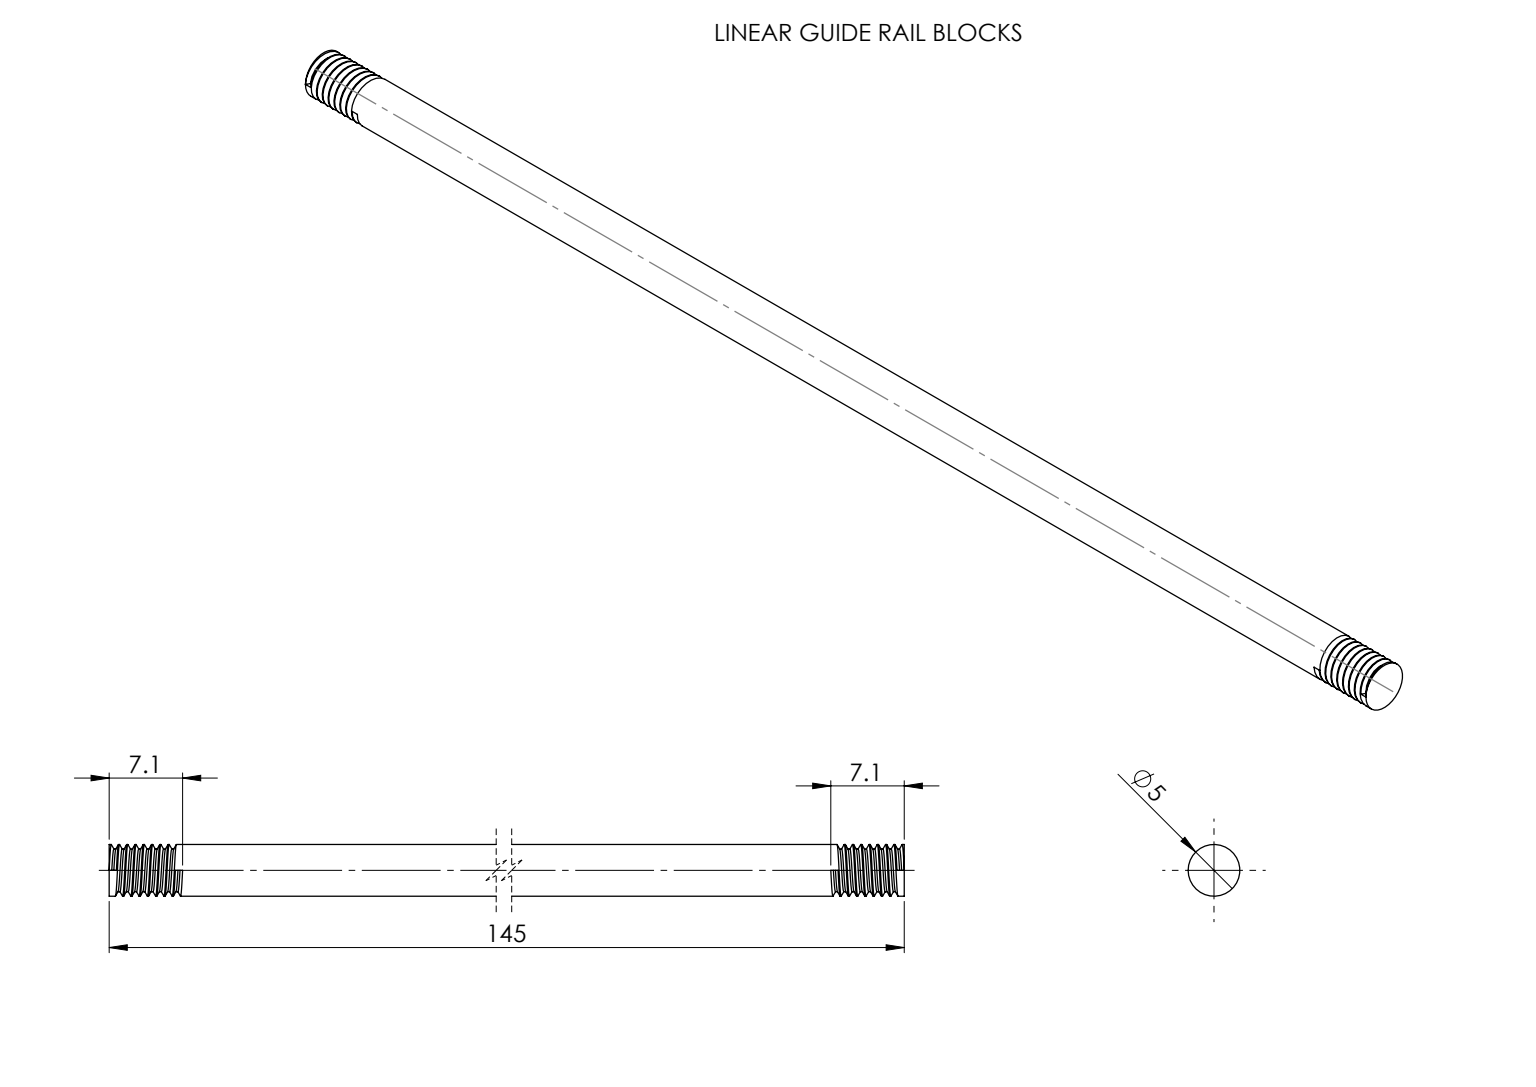
ISO-10303-21;
HEADER;
FILE_DESCRIPTION (('STEP AP214'),
    '1' );
FILE_NAME ('Linear Guide Rail Blocks.step',
    '2026-10-08T13:46:47',
    ( '' ),
    ( '' ),
    'SwSTEP 2.0',
    'SolidWorks 2026',
    '' );
FILE_SCHEMA (( 'AUTOMOTIVE_DESIGN' ));
ENDSEC;

DATA;
#7=AXIS2_PLACEMENT_3D ( 'NONE', #19593, #12332, #12571 ) ;
#8=CARTESIAN_POINT ( 'NONE',  ( -67.64999999999999147, 11.03553390593273598, 17.50000000000000355 ) ) ;
#17=CARTESIAN_POINT ( 'NONE',  ( 65.80000000218494449, 9.999999999999998224, 12.49999999999999289 ) ) ;
#19=CARTESIAN_POINT ( 'NONE',  ( -69.15000000109247935, 8.538419263543524096, 13.53841926354352054 ) ) ;
#22=CARTESIAN_POINT ( 'NONE',  ( -68.25000000109247367, 7.933012699999995476, 14.99999999999999645 ) ) ;
#32=CARTESIAN_POINT ( 'NONE',  ( -70.40000000109250777, 10.85617417291294551, 17.06698729999999742 ) ) ;
#33=CARTESIAN_POINT ( 'NONE',  ( -70.80000000109245661, 7.933012699999995476, 15.85617417291294196 ) ) ;
#43=CARTESIAN_POINT ( 'NONE',  ( 70.34999999999999432, 7.499999999999996447, 13.96446609406725514 ) ) ;
#48=EDGE_CURVE ( 'NONE', #4600, #14452, #12227, .T. ) ;
#57=( BOUNDED_CURVE ( )  B_SPLINE_CURVE ( 2, ( #2610, #2843, #8385, #9828, #929, #6582, #8267, #22849, #6463, #6101, #17122, #17483, #13433, #15701, #13784, #9954, #4303, #22975, #13896, #11639, #18906, #22618, #13542, #6222, #20810, #11753, #17248, #20493, #4334, #741, #505, #18828, #9508, #20729, #17161, #8185, #2415, #386, #851, #13111, #22409, #7826, #15148, #8076, #2169, #17043, #22169, #15387, #5783, #17285, #13469, #19061, #2652, #18588, #20845, #4223, #7945, #20371, #3977, #22286, #6018, #15031, #9746, #619, #18944, #15264, #9995, #7717, #11673, #4452, #2527, #5903, #11314, #13228, #4096, #9867, #13575, #16805, #11436, #18711, #22651, #22534, #2301, #9636, #6257, #16927, #11789, #11559, #13345, #20613, #6145, #10351, #23232, #4923, #21079, #10224, #15739, #2878, #3239, #19639, #8539, #1312, #13695, #13823, #19181, #20955, #6378, #23115, #17398, #12136, #14038, #23010, #4688, #12260, #8652, #1083, #8426, #10464, #2766, #17640, #1430, #6500, #17858, #21428, #22767, #13933, #19527, #15950, #1200 ),
 .UNSPECIFIED., .F., .F. ) 
 B_SPLINE_CURVE_WITH_KNOTS ( ( 3, 2, 2, 2, 2, 2, 2, 2, 2, 2, 2, 2, 2, 2, 2, 2, 2, 2, 2, 2, 2, 2, 2, 2, 2, 2, 2, 2, 2, 2, 2, 2, 2, 2, 2, 2, 2, 2, 2, 2, 2, 2, 2, 2, 2, 2, 2, 2, 2, 2, 2, 2, 2, 2, 2, 2, 2, 2, 2, 2, 2, 2, 2, 2, 3 ),
 ( 0.000000000000000000, 0.01562500000000000000, 0.03125000000000000000, 0.04687500000000000000, 0.06250000000000000000, 0.07812500000000000000, 0.09375000000000000000, 0.1093750000000000000, 0.1250000000000000000, 0.1406250000000000000, 0.1562500000000000000, 0.1718750000000000000, 0.1875000000000000000, 0.2031250000000000000, 0.2187500000000000000, 0.2343750000000000000, 0.2500000000000000000, 0.2656250000000000000, 0.2812500000000000000, 0.2968750000000000000, 0.3125000000000000000, 0.3281250000000000000, 0.3437500000000000000, 0.3593750000000000000, 0.3750000000000000000, 0.3906250000000000000, 0.4062500000000000000, 0.4218750000000000000, 0.4375000000000000000, 0.4531250000000000000, 0.4687500000000000000, 0.4843750000000000000, 0.5000000000000000000, 0.5156250000000000000, 0.5312500000000000000, 0.5468750000000000000, 0.5625000000000000000, 0.5781250000000000000, 0.5937500000000000000, 0.6093750000000000000, 0.6250000000000000000, 0.6406250000000000000, 0.6562500000000000000, 0.6718750000000000000, 0.6875000000000000000, 0.7031250000000000000, 0.7187500000000000000, 0.7343750000000000000, 0.7500000000000000000, 0.7656250000000000000, 0.7812500000000000000, 0.7968750000000000000, 0.8125000000000000000, 0.8281250000000000000, 0.8437500000000000000, 0.8593750000000000000, 0.8750000000000000000, 0.8906250000000000000, 0.9062500000000000000, 0.9218750000000000000, 0.9375000000000000000, 0.9531250000000000000, 0.9687500000000000000, 0.9843750000000000000, 1.000000000000000000 ),
 .UNSPECIFIED. ) 
 CURVE ( )  GEOMETRIC_REPRESENTATION_ITEM ( )  RATIONAL_B_SPLINE_CURVE ( ( 1.000000000000000000, 0.9238795325112867385, 1.000000000000000000, 0.9238795325112867385, 1.000000000000000000, 0.9238795325112867385, 1.000000000000000000, 0.9238795325112867385, 1.000000000000000000, 0.9238795325112867385, 1.000000000000000000, 0.9238795325112867385, 1.000000000000000000, 0.9238795325112867385, 1.000000000000000000, 0.9238795325112867385, 1.000000000000000000, 0.9238795325112867385, 1.000000000000000000, 0.9238795325112867385, 1.000000000000000000, 0.9238795325112867385, 1.000000000000000000, 0.9238795325112867385, 1.000000000000000000, 0.9238795325112867385, 1.000000000000000000, 0.9238795325112867385, 1.000000000000000000, 0.9238795325112867385, 1.000000000000000000, 0.9238795325112867385, 1.000000000000000000, 0.9238795325112867385, 1.000000000000000000, 0.9238795325112867385, 1.000000000000000000, 0.9238795325112867385, 1.000000000000000000, 0.9238795325112867385, 1.000000000000000000, 0.9238795325112867385, 1.000000000000000000, 0.9238795325112867385, 1.000000000000000000, 0.9238795325112867385, 1.000000000000000000, 0.9238795325112867385, 1.000000000000000000, 0.9238795325112867385, 1.000000000000000000, 0.9238795325112867385, 1.000000000000000000, 0.9238795325112867385, 1.000000000000000000, 0.9238795325112867385, 1.000000000000000000, 0.9238795325112867385, 1.000000000000000000, 0.9238795325112867385, 1.000000000000000000, 0.9238795325112867385, 1.000000000000000000, 0.9238795325112867385, 1.000000000000000000, 0.9238795325112867385, 1.000000000000000000, 0.9238795325112867385, 1.000000000000000000, 0.9238795325112867385, 1.000000000000000000, 0.9238795325112867385, 1.000000000000000000, 0.9238795325112867385, 1.000000000000000000, 0.9238795325112867385, 1.000000000000000000, 0.9238795325112867385, 1.000000000000000000, 0.9238795325112867385, 1.000000000000000000, 0.9238795325112867385, 1.000000000000000000, 0.9238795325112867385, 1.000000000000000000, 0.9238795325112867385, 1.000000000000000000, 0.9238795325112867385, 1.000000000000000000, 0.9238795325112867385, 1.000000000000000000, 0.9238795325112867385, 1.000000000000000000, 0.9238795325112867385, 1.000000000000000000, 0.9238795325112867385, 1.000000000000000000, 0.9238795325112867385, 1.000000000000000000, 0.9238795325112867385, 1.000000000000000000, 0.9238795325112867385, 1.000000000000000000, 0.9238795325112867385, 1.000000000000000000, 0.9238795325112867385, 1.000000000000000000, 0.9238795325112867385, 1.000000000000000000, 0.9238795325112867385, 1.000000000000000000, 0.9238795325112867385, 1.000000000000000000, 0.9238795325112867385, 1.000000000000000000, 0.9238795325112867385, 1.000000000000000000, 0.9238795325112867385, 1.000000000000000000, 0.9238795325112867385, 1.000000000000000000, 0.9238795325112867385, 1.000000000000000000, 0.9238795325112867385, 1.000000000000000000, 0.9238795325112867385, 1.000000000000000000, 0.9238795325112867385, 1.000000000000000000 ) ) 
 REPRESENTATION_ITEM ( '' )  );
#59=CARTESIAN_POINT ( 'NONE',  ( 68.14999999999999147, 11.03553390593273598, 12.49999999999999289 ) ) ;
#68=ORIENTED_EDGE ( 'NONE', *, *, #3329, .T. ) ;
#71=CARTESIAN_POINT ( 'NONE',  ( -72.37500000054622262, 9.999999999999998224, 17.28349365000000049 ) ) ;
#81=CARTESIAN_POINT ( 'NONE',  ( 66.15000000218495302, 11.03553390593273598, 17.50000000000000355 ) ) ;
#93=CARTESIAN_POINT ( 'NONE',  ( 72.25000000000000000, 12.50000000000000000, 13.96446609406725692 ) ) ;
#94=LINE ( 'NONE', #22476, #8071 ) ;
#96=DIRECTION ( 'NONE',  ( -1.000000000000000000, -0.000000000000000000, -0.000000000000000000 ) ) ;
#99=( NAMED_UNIT ( * ) PLANE_ANGLE_UNIT ( ) SI_UNIT ( $, .RADIAN. ) );
#105=CARTESIAN_POINT ( 'NONE',  ( 69.74999999999998579, 11.03553390593276262, 12.50000000000001776 ) ) ;
#107=CARTESIAN_POINT ( 'NONE',  ( -65.40000000218495302, 9.999999999999998224, 17.49999999999999645 ) ) ;
#116=CARTESIAN_POINT ( 'NONE',  ( -66.74999999999998579, 12.50000000000000000, 16.03553390593273420 ) ) ;
#117=AXIS2_PLACEMENT_3D ( 'NONE', #18833, #4695, #4456 ) ;
#118=CARTESIAN_POINT ( 'NONE',  ( 66.45000000218495018, 7.499999999999996447, 13.96446609406725514 ) ) ;
#120=CARTESIAN_POINT ( 'NONE',  ( 65.80000000109247082, 7.933012699999995476, 15.85617417291294196 ) ) ;
#127=PRODUCT ( 'Linear Guide Rail Blocks', 'Linear Guide Rail Blocks', '', ( #7707 ) ) ;
#130=CARTESIAN_POINT ( 'NONE',  ( -70.65000000109247935, 7.933012699999995476, 14.99999999999999645 ) ) ;
#133=CARTESIAN_POINT ( 'NONE',  ( -69.95000000109247651, 8.538419263543522320, 16.46158073645647235 ) ) ;
#141=CARTESIAN_POINT ( 'NONE',  ( -70.30000000109248504, 12.06698730000000275, 15.85617417291294196 ) ) ;
#144=CARTESIAN_POINT ( 'NONE',  ( -68.90000000109246514, 12.06698730000000275, 15.85617417291294196 ) ) ;
#170=CARTESIAN_POINT ( 'NONE',  ( 67.99999999999998579, 8.232233047033629347, 13.23223304703362402 ) ) ;
#172=DIRECTION ( 'NONE',  ( 0.000000000000000000, 0.000000000000000000, 1.000000000000000000 ) ) ;
#181=CARTESIAN_POINT ( 'NONE',  ( 68.60000000218495586, 9.999999999999998224, 17.49999999999999645 ) ) ;
#191=( BOUNDED_CURVE ( )  B_SPLINE_CURVE ( 2, ( #20921, #4538, #19693, #10520, #10408, #17688, #1250, #8589, #23173 ),
 .UNSPECIFIED., .F., .F. ) 
 B_SPLINE_CURVE_WITH_KNOTS ( ( 3, 2, 2, 2, 3 ),
 ( 0.3125000000000002776, 0.3281250000000001665, 0.3437500000000001110, 0.3593750000000000000, 0.3749999999999998890 ),
 .UNSPECIFIED. ) 
 CURVE ( )  GEOMETRIC_REPRESENTATION_ITEM ( )  RATIONAL_B_SPLINE_CURVE ( ( 0.9999999999999986677, 0.9238795325112880708, 1.000000000000000000, 0.9238795325112867385, 1.000000000000000000, 0.9238795325112867385, 1.000000000000000000, 0.9238795325112872936, 0.9999999999999994449 ) ) 
 REPRESENTATION_ITEM ( '' )  );
#198=CARTESIAN_POINT ( 'NONE',  ( 70.50000000109247367, 9.143825827087049163, 17.06698729999999742 ) ) ;
#200=CARTESIAN_POINT ( 'NONE',  ( 70.75000000109247367, 8.538419263543522320, 16.46158073645647235 ) ) ;
#206=DIRECTION ( 'NONE',  ( -1.000000000000000000, -0.000000000000000000, -0.000000000000000000 ) ) ;
#218=CARTESIAN_POINT ( 'NONE',  ( 70.54999999999999716, 11.03553390593272177, 12.49999999999998046 ) ) ;
#229=CARTESIAN_POINT ( 'NONE',  ( 71.25000000109247367, 12.06698730000000097, 14.99999999999999645 ) ) ;
#230=ORIENTED_EDGE ( 'NONE', *, *, #2307, .F. ) ;
#231=CARTESIAN_POINT ( 'NONE',  ( -68.54999999999999716, 8.964466094067258695, 17.50000000000000355 ) ) ;
#233=CARTESIAN_POINT ( 'NONE',  ( 66.95000000109246230, 11.46158073645647235, 13.53841926354352232 ) ) ;
#242=CARTESIAN_POINT ( 'NONE',  ( -69.65000000109247935, 9.999999999999998224, 17.06698730000000097 ) ) ;
#245=CARTESIAN_POINT ( 'NONE',  ( -71.80000000109245661, 9.143825827087050939, 12.93301269999999370 ) ) ;
#254=CARTESIAN_POINT ( 'NONE',  ( -70.50000000109247367, 9.143825827087049163, 17.06698729999999742 ) ) ;
#256=CARTESIAN_POINT ( 'NONE',  ( -69.15000000109246514, 8.538419263543522320, 16.46158073645647235 ) ) ;
#258=PLANE ( 'NONE',  #11121 ) ;
#260=CARTESIAN_POINT ( 'NONE',  ( -71.70000000000000284, 9.999999999999998224, 17.49999999999999645 ) ) ;
#283=ADVANCED_FACE ( 'NONE', ( #1848 ), #11347, .T. ) ;
#289=CARTESIAN_POINT ( 'NONE',  ( 69.14999999999999147, 12.50000000000000000, 16.03553390593273420 ) ) ;
#318=CARTESIAN_POINT ( 'NONE',  ( 70.70000000109247651, 7.933012699999995476, 14.14382582708705094 ) ) ;
#319=CARTESIAN_POINT ( 'NONE',  ( 66.49999999999998579, 9.999999999999998224, 12.49999999999999289 ) ) ;
#320=CARTESIAN_POINT ( 'NONE',  ( 71.55000000109245661, 8.538419263543522320, 16.46158073645647235 ) ) ;
#333=CARTESIAN_POINT ( 'NONE',  ( -70.20000000218495018, 9.999999999999998224, 17.49999999999999645 ) ) ;
#337=ORIENTED_EDGE ( 'NONE', *, *, #22086, .T. ) ;
#354=CARTESIAN_POINT ( 'NONE',  ( 69.75000000109245946, 11.46158073645647235, 16.46158073645647235 ) ) ;
#360=CARTESIAN_POINT ( 'NONE',  ( 65.75000000109247367, 8.538419263543522320, 16.46158073645647235 ) ) ;
#366=CARTESIAN_POINT ( 'NONE',  ( -71.30000000218494449, 8.232233047033629347, 13.23223304703362402 ) ) ;
#370=CARTESIAN_POINT ( 'NONE',  ( -68.10000000109248219, 9.143825827087049163, 17.06698730000000097 ) ) ;
#373=CARTESIAN_POINT ( 'NONE',  ( -71.90000000109246514, 10.85617417291294551, 12.93301269999999370 ) ) ;
#384=CARTESIAN_POINT ( 'NONE',  ( -67.50000000109247367, 7.933012699999995476, 14.14382582708705094 ) ) ;
#386=CARTESIAN_POINT ( 'NONE',  ( 70.20000000109246230, 12.06698729999999919, 14.14382582708705094 ) ) ;
#388=CARTESIAN_POINT ( 'NONE',  ( -67.75000000109245946, 8.538419263543524096, 13.53841926354352054 ) ) ;
#399=ORIENTED_EDGE ( 'NONE', *, *, #10605, .F. ) ;
#400=CARTESIAN_POINT ( 'NONE',  ( 70.39999999999999147, 8.232233047033629347, 13.23223304703362402 ) ) ;
#411=DIRECTION ( 'NONE',  ( 0.000000000000000000, 0.000000000000000000, -1.000000000000000000 ) ) ;
#413=CARTESIAN_POINT ( 'NONE',  ( -70.80000000218494449, 12.50000000000000000, 14.99999999999999645 ) ) ;
#417=CARTESIAN_POINT ( 'NONE',  ( 69.49999999999998579, 7.499999999999996447, 14.99999999999999645 ) ) ;
#426=CARTESIAN_POINT ( 'NONE',  ( -71.30000000109247082, 12.06698729999999919, 15.85617417291294196 ) ) ;
#431=CARTESIAN_POINT ( 'NONE',  ( -71.35000000109246798, 8.538419263543522320, 16.46158073645647235 ) ) ;
#433=VERTEX_POINT ( 'NONE', #17433 ) ;
#442=CARTESIAN_POINT ( 'NONE',  ( 71.20000000109246230, 10.85617417291294551, 17.06698729999999742 ) ) ;
#444=CARTESIAN_POINT ( 'NONE',  ( 70.85000000109246798, 7.933012699999995476, 14.99999999999999645 ) ) ;
#445=EDGE_CURVE ( 'NONE', #15027, #12453, #14670, .T. ) ;
#448=CARTESIAN_POINT ( 'NONE',  ( -69.70000000000000284, 9.999999999999998224, 12.49999999999999289 ) ) ;
#456=CARTESIAN_POINT ( 'NONE',  ( -67.00000000109245946, 9.143825827087052716, 12.93301269999999192 ) ) ;
#467=ORIENTED_EDGE ( 'NONE', *, *, #9823, .T. ) ;
#468=CARTESIAN_POINT ( 'NONE',  ( 72.50000000000000000, 9.999999999999998224, 14.99999999999999645 ) ) ;
#474=( NAMED_UNIT ( * ) PLANE_ANGLE_UNIT ( ) SI_UNIT ( $, .RADIAN. ) );
#475=CARTESIAN_POINT ( 'NONE',  ( 70.65000000109246514, 9.999999999999998224, 17.06698730000000097 ) ) ;
#481=CARTESIAN_POINT ( 'NONE',  ( 71.55000000109245661, 8.538419263543522320, 16.46158073645647235 ) ) ;
#489=DIRECTION ( 'NONE',  ( -1.000000000000000000, -0.000000000000000000, -0.000000000000000000 ) ) ;
#494=CARTESIAN_POINT ( 'NONE',  ( -71.70000000109247651, 7.933012699999995476, 14.14382582708705094 ) ) ;
#503=CARTESIAN_POINT ( 'NONE',  ( -66.95000000109246230, 11.46158073645647235, 13.53841926354352232 ) ) ;
#505=CARTESIAN_POINT ( 'NONE',  ( 70.55000000109247082, 8.538419263543522320, 16.46158073645647235 ) ) ;
#506=CARTESIAN_POINT ( 'NONE',  ( -67.35000000109246798, 11.46158073645647235, 16.46158073645647235 ) ) ;
#515=CARTESIAN_POINT ( 'NONE',  ( 72.09999999999999432, 9.999999999999998224, 12.49999999999999289 ) ) ;
#516=EDGE_LOOP ( 'NONE', ( #68, #21518, #3055, #2681, #12780, #20192, #1158, #14031, #18308, #16919, #16791, #2387, #4988, #13331, #13453, #17105, #21865, #10269, #6716 ) ) ;
#528=CARTESIAN_POINT ( 'NONE',  ( -69.50000000218494733, 8.232233047033627571, 16.76776695296636532 ) ) ;
#531=CARTESIAN_POINT ( 'NONE',  ( 68.34999999999999432, 12.50000000000000000, 16.03553390593273420 ) ) ;
#541=( BOUNDED_CURVE ( )  B_SPLINE_CURVE ( 2, ( #16400, #7064, #18073, #8877, #7426, #5378, #16170, #18188, #11021 ),
 .UNSPECIFIED., .F., .F. ) 
 B_SPLINE_CURVE_WITH_KNOTS ( ( 3, 2, 2, 2, 3 ),
 ( 0.4999999999999991118, 0.5156249999999995559, 0.5312500000000000000, 0.5468750000000004441, 0.5625000000000008882 ),
 .UNSPECIFIED. ) 
 CURVE ( )  GEOMETRIC_REPRESENTATION_ITEM ( )  RATIONAL_B_SPLINE_CURVE ( ( 1.000000000000004219, 0.9238795325112824086, 1.000000000000000000, 0.9238795325112867385, 1.000000000000000000, 0.9238795325112867385, 1.000000000000000000, 0.9238795325112824086, 1.000000000000004219 ) ) 
 REPRESENTATION_ITEM ( '' )  );
#543=CARTESIAN_POINT ( 'NONE',  ( -70.85000000109246798, 9.999999999999998224, 12.93301269999999192 ) ) ;
#552=CARTESIAN_POINT ( 'NONE',  ( 66.35000000218495586, 7.499999999999995559, 16.03553390593273420 ) ) ;
#555=CARTESIAN_POINT ( 'NONE',  ( 71.30000000109247082, 12.06698730000000275, 15.85617417291294196 ) ) ;
#588=CARTESIAN_POINT ( 'NONE',  ( 69.45000000109247651, 9.999999999999998224, 12.93301269999999192 ) ) ;
#593=CARTESIAN_POINT ( 'NONE',  ( 72.15000000109246514, 11.46158073645647235, 16.46158073645647235 ) ) ;
#603=CARTESIAN_POINT ( 'NONE',  ( -66.70000000109246230, 7.933012699999995476, 14.14382582708705094 ) ) ;
#606=CARTESIAN_POINT ( 'NONE',  ( -67.85000000109246798, 9.999999999999998224, 12.93301269999999192 ) ) ;
#618=CARTESIAN_POINT ( 'NONE',  ( -67.35000000109248219, 8.538419263543522320, 16.46158073645647235 ) ) ;
#619=CARTESIAN_POINT ( 'NONE',  ( 68.90000000109247935, 9.143825827087049163, 17.06698730000000097 ) ) ;
#620=CARTESIAN_POINT ( 'NONE',  ( -72.29999999999998295, 12.50000000000000000, 14.99999999999999645 ) ) ;
#635=LINE ( 'NONE', #22428, #20559 ) ;
#641=CARTESIAN_POINT ( 'NONE',  ( -71.65000000218496723, 12.50000000000000000, 16.03553390593273420 ) ) ;
#646=CARTESIAN_POINT ( 'NONE',  ( 70.45000000109247651, 9.999999999999998224, 17.06698730000000097 ) ) ;
#647=VECTOR ( 'NONE', #5180, 999.9999999999997726 ) ;
#653=CARTESIAN_POINT ( 'NONE',  ( -71.40000000109246514, 10.85617417291294551, 17.06698730000000097 ) ) ;
#658=CARTESIAN_POINT ( 'NONE',  ( -71.10000000109246798, 12.06698730000000275, 15.85617417291294196 ) ) ;
#667=CARTESIAN_POINT ( 'NONE',  ( 68.15000000109247935, 8.538419263543522320, 16.46158073645647235 ) ) ;
#668=CARTESIAN_POINT ( 'NONE',  ( 69.50000000109247367, 10.85617417291294551, 12.93301269999999370 ) ) ;
#683=VERTEX_POINT ( 'NONE', #3814 ) ;
#686=CARTESIAN_POINT ( 'NONE',  ( -70.54999999999999716, 11.03553390593272177, 12.49999999999998046 ) ) ;
#687=ADVANCED_FACE ( 'NONE', ( #12941 ), #1773, .T. ) ;
#691=CARTESIAN_POINT ( 'NONE',  ( -72.50000000000000000, 9.999999999999998224, 12.49999999999999289 ) ) ;
#704=CARTESIAN_POINT ( 'NONE',  ( 71.50000000109247367, 9.143825827087049163, 17.06698730000000097 ) ) ;
#711=CARTESIAN_POINT ( 'NONE',  ( 70.70000000109247651, 9.143825827087049163, 17.06698729999999742 ) ) ;
#728=CARTESIAN_POINT ( 'NONE',  ( -67.80000000109247082, 9.143825827087050939, 12.93301269999999370 ) ) ;
#735=VERTEX_POINT ( 'NONE', #17959 ) ;
#740=CARTESIAN_POINT ( 'NONE',  ( -68.40000000109249356, 9.143825827087050939, 12.93301269999999370 ) ) ;
#741=CARTESIAN_POINT ( 'NONE',  ( 70.60000000109246798, 7.933012699999995476, 15.85617417291294196 ) ) ;
#742=CARTESIAN_POINT ( 'NONE',  ( -65.90000000109246514, 9.143825827087049163, 17.06698729999999742 ) ) ;
#748=CARTESIAN_POINT ( 'NONE',  ( 72.50000000000000000, 9.999999999999998224, 17.49999999999999645 ) ) ;
#751=CARTESIAN_POINT ( 'NONE',  ( 72.05000000109247082, 9.999999999999998224, 17.06698730000000097 ) ) ;
#768=CARTESIAN_POINT ( 'NONE',  ( -69.20000000218495018, 12.50000000000000000, 14.99999999999999645 ) ) ;
#773=CARTESIAN_POINT ( 'NONE',  ( -71.29999999999998295, 9.999999999999998224, 12.49999999999999289 ) ) ;
#775=CARTESIAN_POINT ( 'NONE',  ( 70.40000000109250777, 10.85617417291294551, 17.06698729999999742 ) ) ;
#776=CARTESIAN_POINT ( 'NONE',  ( 70.70000000218495018, 11.76776695296636888, 13.23223304703362579 ) ) ;
#783=CARTESIAN_POINT ( 'NONE',  ( -68.40000000109246514, 7.933012699999995476, 15.85617417291294196 ) ) ;
#790=CARTESIAN_POINT ( 'NONE',  ( -69.45000000109247651, 12.06698730000000097, 14.99999999999999645 ) ) ;
#793=CARTESIAN_POINT ( 'NONE',  ( 72.50000000000000000, 9.999999999999998224, 12.49999999999999289 ) ) ;
#798=CARTESIAN_POINT ( 'NONE',  ( 68.70000000109246230, 12.06698730000000275, 15.85617417291294196 ) ) ;
#799=CARTESIAN_POINT ( 'NONE',  ( 68.70000000109246230, 10.85617417291294551, 12.93301269999999370 ) ) ;
#807=ORIENTED_EDGE ( 'NONE', *, *, #21186, .F. ) ;
#815=CARTESIAN_POINT ( 'NONE',  ( 71.20000000218495018, 7.499999999999996447, 14.99999999999999645 ) ) ;
#822=CARTESIAN_POINT ( 'NONE',  ( 71.45000000218495018, 11.03553390593273598, 12.49999999999999289 ) ) ;
#826=CARTESIAN_POINT ( 'NONE',  ( 68.30000000109247082, 9.143825827087049163, 17.06698730000000097 ) ) ;
#829=CARTESIAN_POINT ( 'NONE',  ( 70.65000000109246514, 9.999999999999998224, 17.06698730000000097 ) ) ;
#838=CARTESIAN_POINT ( 'NONE',  ( -67.10000000109248219, 12.06698729999999919, 15.85617417291294196 ) ) ;
#840=CARTESIAN_POINT ( 'NONE',  ( -68.10000000109245377, 12.06698730000000275, 15.85617417291294196 ) ) ;
#849=CARTESIAN_POINT ( 'NONE',  ( -68.60000000109248219, 12.06698730000000275, 14.14382582708705094 ) ) ;
#851=CARTESIAN_POINT ( 'NONE',  ( 70.15000000109247935, 11.46158073645647235, 13.53841926354352232 ) ) ;
#853=CARTESIAN_POINT ( 'NONE',  ( -67.95000000109247651, 11.46158073645647235, 13.53841926354352232 ) ) ;
#858=LINE ( 'NONE', #4584, #16612 ) ;
#876=CARTESIAN_POINT ( 'NONE',  ( -71.70000000218495018, 11.76776695296636888, 16.76776695296636532 ) ) ;
#881=CARTESIAN_POINT ( 'NONE',  ( 66.59999999999999432, 11.76776695296636888, 13.23223304703362579 ) ) ;
#882=CARTESIAN_POINT ( 'NONE',  ( 70.75000000109247367, 8.538419263543524096, 13.53841926354352054 ) ) ;
#888=CARTESIAN_POINT ( 'NONE',  ( 67.35000000000000853, 11.03553390593276973, 12.50000000000002665 ) ) ;
#889=CARTESIAN_POINT ( 'NONE',  ( -69.40000000109246514, 9.143825827087052716, 12.93301269999999192 ) ) ;
#905=CARTESIAN_POINT ( 'NONE',  ( 67.75000000109247367, 11.46158073645647235, 13.53841926354352232 ) ) ;
#906=EDGE_CURVE ( 'NONE', #14683, #16067, #1009, .T. ) ;
#907=CARTESIAN_POINT ( 'NONE',  ( 68.45000000109247651, 7.933012699999995476, 14.99999999999999645 ) ) ;
#914=DIRECTION ( 'NONE',  ( -1.000000000000000000, -0.000000000000000000, -0.000000000000000000 ) ) ;
#921=CARTESIAN_POINT ( 'NONE',  ( 69.30000000218494449, 11.76776695296636888, 16.76776695296636532 ) ) ;
#922=CARTESIAN_POINT ( 'NONE',  ( 72.50000000000000000, 9.999999999999998224, 12.49999999999999289 ) ) ;
#923=PRODUCT_DEFINITION_CONTEXT ( 'detailed design', #3030, 'design' ) ;
#928=ORIENTED_EDGE ( 'NONE', *, *, #4298, .F. ) ;
#929=CARTESIAN_POINT ( 'NONE',  ( 71.85000000109246798, 12.06698730000000097, 14.99999999999999645 ) ) ;
#932=CARTESIAN_POINT ( 'NONE',  ( 70.70000000218495018, 11.76776695296636888, 13.23223304703362579 ) ) ;
#935=CARTESIAN_POINT ( 'NONE',  ( 68.10000000109246798, 12.06698729999999919, 15.85617417291294196 ) ) ;
#939=CARTESIAN_POINT ( 'NONE',  ( 70.30000000109248504, 10.85617417291294551, 12.93301269999999370 ) ) ;
#945=LINE ( 'NONE', #1062, #11167 ) ;
#955=CARTESIAN_POINT ( 'NONE',  ( -69.20000000109246230, 7.933012699999995476, 15.85617417291294196 ) ) ;
#967=CARTESIAN_POINT ( 'NONE',  ( -70.95000000000000284, 8.964466094067258695, 17.50000000000000355 ) ) ;
#980=CARTESIAN_POINT ( 'NONE',  ( -71.40000000218495302, 9.999999999999998224, 12.49999999999999289 ) ) ;
#985=EDGE_CURVE ( 'NONE', #683, #21124, #19386, .T. ) ;
#994=CARTESIAN_POINT ( 'NONE',  ( -67.35000000218495586, 8.964466094067258695, 12.49999999999999289 ) ) ;
#997=CARTESIAN_POINT ( 'NONE',  ( 66.40000000000000568, 8.232233047033629347, 13.23223304703362402 ) ) ;
#1000=CARTESIAN_POINT ( 'NONE',  ( 71.20000000109246230, 10.85617417291294551, 17.06698729999999742 ) ) ;
#1008=CARTESIAN_POINT ( 'NONE',  ( -67.55000000109247082, 8.538419263543522320, 16.46158073645647235 ) ) ;
#1009=LINE ( 'NONE', #6420, #5098 ) ;
#1023=CARTESIAN_POINT ( 'NONE',  ( 68.30000000109247082, 7.933012699999995476, 14.14382582708705094 ) ) ;
#1025=CARTESIAN_POINT ( 'NONE',  ( 68.15000000109246514, 11.46158073645647235, 16.46158073645647235 ) ) ;
#1047=CARTESIAN_POINT ( 'NONE',  ( 71.70000000000000284, 9.999999999999998224, 17.49999999999999645 ) ) ;
#1050=CARTESIAN_POINT ( 'NONE',  ( 69.75000000218496155, 8.964466094067258695, 12.49999999999999289 ) ) ;
#1054=CARTESIAN_POINT ( 'NONE',  ( 68.40000000109246514, 7.933012699999995476, 15.85617417291294196 ) ) ;
#1057=LINE ( 'NONE', #8392, #23303 ) ;
#1059=CARTESIAN_POINT ( 'NONE',  ( 69.60000000109248219, 12.06698730000000275, 14.14382582708705094 ) ) ;
#1062=CARTESIAN_POINT ( 'NONE',  ( 72.50000000000000000, 9.999999999999998224, 12.49999999999999289 ) ) ;
#1073=CARTESIAN_POINT ( 'NONE',  ( -68.00000000109245946, 12.06698730000000275, 14.14382582708705094 ) ) ;
#1083=CARTESIAN_POINT ( 'NONE',  ( 66.30000000109247082, 12.06698729999999919, 15.85617417291294196 ) ) ;
#1084=CARTESIAN_POINT ( 'NONE',  ( -70.09999999999999432, 9.999999999999998224, 17.49999999999999645 ) ) ;
#1095=CARTESIAN_POINT ( 'NONE',  ( -71.00000000109248788, 12.06698729999999919, 14.14382582708705094 ) ) ;
#1109=CARTESIAN_POINT ( 'NONE',  ( -66.35000000218495586, 7.499999999999995559, 16.03553390593273420 ) ) ;
#1117=CARTESIAN_POINT ( 'NONE',  ( 68.50000000109247367, 10.85617417291294551, 12.93301269999999370 ) ) ;
#1119=CARTESIAN_POINT ( 'NONE',  ( 70.80000000218494449, 12.50000000000000000, 14.99999999999999645 ) ) ;
#1123=CARTESIAN_POINT ( 'NONE',  ( -69.60000000109246798, 12.06698729999999919, 14.14382582708705094 ) ) ;
#1125=CARTESIAN_POINT ( 'NONE',  ( -69.95000000218493597, 12.50000000000000000, 13.96446609406725692 ) ) ;
#1141=CARTESIAN_POINT ( 'NONE',  ( 66.75000000109247367, 8.538419263543524096, 13.53841926354352054 ) ) ;
#1144=CARTESIAN_POINT ( 'NONE',  ( 68.60000000109246798, 9.143825827087050939, 12.93301269999999370 ) ) ;
#1157=VECTOR ( 'NONE', #6497, 1000.000000000000000 ) ;
#1158=ORIENTED_EDGE ( 'NONE', *, *, #4205, .F. ) ;
#1160=CARTESIAN_POINT ( 'NONE',  ( 71.50000000109248788, 7.933012699999995476, 14.14382582708705094 ) ) ;
#1164=ORIENTED_EDGE ( 'NONE', *, *, #3803, .F. ) ;
#1169=CARTESIAN_POINT ( 'NONE',  ( 71.40000000218495302, 9.999999999999998224, 12.49999999999999289 ) ) ;
#1172=CARTESIAN_POINT ( 'NONE',  ( 67.65000000109247935, 7.933012699999995476, 14.99999999999999645 ) ) ;
#1188=CARTESIAN_POINT ( 'NONE',  ( -72.15000000000001990, 11.03553390593275374, 12.50000000000001243 ) ) ;
#1189=ORIENTED_EDGE ( 'NONE', *, *, #10837, .T. ) ;
#1200=CARTESIAN_POINT ( 'NONE',  ( 65.65000000109247935, 9.999999999999998224, 17.06698730000000097 ) ) ;
#1203=CARTESIAN_POINT ( 'NONE',  ( -69.05000000000002558, 12.50000000000000000, 13.96446609406725869 ) ) ;
#1207=CARTESIAN_POINT ( 'NONE',  ( -67.60000000218495586, 12.50000000000000000, 14.99999999999999645 ) ) ;
#1208=CARTESIAN_POINT ( 'NONE',  ( 72.50000000000000000, 9.999999999999998224, 14.99999999999999645 ) ) ;
#1212=CARTESIAN_POINT ( 'NONE',  ( -71.95000000109247651, 11.46158073645647235, 16.46158073645647235 ) ) ;
#1215=CARTESIAN_POINT ( 'NONE',  ( -70.25000000109247367, 12.06698730000000097, 14.99999999999999645 ) ) ;
#1224=CARTESIAN_POINT ( 'NONE',  ( -65.80000000218494449, 9.999999999999998224, 12.49999999999999289 ) ) ;
#1235=CARTESIAN_POINT ( 'NONE',  ( -67.60000000109246798, 7.933012699999995476, 15.85617417291294196 ) ) ;
#1244=ORIENTED_EDGE ( 'NONE', *, *, #22795, .F. ) ;
#1250=CARTESIAN_POINT ( 'NONE',  ( -69.50000000218494733, 8.232233047033627571, 16.76776695296636532 ) ) ;
#1253=CARTESIAN_POINT ( 'NONE',  ( 71.89999999999999147, 7.499999999999996447, 14.99999999999999645 ) ) ;
#1264=VERTEX_POINT ( 'NONE', #3404 ) ;
#1266=EDGE_CURVE ( 'NONE', #1264, #22517, #13759, .T. ) ;
#1267=CARTESIAN_POINT ( 'NONE',  ( 68.49999999999998579, 9.999999999999998224, 17.49999999999999645 ) ) ;
#1278=CARTESIAN_POINT ( 'NONE',  ( 67.95000000218495018, 7.499999999999995559, 16.03553390593273420 ) ) ;
#1282=CARTESIAN_POINT ( 'NONE',  ( 68.50000000109245946, 7.933012699999995476, 14.14382582708705094 ) ) ;
#1287=CARTESIAN_POINT ( 'NONE',  ( 67.05000000109247082, 9.999999999999998224, 12.93301269999999192 ) ) ;
#1294=EDGE_CURVE ( 'NONE', #4086, #4004, #9769, .T. ) ;
#1296=CARTESIAN_POINT ( 'NONE',  ( 66.74999999999998579, 12.50000000000000000, 16.03553390593273775 ) ) ;
#1301=( BOUNDED_CURVE ( )  B_SPLINE_CURVE ( 2, ( #8573, #11827, #14083, #4487, #6656, #23044, #12176, #888, #15541 ),
 .UNSPECIFIED., .F., .F. ) 
 B_SPLINE_CURVE_WITH_KNOTS ( ( 3, 2, 2, 2, 3 ),
 ( 0.7499999999999997780, 0.7656249999999996669, 0.7812499999999995559, 0.7968749999999994449, 0.8124999999999993339 ),
 .UNSPECIFIED. ) 
 CURVE ( )  GEOMETRIC_REPRESENTATION_ITEM ( )  RATIONAL_B_SPLINE_CURVE ( ( 1.000000000000001110, 0.9238795325112856283, 1.000000000000000000, 0.9238795325112867385, 1.000000000000000000, 0.9238795325112867385, 1.000000000000000000, 0.9238795325112899581, 0.9999999999999967804 ) ) 
 REPRESENTATION_ITEM ( '' )  );
#1311=CARTESIAN_POINT ( 'NONE',  ( -65.85000000109248219, 7.933012699999995476, 14.99999999999999645 ) ) ;
#1312=CARTESIAN_POINT ( 'NONE',  ( 67.00000000109247367, 12.06698729999999919, 14.14382582708705094 ) ) ;
#1315=CARTESIAN_POINT ( 'NONE',  ( -69.34999999999999432, 8.964466094067258695, 17.50000000000000355 ) ) ;
#1316=AXIS2_PLACEMENT_3D ( 'NONE', #8399, #23094, #6705 ) ;
#1329=CARTESIAN_POINT ( 'NONE',  ( -68.40000000109249356, 9.143825827087050939, 12.93301269999999370 ) ) ;
#1340=EDGE_LOOP ( 'NONE', ( #18060, #5958, #5413, #5040 ) ) ;
#1342=CARTESIAN_POINT ( 'NONE',  ( -68.65000000218496723, 8.964466094067258695, 17.50000000000000355 ) ) ;
#1345=CARTESIAN_POINT ( 'NONE',  ( -71.95000000109247651, 11.46158073645647235, 13.53841926354352232 ) ) ;
#1355=CARTESIAN_POINT ( 'NONE',  ( 70.40000000218495302, 7.499999999999996447, 14.99999999999999645 ) ) ;
#1363=LINE ( 'NONE', #18249, #21589 ) ;
#1371=CARTESIAN_POINT ( 'NONE',  ( 66.00000000109247367, 9.143825827087050939, 12.93301269999999370 ) ) ;
#1372=CARTESIAN_POINT ( 'NONE',  ( 71.70000000000000284, 9.999999999999998224, 17.49999999999999645 ) ) ;
#1373=CARTESIAN_POINT ( 'NONE',  ( -65.60000000218495586, 7.499999999999996447, 14.99999999999999645 ) ) ;
#1390=ORIENTED_EDGE ( 'NONE', *, *, #6277, .F. ) ;
#1392=CARTESIAN_POINT ( 'NONE',  ( 68.95000000218495018, 8.964466094067258695, 12.49999999999999289 ) ) ;
#1395=CARTESIAN_POINT ( 'NONE',  ( -68.79999999999999716, 8.232233047033629347, 13.23223304703362402 ) ) ;
#1402=CARTESIAN_POINT ( 'NONE',  ( 68.00000000109245946, 12.06698730000000275, 14.14382582708705094 ) ) ;
#1405=CARTESIAN_POINT ( 'NONE',  ( 72.50000000000000000, 9.999999999999998224, 14.99999999999999645 ) ) ;
#1411=CARTESIAN_POINT ( 'NONE',  ( 66.49999999999998579, 9.999999999999998224, 12.49999999999999289 ) ) ;
#1412=ORIENTED_EDGE ( 'NONE', *, *, #20233, .F. ) ;
#1417=CARTESIAN_POINT ( 'NONE',  ( -66.05000000218494449, 12.50000000000000000, 16.03553390593273775 ) ) ;
#1428=CARTESIAN_POINT ( 'NONE',  ( -65.70000000109249072, 9.143825827087049163, 17.06698729999999742 ) ) ;
#1430=CARTESIAN_POINT ( 'NONE',  ( 66.05000000109247082, 9.999999999999998224, 12.93301269999999192 ) ) ;
#1432=CARTESIAN_POINT ( 'NONE',  ( -71.84999999999999432, 7.499999999999995559, 16.03553390593273420 ) ) ;
#1440=CARTESIAN_POINT ( 'NONE',  ( 67.40000000218495302, 9.999999999999998224, 12.49999999999999289 ) ) ;
#1443=CARTESIAN_POINT ( 'NONE',  ( -66.60000000218495586, 9.999999999999998224, 12.49999999999999289 ) ) ;
#1445=ORIENTED_EDGE ( 'NONE', *, *, #21073, .F. ) ;
#1447=CARTESIAN_POINT ( 'NONE',  ( -71.20000000109246230, 10.85617417291294551, 17.06698730000000097 ) ) ;
#1450=CARTESIAN_POINT ( 'NONE',  ( -68.55000000109247082, 11.46158073645647235, 13.53841926354352232 ) ) ;
#1461=CARTESIAN_POINT ( 'NONE',  ( -68.00000000218494733, 7.499999999999996447, 14.99999999999999645 ) ) ;
#1468=EDGE_CURVE ( 'NONE', #20225, #9434, #3125, .T. ) ;
#1470=CARTESIAN_POINT ( 'NONE',  ( 67.20000000000000284, 8.232233047033629347, 13.23223304703362402 ) ) ;
#1489=( BOUNDED_CURVE ( )  B_SPLINE_CURVE ( 2, ( #9941, #22479, #9817, #5972, #17238, #4406, #20909, #686, #6333 ),
 .UNSPECIFIED., .F., .F. ) 
 B_SPLINE_CURVE_WITH_KNOTS ( ( 3, 2, 2, 2, 3 ),
 ( 0.2500000000000006661, 0.2656250000000005551, 0.2812500000000004441, 0.2968750000000003886, 0.3125000000000002776 ),
 .UNSPECIFIED. ) 
 CURVE ( )  GEOMETRIC_REPRESENTATION_ITEM ( )  RATIONAL_B_SPLINE_CURVE ( ( 0.9999999999999967804, 0.9238795325112899581, 1.000000000000000000, 0.9238795325112867385, 1.000000000000000000, 0.9238795325112867385, 1.000000000000000000, 0.9238795325112854062, 1.000000000000001332 ) ) 
 REPRESENTATION_ITEM ( '' )  );
#1493=ORIENTED_EDGE ( 'NONE', *, *, #3803, .T. ) ;
#1501=CARTESIAN_POINT ( 'NONE',  ( 71.00000000000000000, 8.232233047033627571, 16.76776695296636532 ) ) ;
#1525=CARTESIAN_POINT ( 'NONE',  ( 67.85000000218495586, 8.964466094067258695, 17.50000000000000355 ) ) ;
#1529=ORIENTED_EDGE ( 'NONE', *, *, #19125, .F. ) ;
#1533=CARTESIAN_POINT ( 'NONE',  ( 67.20000000109247651, 12.06698730000000275, 14.14382582708705094 ) ) ;
#1536=CARTESIAN_POINT ( 'NONE',  ( -68.05000000000001137, 8.964466094067256918, 12.49999999999999822 ) ) ;
#1559=CARTESIAN_POINT ( 'NONE',  ( -68.25000000000000000, 12.50000000000000000, 13.96446609406725869 ) ) ;
#1568=ORIENTED_EDGE ( 'NONE', *, *, #14803, .T. ) ;
#1570=CARTESIAN_POINT ( 'NONE',  ( -71.85000000109246798, 12.06698730000000097, 14.99999999999999645 ) ) ;
#1573=CARTESIAN_POINT ( 'NONE',  ( -66.90000000109246514, 10.85617417291294551, 12.93301269999999370 ) ) ;
#1584=CARTESIAN_POINT ( 'NONE',  ( -71.30000000109248504, 9.143825827087049163, 17.06698729999999742 ) ) ;
#1591=CARTESIAN_POINT ( 'NONE',  ( 72.50000000000000000, 9.999999999999998224, 17.49999999999999645 ) ) ;
#1598=CARTESIAN_POINT ( 'NONE',  ( 70.45000000000000284, 8.964466094067244484, 12.50000000000000711 ) ) ;
#1604=DIRECTION ( 'NONE',  ( -1.000000000000000000, -0.000000000000000000, -0.000000000000000000 ) ) ;
#1612=EDGE_CURVE ( 'NONE', #7519, #14091, #3168, .T. ) ;
#1615=CARTESIAN_POINT ( 'NONE',  ( 65.80000000109247082, 7.933012699999995476, 15.85617417291294196 ) ) ;
#1616=CARTESIAN_POINT ( 'NONE',  ( 66.20000000109246230, 9.143825827087050939, 12.93301269999999370 ) ) ;
#1620=CARTESIAN_POINT ( 'NONE',  ( 69.55000000218493028, 7.499999999999996447, 16.03553390593273775 ) ) ;
#1625=CARTESIAN_POINT ( 'NONE',  ( 72.50000000000000000, 9.999999999999998224, 14.99999999999999645 ) ) ;
#1635=EDGE_CURVE ( 'NONE', #7935, #14210, #23634, .T. ) ;
#1643=CARTESIAN_POINT ( 'NONE',  ( 66.55000000218494449, 8.964466094067258695, 12.49999999999999289 ) ) ;
#1651=LINE ( 'NONE', #6817, #13751 ) ;
#1652=CARTESIAN_POINT ( 'NONE',  ( 67.70000000109246230, 7.933012699999995476, 14.14382582708705094 ) ) ;
#1676=CARTESIAN_POINT ( 'NONE',  ( -66.24999999999998579, 7.499999999999995559, 16.03553390593273420 ) ) ;
#1686=CARTESIAN_POINT ( 'NONE',  ( -70.55000000109247082, 8.538419263543522320, 16.46158073645647235 ) ) ;
#1689=CARTESIAN_POINT ( 'NONE',  ( -66.20000000109247651, 12.06698730000000275, 14.14382582708705094 ) ) ;
#1691=CARTESIAN_POINT ( 'NONE',  ( 72.50000000000000000, 9.999999999999998224, 14.99999999999999645 ) ) ;
#1697=CARTESIAN_POINT ( 'NONE',  ( -70.60000000109246798, 7.933012699999995476, 15.85617417291294196 ) ) ;
#1700=CARTESIAN_POINT ( 'NONE',  ( -69.90000000109246514, 9.143825827087049163, 17.06698729999999742 ) ) ;
#1714=VECTOR ( 'NONE', #1604, 1000.000000000000000 ) ;
#1717=VECTOR ( 'NONE', #16961, 999.9999999999997726 ) ;
#1729=CARTESIAN_POINT ( 'NONE',  ( 65.70000000109249072, 9.143825827087049163, 17.06698729999999742 ) ) ;
#1732=CARTESIAN_POINT ( 'NONE',  ( 70.45000000000000284, 8.964466094067258695, 12.49999999999999289 ) ) ;
#1741=FACE_OUTER_BOUND ( 'NONE', #8414, .T. ) ;
#1756=ORIENTED_EDGE ( 'NONE', *, *, #3903, .T. ) ;
#1758=CARTESIAN_POINT ( 'NONE',  ( 69.15000000218495302, 12.50000000000000000, 13.96446609406725869 ) ) ;
#1769=CARTESIAN_POINT ( 'NONE',  ( 72.29999999999998295, 12.50000000000000000, 14.99999999999999645 ) ) ;
#1773=CYLINDRICAL_SURFACE ( 'NONE', #14305, 2.500000000000002220 ) ;
#1792=CARTESIAN_POINT ( 'NONE',  ( -68.39999999999999147, 11.76776695296636888, 16.76776695296636532 ) ) ;
#1802=ORIENTED_EDGE ( 'NONE', *, *, #20831, .F. ) ;
#1804=CARTESIAN_POINT ( 'NONE',  ( -69.70000000109247651, 9.143825827087049163, 17.06698730000000097 ) ) ;
#1807=CARTESIAN_POINT ( 'NONE',  ( -68.90000000109247935, 9.143825827087049163, 17.06698729999999742 ) ) ;
#1815=CARTESIAN_POINT ( 'NONE',  ( -69.40000000109249356, 12.06698730000000275, 14.14382582708705094 ) ) ;
#1817=CARTESIAN_POINT ( 'NONE',  ( -70.15000000109246514, 8.538419263543524096, 13.53841926354352054 ) ) ;
#1821=CARTESIAN_POINT ( 'NONE',  ( 71.89999999999999147, 7.499999999999996447, 14.99999999999999645 ) ) ;
#1829=CARTESIAN_POINT ( 'NONE',  ( -70.14999999999999147, 8.964466094067256918, 17.49999999999999289 ) ) ;
#1846=CARTESIAN_POINT ( 'NONE',  ( 67.79999999999999716, 8.232233047033627571, 16.76776695296636532 ) ) ;
#1848=FACE_OUTER_BOUND ( 'NONE', #12091, .T. ) ;
#1854=CYLINDRICAL_SURFACE ( 'NONE', #2105, 2.500000000000002220 ) ;
#1860=DIRECTION ( 'NONE',  ( -0.000000000000000000, 0.000000000000000000, -1.000000000000000000 ) ) ;
#1870=ORIENTED_EDGE ( 'NONE', *, *, #19457, .F. ) ;
#1874=CARTESIAN_POINT ( 'NONE',  ( 71.60000000109246798, 9.143825827087050939, 12.93301269999999370 ) ) ;
#1885=CARTESIAN_POINT ( 'NONE',  ( 72.50000000000000000, 9.999999999999998224, 14.99999999999999645 ) ) ;
#1888=CARTESIAN_POINT ( 'NONE',  ( -67.74999999999997158, 8.964466094067246260, 17.49999999999999289 ) ) ;
#1896=ORIENTED_EDGE ( 'NONE', *, *, #15551, .T. ) ;
#1904=VERTEX_POINT ( 'NONE', #260 ) ;
#1910=EDGE_CURVE ( 'NONE', #19081, #21422, #12084, .T. ) ;
#1915=CARTESIAN_POINT ( 'NONE',  ( -67.25000000000000000, 8.964466094067258695, 12.49999999999999289 ) ) ;
#1917=CARTESIAN_POINT ( 'NONE',  ( 66.45000000109247651, 9.999999999999998224, 17.06698730000000097 ) ) ;
#1925=CARTESIAN_POINT ( 'NONE',  ( -67.70000000109247651, 10.85617417291294551, 12.93301269999999192 ) ) ;
#1926=ORIENTED_EDGE ( 'NONE', *, *, #9858, .T. ) ;
#1928=CARTESIAN_POINT ( 'NONE',  ( -71.25000000109247367, 12.06698730000000097, 14.99999999999999645 ) ) ;
#1938=CARTESIAN_POINT ( 'NONE',  ( -70.95000000109247651, 11.46158073645647235, 13.53841926354352232 ) ) ;
#1940=CARTESIAN_POINT ( 'NONE',  ( -69.00000000109245946, 10.85617417291294551, 17.06698729999999742 ) ) ;
#1952=ORIENTED_EDGE ( 'NONE', *, *, #11567, .F. ) ;
#1964=CARTESIAN_POINT ( 'NONE',  ( 69.70000000000000284, 9.999999999999998224, 12.49999999999999289 ) ) ;
#1983=EDGE_LOOP ( 'NONE', ( #13921, #10487, #4144, #18954 ) ) ;
#1988=CARTESIAN_POINT ( 'NONE',  ( 70.65000000109247935, 7.933012699999995476, 14.99999999999999645 ) ) ;
#1998=DIRECTION ( 'NONE',  ( 0.000000000000000000, 0.000000000000000000, -1.000000000000000000 ) ) ;
#2008=CARTESIAN_POINT ( 'NONE',  ( 70.89999999999999147, 9.999999999999998224, 17.49999999999999645 ) ) ;
#2019=CARTESIAN_POINT ( 'NONE',  ( 70.50000000109247367, 12.06698729999999919, 15.85617417291294196 ) ) ;
#2027=CARTESIAN_POINT ( 'NONE',  ( 71.70000000109247651, 7.933012699999995476, 14.14382582708705094 ) ) ;
#2035=ADVANCED_FACE ( 'NONE', ( #11563 ), #19293, .F. ) ;
#2038=EDGE_LOOP ( 'NONE', ( #7103, #10512, #10582, #2161 ) ) ;
#2039=CARTESIAN_POINT ( 'NONE',  ( -68.05000000109247082, 9.999999999999998224, 17.06698730000000097 ) ) ;
#2042=CARTESIAN_POINT ( 'NONE',  ( -69.60000000109248219, 12.06698730000000275, 14.14382582708705094 ) ) ;
#2048=CARTESIAN_POINT ( 'NONE',  ( -65.75000000218494733, 8.964466094067258695, 12.49999999999999289 ) ) ;
#2049=CARTESIAN_POINT ( 'NONE',  ( -70.00000000109247367, 7.933012699999995476, 15.85617417291294196 ) ) ;
#2055=EDGE_CURVE ( 'NONE', #23001, #2788, #13699, .T. ) ;
#2064=CARTESIAN_POINT ( 'NONE',  ( -71.45000000218495018, 11.03553390593275374, 12.50000000000001243 ) ) ;
#2074=( BOUNDED_SURFACE ( )  B_SPLINE_SURFACE ( 1, 2, ( 
 ( #21337, #17774, #15764, #12528, #19790, #6530, #1345, #6645, #13849, #13959, #14198, #4833, #12164, #19434, #14559, #9279, #11197, #3862, #7242, #18589, #22170, #23505, #14671, #5658, #9391, #11073, #20256, #7119, #16564, #33, #12872, #9166, #9044, #3733, #14792, #16685, #14432, #22040, #3512, #21823, #10845, #2173, #1817, #12992, #16218, #2049, #21931, #1700, #5426, #21698, #12763, #7590, #18359, #13113, #18471, #7363, #16454, #20127, #16334, #5784, #23629, #5540, #256, #5308, #14911, #1940, #3617, #144, #10957, #12649, #7476, #20372, #3978, #11315, #19909, #20015, #18121, #18234, #15265, #5904, #16928, #7719, #6258, #13696, #2302, #4579, #853, #9996, #11914, #20959, #388, #22289, #18945, #17286, #19182, #9510, #20617, #13578, #506, #9868, #11792, #16807, #11439, #22769, #19063, #15032, #7828, #13229, #20494, #4098, #17163, #18713, #6147, #8077, #9747, #22410, #20846, #2654, #18830, #2416, #4453, #9638, #4336, #15149, #8186, #6019, #13347, #742, #6379 ),
 ( #4224, #15389, #17045, #13470, #620, #11560, #20730, #11675, #15499, #2529, #7947, #22536, #22652, #1432, #6845, #12025, #21548, #19289, #2879, #8654, #17860, #8299, #19403, #17400, #3126, #23366, #12503, #16078, #8540, #22889, #10225, #967, #23235, #6970, #17517, #5160, #8774, #3243, #2767, #14287, #15620, #6503, #12263, #10590, #10109, #13824, #13934, #14169, #1084, #10468, #5045, #21080, #4690, #8427, #12377, #15742, #23011, #6616, #21189, #4805, #17749, #12137, #23118, #1315, #3001, #10352, #21431, #19643, #17641, #1203, #15847, #6731, #21305, #14040, #4927, #19529, #15952, #11045, #16655, #231, #16191, #18443, #1792, #5512, #3362, #1559, #19883, #19990, #12845, #7340, #9256, #8896, #23603, #14645, #18333, #14409, #19760, #8, #14531, #21670, #3486, #21796, #10703, #17982, #9019, #1915, #12966, #18212, #3593, #5279, #16426, #21904, #16540, #20227, #23478, #116, #7090, #18094, #12622, #5758, #5402, #7448, #10821, #5633, #9140, #1676, #16312, #7217, #12740 ) ),
 .UNSPECIFIED., .F., .F., .F. ) 
 B_SPLINE_SURFACE_WITH_KNOTS ( ( 2, 2 ),
 ( 3, 2, 2, 2, 2, 2, 2, 2, 2, 2, 2, 2, 2, 2, 2, 2, 2, 2, 2, 2, 2, 2, 2, 2, 2, 2, 2, 2, 2, 2, 2, 2, 2, 2, 2, 2, 2, 2, 2, 2, 2, 2, 2, 2, 2, 2, 2, 2, 2, 2, 2, 2, 2, 2, 2, 2, 2, 2, 2, 2, 2, 2, 2, 2, 3 ),
 ( 0.000000000000000000, 1.000000000000000000 ),
 ( 0.000000000000000000, 0.01562500000000000000, 0.03125000000000000000, 0.04687500000000000000, 0.06250000000000000000, 0.07812500000000000000, 0.09375000000000000000, 0.1093750000000000000, 0.1250000000000000000, 0.1406250000000000000, 0.1562500000000000000, 0.1718750000000000000, 0.1875000000000000000, 0.2031250000000000000, 0.2187500000000000000, 0.2343750000000000000, 0.2500000000000000000, 0.2656250000000000000, 0.2812500000000000000, 0.2968750000000000000, 0.3125000000000000000, 0.3281250000000000000, 0.3437500000000000000, 0.3593750000000000000, 0.3750000000000000000, 0.3906250000000000000, 0.4062500000000000000, 0.4218750000000000000, 0.4375000000000000000, 0.4531250000000000000, 0.4687500000000000000, 0.4843750000000000000, 0.5000000000000000000, 0.5156250000000000000, 0.5312500000000000000, 0.5468750000000000000, 0.5625000000000000000, 0.5781250000000000000, 0.5937500000000000000, 0.6093750000000000000, 0.6250000000000000000, 0.6406250000000000000, 0.6562500000000000000, 0.6718750000000000000, 0.6875000000000000000, 0.7031250000000000000, 0.7187500000000000000, 0.7343750000000000000, 0.7500000000000000000, 0.7656250000000000000, 0.7812500000000000000, 0.7968750000000000000, 0.8125000000000000000, 0.8281250000000000000, 0.8437500000000000000, 0.8593750000000000000, 0.8750000000000000000, 0.8906250000000000000, 0.9062500000000000000, 0.9218750000000000000, 0.9375000000000000000, 0.9531250000000000000, 0.9687500000000000000, 0.9843750000000000000, 1.000000000000000000 ),
 .UNSPECIFIED. ) 
 GEOMETRIC_REPRESENTATION_ITEM ( )  RATIONAL_B_SPLINE_SURFACE ( (
 ( 1.000000000000000000, 0.9238795325112867385, 1.000000000000000000, 0.9238795325112867385, 1.000000000000000000, 0.9238795325112867385, 1.000000000000000000, 0.9238795325112867385, 1.000000000000000000, 0.9238795325112867385, 1.000000000000000000, 0.9238795325112867385, 1.000000000000000000, 0.9238795325112867385, 1.000000000000000000, 0.9238795325112867385, 1.000000000000000000, 0.9238795325112867385, 1.000000000000000000, 0.9238795325112867385, 1.000000000000000000, 0.9238795325112867385, 1.000000000000000000, 0.9238795325112867385, 1.000000000000000000, 0.9238795325112867385, 1.000000000000000000, 0.9238795325112867385, 1.000000000000000000, 0.9238795325112867385, 1.000000000000000000, 0.9238795325112867385, 1.000000000000000000, 0.9238795325112867385, 1.000000000000000000, 0.9238795325112867385, 1.000000000000000000, 0.9238795325112867385, 1.000000000000000000, 0.9238795325112867385, 1.000000000000000000, 0.9238795325112867385, 1.000000000000000000, 0.9238795325112867385, 1.000000000000000000, 0.9238795325112867385, 1.000000000000000000, 0.9238795325112867385, 1.000000000000000000, 0.9238795325112867385, 1.000000000000000000, 0.9238795325112867385, 1.000000000000000000, 0.9238795325112867385, 1.000000000000000000, 0.9238795325112867385, 1.000000000000000000, 0.9238795325112867385, 1.000000000000000000, 0.9238795325112867385, 1.000000000000000000, 0.9238795325112867385, 1.000000000000000000, 0.9238795325112867385, 1.000000000000000000, 0.9238795325112867385, 1.000000000000000000, 0.9238795325112867385, 1.000000000000000000, 0.9238795325112867385, 1.000000000000000000, 0.9238795325112867385, 1.000000000000000000, 0.9238795325112867385, 1.000000000000000000, 0.9238795325112867385, 1.000000000000000000, 0.9238795325112867385, 1.000000000000000000, 0.9238795325112867385, 1.000000000000000000, 0.9238795325112867385, 1.000000000000000000, 0.9238795325112867385, 1.000000000000000000, 0.9238795325112867385, 1.000000000000000000, 0.9238795325112867385, 1.000000000000000000, 0.9238795325112867385, 1.000000000000000000, 0.9238795325112867385, 1.000000000000000000, 0.9238795325112867385, 1.000000000000000000, 0.9238795325112867385, 1.000000000000000000, 0.9238795325112867385, 1.000000000000000000, 0.9238795325112867385, 1.000000000000000000, 0.9238795325112867385, 1.000000000000000000, 0.9238795325112867385, 1.000000000000000000, 0.9238795325112867385, 1.000000000000000000, 0.9238795325112867385, 1.000000000000000000, 0.9238795325112867385, 1.000000000000000000, 0.9238795325112867385, 1.000000000000000000, 0.9238795325112867385, 1.000000000000000000, 0.9238795325112867385, 1.000000000000000000, 0.9238795325112867385, 1.000000000000000000, 0.9238795325112867385, 1.000000000000000000, 0.9238795325112867385, 1.000000000000000000, 0.9238795325112867385, 1.000000000000000000, 0.9238795325112867385, 1.000000000000000000, 0.9238795325112867385, 1.000000000000000000),
 ( 1.000000000000000000, 0.9238795325112867385, 1.000000000000000000, 0.9238795325112867385, 1.000000000000000000, 0.9238795325112867385, 1.000000000000000000, 0.9238795325112867385, 1.000000000000000000, 0.9238795325112867385, 1.000000000000000000, 0.9238795325112867385, 1.000000000000000000, 0.9238795325112867385, 1.000000000000000000, 0.9238795325112867385, 1.000000000000000000, 0.9238795325112867385, 1.000000000000000000, 0.9238795325112867385, 1.000000000000000000, 0.9238795325112867385, 1.000000000000000000, 0.9238795325112867385, 1.000000000000000000, 0.9238795325112867385, 1.000000000000000000, 0.9238795325112867385, 1.000000000000000000, 0.9238795325112867385, 1.000000000000000000, 0.9238795325112867385, 1.000000000000000000, 0.9238795325112867385, 1.000000000000000000, 0.9238795325112867385, 1.000000000000000000, 0.9238795325112867385, 1.000000000000000000, 0.9238795325112867385, 1.000000000000000000, 0.9238795325112867385, 1.000000000000000000, 0.9238795325112867385, 1.000000000000000000, 0.9238795325112867385, 1.000000000000000000, 0.9238795325112867385, 1.000000000000000000, 0.9238795325112867385, 1.000000000000000000, 0.9238795325112867385, 1.000000000000000000, 0.9238795325112867385, 1.000000000000000000, 0.9238795325112867385, 1.000000000000000000, 0.9238795325112867385, 1.000000000000000000, 0.9238795325112867385, 1.000000000000000000, 0.9238795325112867385, 1.000000000000000000, 0.9238795325112867385, 1.000000000000000000, 0.9238795325112867385, 1.000000000000000000, 0.9238795325112867385, 1.000000000000000000, 0.9238795325112867385, 1.000000000000000000, 0.9238795325112867385, 1.000000000000000000, 0.9238795325112867385, 1.000000000000000000, 0.9238795325112867385, 1.000000000000000000, 0.9238795325112867385, 1.000000000000000000, 0.9238795325112867385, 1.000000000000000000, 0.9238795325112867385, 1.000000000000000000, 0.9238795325112867385, 1.000000000000000000, 0.9238795325112867385, 1.000000000000000000, 0.9238795325112867385, 1.000000000000000000, 0.9238795325112867385, 1.000000000000000000, 0.9238795325112867385, 1.000000000000000000, 0.9238795325112867385, 1.000000000000000000, 0.9238795325112867385, 1.000000000000000000, 0.9238795325112867385, 1.000000000000000000, 0.9238795325112867385, 1.000000000000000000, 0.9238795325112867385, 1.000000000000000000, 0.9238795325112867385, 1.000000000000000000, 0.9238795325112867385, 1.000000000000000000, 0.9238795325112867385, 1.000000000000000000, 0.9238795325112867385, 1.000000000000000000, 0.9238795325112867385, 1.000000000000000000, 0.9238795325112867385, 1.000000000000000000, 0.9238795325112867385, 1.000000000000000000, 0.9238795325112867385, 1.000000000000000000, 0.9238795325112867385, 1.000000000000000000, 0.9238795325112867385, 1.000000000000000000, 0.9238795325112867385, 1.000000000000000000, 0.9238795325112867385, 1.000000000000000000, 0.9238795325112867385, 1.000000000000000000) ) ) 
 REPRESENTATION_ITEM ( '' )  SURFACE ( )  );
#2079=CARTESIAN_POINT ( 'NONE',  ( 68.70000000000000284, 7.499999999999996447, 14.99999999999999645 ) ) ;
#2082=AXIS2_PLACEMENT_3D ( 'NONE', #15831, #16178, #3114 ) ;
#2090=CARTESIAN_POINT ( 'NONE',  ( -70.90000000109246514, 7.933012699999995476, 14.14382582708705094 ) ) ;
#2095=CARTESIAN_POINT ( 'NONE',  ( 71.92500000163870766, 9.999999999999998224, 17.28349365000000049 ) ) ;
#2105=AXIS2_PLACEMENT_3D ( 'NONE', #1625, #11114, #16144 ) ;
#2106=CARTESIAN_POINT ( 'NONE',  ( 70.10000000109246798, 10.85617417291294551, 12.93301269999999370 ) ) ;
#2107=DIRECTION ( 'NONE',  ( 1.000000000000000000, 0.000000000000000000, 0.000000000000000000 ) ) ;
#2108=CARTESIAN_POINT ( 'NONE',  ( 70.40000000109247935, 12.06698730000000275, 14.14382582708705094 ) ) ;
#2118=CARTESIAN_POINT ( 'NONE',  ( -67.50000000109245946, 9.143825827087049163, 17.06698730000000097 ) ) ;
#2125=SURFACE_SIDE_STYLE ('',( #9118 ) ) ;
#2132=CARTESIAN_POINT ( 'NONE',  ( -69.80000000218494449, 9.999999999999998224, 12.49999999999999289 ) ) ;
#2133=ORIENTED_EDGE ( 'NONE', *, *, #21624, .F. ) ;
#2140=CARTESIAN_POINT ( 'NONE',  ( 71.70000000109247651, 7.933012699999995476, 14.14382582708705094 ) ) ;
#2145=CARTESIAN_POINT ( 'NONE',  ( 66.50000000109247367, 9.143825827087049163, 17.06698729999999742 ) ) ;
#2154=CARTESIAN_POINT ( 'NONE',  ( -68.45000000109247651, 9.999999999999998224, 12.93301269999999192 ) ) ;
#2157=CARTESIAN_POINT ( 'NONE',  ( -69.90000000109246514, 9.143825827087049163, 17.06698729999999742 ) ) ;
#2161=ORIENTED_EDGE ( 'NONE', *, *, #22966, .F. ) ;
#2164=ORIENTED_EDGE ( 'NONE', *, *, #19940, .F. ) ;
#2168=CARTESIAN_POINT ( 'NONE',  ( -69.00000000109247367, 7.933012699999995476, 15.85617417291294196 ) ) ;
#2169=CARTESIAN_POINT ( 'NONE',  ( 69.85000000109248219, 7.933012699999995476, 14.99999999999999645 ) ) ;
#2173=CARTESIAN_POINT ( 'NONE',  ( -70.20000000109246230, 9.143825827087050939, 12.93301269999999370 ) ) ;
#2177=CARTESIAN_POINT ( 'NONE',  ( 71.75000000000001421, 8.964466094067221391, 17.49999999999996447 ) ) ;
#2178=STYLED_ITEM ( 'NONE', ( #3945 ), #13661 ) ;
#2185=ORIENTED_EDGE ( 'NONE', *, *, #9823, .F. ) ;
#2187=CARTESIAN_POINT ( 'NONE',  ( -70.09999999999999432, 9.999999999999998224, 17.49999999999999645 ) ) ;
#2192=EDGE_CURVE ( 'NONE', #3210, #6908, #15443, .T. ) ;
#2205=CARTESIAN_POINT ( 'NONE',  ( 67.25000000000000000, 8.964466094067258695, 12.49999999999999289 ) ) ;
#2216=( BOUNDED_CURVE ( )  B_SPLINE_CURVE ( 2, ( #21610, #8712, #10769, #18043, #10986, #1620, #12686, #19941, #3182 ),
 .UNSPECIFIED., .F., .T. ) 
 B_SPLINE_CURVE_WITH_KNOTS ( ( 3, 2, 2, 2, 3 ),
 ( 0.3125000000000002776, 0.3281250000000001665, 0.3437500000000001110, 0.3593750000000000000, 0.3749999999999998890 ),
 .UNSPECIFIED. ) 
 CURVE ( )  GEOMETRIC_REPRESENTATION_ITEM ( )  RATIONAL_B_SPLINE_CURVE ( ( 0.9999999999999986677, 0.9238795325112880708, 1.000000000000000000, 0.9238795325112867385, 1.000000000000000000, 0.9238795325112867385, 1.000000000000000000, 0.9238795325112872936, 0.9999999999999994449 ) ) 
 REPRESENTATION_ITEM ( '' )  );
#2218=CARTESIAN_POINT ( 'NONE',  ( -71.30000000109248504, 9.143825827087049163, 17.06698729999999742 ) ) ;
#2230=CARTESIAN_POINT ( 'NONE',  ( 66.25000000218494733, 8.964466094067258695, 17.50000000000000355 ) ) ;
#2232=VECTOR ( 'NONE', #16777, 1000.000000000000000 ) ;
#2233=CARTESIAN_POINT ( 'NONE',  ( 66.40000000000000568, 8.232233047033629347, 13.23223304703362402 ) ) ;
#2234=CARTESIAN_POINT ( 'NONE',  ( 71.40000000109246514, 10.85617417291294551, 17.06698729999999742 ) ) ;
#2251=CARTESIAN_POINT ( 'NONE',  ( 69.25000000218494733, 12.50000000000000000, 16.03553390593273775 ) ) ;
#2256=CARTESIAN_POINT ( 'NONE',  ( 72.50000000000000000, 9.999999999999998224, 12.49999999999999289 ) ) ;
#2267=CARTESIAN_POINT ( 'NONE',  ( 71.15000000109246514, 11.46158073645647235, 13.53841926354352232 ) ) ;
#2274=CARTESIAN_POINT ( 'NONE',  ( 66.85000000109248219, 9.999999999999998224, 12.93301269999999192 ) ) ;
#2285=CARTESIAN_POINT ( 'NONE',  ( -66.75000000109247367, 8.538419263543524096, 13.53841926354352054 ) ) ;
#2288=CARTESIAN_POINT ( 'NONE',  ( -72.00000000109245946, 12.06698730000000275, 14.14382582708705094 ) ) ;
#2299=CARTESIAN_POINT ( 'NONE',  ( -66.65000000109247935, 7.933012699999995476, 14.99999999999999645 ) ) ;
#2301=CARTESIAN_POINT ( 'NONE',  ( 67.95000000109247651, 11.46158073645647235, 16.46158073645647235 ) ) ;
#2302=CARTESIAN_POINT ( 'NONE',  ( -68.05000000109247082, 12.06698730000000097, 14.99999999999999645 ) ) ;
#2307=EDGE_CURVE ( 'NONE', #16726, #19572, #20022, .T. ) ;
#2326=CARTESIAN_POINT ( 'NONE',  ( -70.75000000218496155, 12.50000000000000000, 13.96446609406725869 ) ) ;
#2330=CARTESIAN_POINT ( 'NONE',  ( 69.64999999999999147, 8.964466094067258695, 12.49999999999999289 ) ) ;
#2338=CARTESIAN_POINT ( 'NONE',  ( -72.25000000109247367, 9.999999999999998224, 17.06698730000000097 ) ) ;
#2339=CARTESIAN_POINT ( 'NONE',  ( -69.84999999999999432, 12.50000000000000000, 13.96446609406725692 ) ) ;
#2343=CARTESIAN_POINT ( 'NONE',  ( -71.40000000109249356, 7.933012699999995476, 15.85617417291294196 ) ) ;
#2352=UNCERTAINTY_MEASURE_WITH_UNIT (LENGTH_MEASURE( 1.000000000000000082E-05 ), #20701, 'distance_accuracy_value', 'NONE');
#2353=CARTESIAN_POINT ( 'NONE',  ( 71.95000000109247651, 11.46158073645647235, 16.46158073645647235 ) ) ;
#2355=CARTESIAN_POINT ( 'NONE',  ( 71.50000000109247367, 9.143825827087049163, 17.06698729999999742 ) ) ;
#2361=CARTESIAN_POINT ( 'NONE',  ( 71.75000000218496155, 11.03553390593273953, 17.50000000000000355 ) ) ;
#2364=CARTESIAN_POINT ( 'NONE',  ( -67.20000000109246230, 12.06698729999999919, 14.14382582708705094 ) ) ;
#2386=CARTESIAN_POINT ( 'NONE',  ( 71.20000000109246230, 12.06698729999999919, 14.14382582708705094 ) ) ;
#2387=ORIENTED_EDGE ( 'NONE', *, *, #22388, .F. ) ;
#2390=CARTESIAN_POINT ( 'NONE',  ( 67.35000000109248219, 8.538419263543522320, 16.46158073645647235 ) ) ;
#2404=CARTESIAN_POINT ( 'NONE',  ( -70.95000000109247651, 8.538419263543524096, 13.53841926354352054 ) ) ;
#2413=CARTESIAN_POINT ( 'NONE',  ( -67.20000000109247651, 10.85617417291294551, 17.06698729999999742 ) ) ;
#2415=CARTESIAN_POINT ( 'NONE',  ( 70.25000000109247367, 12.06698730000000097, 14.99999999999999645 ) ) ;
#2416=CARTESIAN_POINT ( 'NONE',  ( -66.30000000109247082, 10.85617417291294551, 12.93301269999999370 ) ) ;
#2423=CARTESIAN_POINT ( 'NONE',  ( 68.70000000000000284, 7.499999999999996447, 14.99999999999999645 ) ) ;
#2435=ORIENTED_EDGE ( 'NONE', *, *, #3000, .T. ) ;
#2437=CARTESIAN_POINT ( 'NONE',  ( -70.40000000218495302, 7.499999999999996447, 14.99999999999999645 ) ) ;
#2440=CARTESIAN_POINT ( 'NONE',  ( 66.79999999999999716, 11.76776695296636888, 16.76776695296636532 ) ) ;
#2443=CARTESIAN_POINT ( 'NONE',  ( 70.65000000109247935, 7.933012699999995476, 14.99999999999999645 ) ) ;
#2449=CARTESIAN_POINT ( 'NONE',  ( -71.35000000109246798, 11.46158073645647235, 16.46158073645647235 ) ) ;
#2454=CARTESIAN_POINT ( 'NONE',  ( -71.60000000109246798, 9.143825827087050939, 12.93301269999999370 ) ) ;
#2463=CARTESIAN_POINT ( 'NONE',  ( 68.75000000109247367, 11.46158073645647235, 16.46158073645647235 ) ) ;
#2466=CARTESIAN_POINT ( 'NONE',  ( 71.20000000109246230, 12.06698730000000275, 14.14382582708705094 ) ) ;
#2476=CARTESIAN_POINT ( 'NONE',  ( -67.10000000109246798, 10.85617417291294551, 12.93301269999999192 ) ) ;
#2478=DIRECTION ( 'NONE',  ( 0.000000000000000000, 0.000000000000000000, 1.000000000000000000 ) ) ;
#2482=ORIENTED_EDGE ( 'NONE', *, *, #16675, .T. ) ;
#2497=( BOUNDED_CURVE ( )  B_SPLINE_CURVE ( 2, ( #9362, #16775, #17128, #4189, #22625, #15231, #9608, #11401, #22376, #11279, #8040, #2140, #7799, #2499, #7560, #704, #18681, #13195, #11532, #20460, #229, #2386, #2267, #15356, #6228, #13548, #22258, #7913, #4308, #5754, #16900, #9835, #475, #18803, #9715, #2019, #5987, #4068, #3946, #9475, #15117, #22499, #20816, #14882, #13313, #16651, #17012, #4423, #11759, #20340, #354, #7688, #22137, #13085, #18555, #20583, #588, #6108, #13440, #15006, #20702, #11646, #18911, #5871, #17367, #2617, #10079, #10438, #21160, #15924, #8513, #2849, #4659, #15706, #4545, #1282, #19149, #1054, #19499, #826, #17720, #6586, #8390, #935, #13791, #23087, #19372, #19261, #8619, #23201, #6814, #15589, #1172, #21272, #22739, #10198, #3096, #17487, #4774, #12110, #19029, #14135, #21401, #5018, #9960, #17255, #8158, #2966, #15468, #6350, #13664, #6469, #6698, #8273, #10319, #4895, #20925, #11880, #2738, #12231, #22855, #21047, #22981, #11994, #17607, #14013, #13901, #15815, #14258 ),
 .UNSPECIFIED., .F., .F. ) 
 B_SPLINE_CURVE_WITH_KNOTS ( ( 3, 2, 2, 2, 2, 2, 2, 2, 2, 2, 2, 2, 2, 2, 2, 2, 2, 2, 2, 2, 2, 2, 2, 2, 2, 2, 2, 2, 2, 2, 2, 2, 2, 2, 2, 2, 2, 2, 2, 2, 2, 2, 2, 2, 2, 2, 2, 2, 2, 2, 2, 2, 2, 2, 2, 2, 2, 2, 2, 2, 2, 2, 2, 2, 3 ),
 ( 0.000000000000000000, 0.01562500000000000000, 0.03125000000000000000, 0.04687500000000000000, 0.06250000000000000000, 0.07812500000000000000, 0.09375000000000000000, 0.1093750000000000000, 0.1250000000000000000, 0.1406250000000000000, 0.1562500000000000000, 0.1718750000000000000, 0.1875000000000000000, 0.2031250000000000000, 0.2187500000000000000, 0.2343750000000000000, 0.2500000000000000000, 0.2656250000000000000, 0.2812500000000000000, 0.2968750000000000000, 0.3125000000000000000, 0.3281250000000000000, 0.3437500000000000000, 0.3593750000000000000, 0.3750000000000000000, 0.3906250000000000000, 0.4062500000000000000, 0.4218750000000000000, 0.4375000000000000000, 0.4531250000000000000, 0.4687500000000000000, 0.4843750000000000000, 0.5000000000000000000, 0.5156250000000000000, 0.5312500000000000000, 0.5468750000000000000, 0.5625000000000000000, 0.5781250000000000000, 0.5937500000000000000, 0.6093750000000000000, 0.6250000000000000000, 0.6406250000000000000, 0.6562500000000000000, 0.6718750000000000000, 0.6875000000000000000, 0.7031250000000000000, 0.7187500000000000000, 0.7343750000000000000, 0.7500000000000000000, 0.7656250000000000000, 0.7812500000000000000, 0.7968750000000000000, 0.8125000000000000000, 0.8281250000000000000, 0.8437500000000000000, 0.8593750000000000000, 0.8750000000000000000, 0.8906250000000000000, 0.9062500000000000000, 0.9218750000000000000, 0.9375000000000000000, 0.9531250000000000000, 0.9687500000000000000, 0.9843750000000000000, 1.000000000000000000 ),
 .UNSPECIFIED. ) 
 CURVE ( )  GEOMETRIC_REPRESENTATION_ITEM ( )  RATIONAL_B_SPLINE_CURVE ( ( 1.000000000000000000, 0.9238795325112867385, 1.000000000000000000, 0.9238795325112867385, 1.000000000000000000, 0.9238795325112867385, 1.000000000000000000, 0.9238795325112867385, 1.000000000000000000, 0.9238795325112867385, 1.000000000000000000, 0.9238795325112867385, 1.000000000000000000, 0.9238795325112867385, 1.000000000000000000, 0.9238795325112867385, 1.000000000000000000, 0.9238795325112867385, 1.000000000000000000, 0.9238795325112867385, 1.000000000000000000, 0.9238795325112867385, 1.000000000000000000, 0.9238795325112867385, 1.000000000000000000, 0.9238795325112867385, 1.000000000000000000, 0.9238795325112867385, 1.000000000000000000, 0.9238795325112867385, 1.000000000000000000, 0.9238795325112867385, 1.000000000000000000, 0.9238795325112867385, 1.000000000000000000, 0.9238795325112867385, 1.000000000000000000, 0.9238795325112867385, 1.000000000000000000, 0.9238795325112867385, 1.000000000000000000, 0.9238795325112867385, 1.000000000000000000, 0.9238795325112867385, 1.000000000000000000, 0.9238795325112867385, 1.000000000000000000, 0.9238795325112867385, 1.000000000000000000, 0.9238795325112867385, 1.000000000000000000, 0.9238795325112867385, 1.000000000000000000, 0.9238795325112867385, 1.000000000000000000, 0.9238795325112867385, 1.000000000000000000, 0.9238795325112867385, 1.000000000000000000, 0.9238795325112867385, 1.000000000000000000, 0.9238795325112867385, 1.000000000000000000, 0.9238795325112867385, 1.000000000000000000, 0.9238795325112867385, 1.000000000000000000, 0.9238795325112867385, 1.000000000000000000, 0.9238795325112867385, 1.000000000000000000, 0.9238795325112867385, 1.000000000000000000, 0.9238795325112867385, 1.000000000000000000, 0.9238795325112867385, 1.000000000000000000, 0.9238795325112867385, 1.000000000000000000, 0.9238795325112867385, 1.000000000000000000, 0.9238795325112867385, 1.000000000000000000, 0.9238795325112867385, 1.000000000000000000, 0.9238795325112867385, 1.000000000000000000, 0.9238795325112867385, 1.000000000000000000, 0.9238795325112867385, 1.000000000000000000, 0.9238795325112867385, 1.000000000000000000, 0.9238795325112867385, 1.000000000000000000, 0.9238795325112867385, 1.000000000000000000, 0.9238795325112867385, 1.000000000000000000, 0.9238795325112867385, 1.000000000000000000, 0.9238795325112867385, 1.000000000000000000, 0.9238795325112867385, 1.000000000000000000, 0.9238795325112867385, 1.000000000000000000, 0.9238795325112867385, 1.000000000000000000, 0.9238795325112867385, 1.000000000000000000, 0.9238795325112867385, 1.000000000000000000, 0.9238795325112867385, 1.000000000000000000, 0.9238795325112867385, 1.000000000000000000, 0.9238795325112867385, 1.000000000000000000, 0.9238795325112867385, 1.000000000000000000, 0.9238795325112867385, 1.000000000000000000, 0.9238795325112867385, 1.000000000000000000, 0.9238795325112867385, 1.000000000000000000, 0.9238795325112867385, 1.000000000000000000 ) ) 
 REPRESENTATION_ITEM ( '' )  );
#2499=CARTESIAN_POINT ( 'NONE',  ( 71.60000000109246798, 7.933012699999995476, 15.85617417291294196 ) ) ;
#2505=CARTESIAN_POINT ( 'NONE',  ( 68.90000000109246514, 12.06698730000000275, 15.85617417291294196 ) ) ;
#2509=ORIENTED_EDGE ( 'NONE', *, *, #21073, .T. ) ;
#2519=CARTESIAN_POINT ( 'NONE',  ( -68.30000000109247082, 9.143825827087049163, 17.06698729999999742 ) ) ;
#2526=CARTESIAN_POINT ( 'NONE',  ( -68.95000000109247651, 8.538419263543522320, 16.46158073645647235 ) ) ;
#2527=CARTESIAN_POINT ( 'NONE',  ( 68.55000000109247082, 11.46158073645647235, 13.53841926354352232 ) ) ;
#2529=CARTESIAN_POINT ( 'NONE',  ( -72.05000000000001137, 8.964466094067258695, 12.49999999999999289 ) ) ;
#2543=EDGE_LOOP ( 'NONE', ( #16291, #1568, #17086, #21048 ) ) ;
#2549=CARTESIAN_POINT ( 'NONE',  ( -71.60000000218494165, 12.50000000000000000, 14.99999999999999645 ) ) ;
#2552=CARTESIAN_POINT ( 'NONE',  ( -70.95000000000000284, 8.964466094067294222, 17.50000000000003908 ) ) ;
#2554=CARTESIAN_POINT ( 'NONE',  ( 68.95000000109247651, 8.538419263543522320, 16.46158073645647235 ) ) ;
#2561=CARTESIAN_POINT ( 'NONE',  ( -71.90000000109246514, 10.85617417291294551, 12.93301269999999192 ) ) ;
#2565=ORIENTED_EDGE ( 'NONE', *, *, #23408, .T. ) ;
#2568=FACE_OUTER_BOUND ( 'NONE', #18804, .T. ) ;
#2574=EDGE_CURVE ( 'NONE', #14091, #14025, #23666, .T. ) ;
#2581=CARTESIAN_POINT ( 'NONE',  ( 68.10000000109246798, 9.143825827087049163, 17.06698729999999742 ) ) ;
#2583=CARTESIAN_POINT ( 'NONE',  ( 67.20000000109247651, 12.06698730000000275, 14.14382582708705094 ) ) ;
#2589=CARTESIAN_POINT ( 'NONE',  ( 66.80000000218494449, 12.50000000000000000, 14.99999999999999645 ) ) ;
#2593=AXIS2_PLACEMENT_3D ( 'NONE', #10126, #6394, #21449 ) ;
#2600=ORIENTED_EDGE ( 'NONE', *, *, #14803, .F. ) ;
#2601=CARTESIAN_POINT ( 'NONE',  ( -66.20000000218495018, 9.999999999999998224, 17.49999999999999645 ) ) ;
#2605=CARTESIAN_POINT ( 'NONE',  ( -70.60000000218494165, 9.999999999999998224, 12.49999999999999289 ) ) ;
#2610=CARTESIAN_POINT ( 'NONE',  ( 72.05000000109247082, 9.999999999999998224, 17.06698730000000097 ) ) ;
#2612=CARTESIAN_POINT ( 'NONE',  ( 71.60000000218494165, 12.50000000000000000, 14.99999999999999645 ) ) ;
#2615=AXIS2_PLACEMENT_3D ( 'NONE', #468, #11525, #4301 ) ;
#2617=CARTESIAN_POINT ( 'NONE',  ( 69.00000000109245946, 10.85617417291294551, 17.06698730000000097 ) ) ;
#2619=CARTESIAN_POINT ( 'NONE',  ( 72.50000000000000000, 9.999999999999998224, 12.49999999999999289 ) ) ;
#2623=CARTESIAN_POINT ( 'NONE',  ( 70.80000000109245661, 7.933012699999995476, 15.85617417291294196 ) ) ;
#2636=CARTESIAN_POINT ( 'NONE',  ( -65.80000000109247082, 7.933012699999995476, 15.85617417291294196 ) ) ;
#2638=CARTESIAN_POINT ( 'NONE',  ( -67.05000000109247082, 9.999999999999998224, 12.93301269999999192 ) ) ;
#2642=CARTESIAN_POINT ( 'NONE',  ( 65.97500000054623115, 9.999999999999998224, 17.28349365000000049 ) ) ;
#2651=CARTESIAN_POINT ( 'NONE',  ( -66.15000000109247935, 11.46158073645647235, 13.53841926354352232 ) ) ;
#2652=CARTESIAN_POINT ( 'NONE',  ( 69.45000000109247651, 12.06698730000000097, 14.99999999999999645 ) ) ;
#2654=CARTESIAN_POINT ( 'NONE',  ( -66.40000000109247935, 12.06698730000000275, 14.14382582708705094 ) ) ;
#2660=CARTESIAN_POINT ( 'NONE',  ( 71.39999999999999147, 11.76776695296636888, 13.23223304703362579 ) ) ;
#2665=ORIENTED_EDGE ( 'NONE', *, *, #12495, .T. ) ;
#2677=FACE_OUTER_BOUND ( 'NONE', #20385, .T. ) ;
#2681=ORIENTED_EDGE ( 'NONE', *, *, #18759, .F. ) ;
#2683=CARTESIAN_POINT ( 'NONE',  ( -69.60000000218495586, 7.499999999999996447, 14.99999999999999645 ) ) ;
#2688=CARTESIAN_POINT ( 'NONE',  ( 70.70000000109247651, 7.933012699999995476, 14.14382582708705094 ) ) ;
#2695=CARTESIAN_POINT ( 'NONE',  ( -70.05000000109247082, 7.933012699999995476, 14.99999999999999645 ) ) ;
#2696=CARTESIAN_POINT ( 'NONE',  ( -70.15000000218495302, 11.03553390593276973, 17.49999999999997158 ) ) ;
#2698=ORIENTED_EDGE ( 'NONE', *, *, #17416, .T. ) ;
#2708=CARTESIAN_POINT ( 'NONE',  ( 67.10000000109248219, 12.06698730000000275, 15.85617417291294196 ) ) ;
#2710=CARTESIAN_POINT ( 'NONE',  ( 67.05000000109247082, 9.999999999999998224, 12.93301269999999192 ) ) ;
#2717=CARTESIAN_POINT ( 'NONE',  ( 72.50000000000000000, 9.999999999999998224, 14.99999999999999645 ) ) ;
#2733=CARTESIAN_POINT ( 'NONE',  ( 71.15000000218493881, 7.499999999999995559, 16.03553390593273420 ) ) ;
#2738=CARTESIAN_POINT ( 'NONE',  ( 66.35000000109246798, 11.46158073645647235, 13.53841926354352232 ) ) ;
#2743=CARTESIAN_POINT ( 'NONE',  ( 69.15000000109246514, 8.538419263543522320, 16.46158073645647235 ) ) ;
#2755=CARTESIAN_POINT ( 'NONE',  ( -68.40000000109246514, 7.933012699999995476, 15.85617417291294196 ) ) ;
#2758=ORIENTED_EDGE ( 'NONE', *, *, #5286, .F. ) ;
#2766=CARTESIAN_POINT ( 'NONE',  ( 66.15000000109247935, 11.46158073645647235, 13.53841926354352232 ) ) ;
#2767=CARTESIAN_POINT ( 'NONE',  ( -70.59999999999999432, 11.76776695296636888, 13.23223304703362579 ) ) ;
#2768=CARTESIAN_POINT ( 'NONE',  ( -71.50000000000000000, 12.50000000000000000, 14.99999999999999645 ) ) ;
#2769=ADVANCED_FACE ( 'NONE', ( #5739 ), #13068, .T. ) ;
#2774=CARTESIAN_POINT ( 'NONE',  ( 71.54999999999998295, 12.50000000000000000, 16.03553390593273775 ) ) ;
#2779=ORIENTED_EDGE ( 'NONE', *, *, #4855, .T. ) ;
#2786=CARTESIAN_POINT ( 'NONE',  ( 72.50000000000000000, 9.999999999999998224, 14.99999999999999645 ) ) ;
#2788=VERTEX_POINT ( 'NONE', #4645 ) ;
#2797=CARTESIAN_POINT ( 'NONE',  ( 66.54999999999999716, 11.03553390593273598, 12.49999999999999289 ) ) ;
#2800=CARTESIAN_POINT ( 'NONE',  ( 69.20000000109246230, 9.143825827087050939, 12.93301269999999370 ) ) ;
#2808=CARTESIAN_POINT ( 'NONE',  ( -70.20000000109246230, 9.143825827087052716, 12.93301269999999192 ) ) ;
#2818=CARTESIAN_POINT ( 'NONE',  ( -66.54999999999999716, 11.03553390593269867, 12.49999999999995559 ) ) ;
#2822=CARTESIAN_POINT ( 'NONE',  ( 67.70000000109246230, 10.85617417291294551, 12.93301269999999370 ) ) ;
#2823=CARTESIAN_POINT ( 'NONE',  ( 69.10000000109246798, 9.143825827087049163, 17.06698729999999742 ) ) ;
#2829=CARTESIAN_POINT ( 'NONE',  ( 67.80000000218494449, 9.999999999999998224, 17.49999999999999645 ) ) ;
#2831=EDGE_LOOP ( 'NONE', ( #2698, #5888, #1244, #23030 ) ) ;
#2838=AXIS2_PLACEMENT_3D ( 'NONE', #11973, #13524, #11619 ) ;
#2843=CARTESIAN_POINT ( 'NONE',  ( 72.00000000109248788, 10.85617417291294551, 17.06698730000000097 ) ) ;
#2849=CARTESIAN_POINT ( 'NONE',  ( 68.70000000109247651, 10.85617417291294551, 12.93301269999999192 ) ) ;
#2853=CARTESIAN_POINT ( 'NONE',  ( 68.65000000109246514, 9.999999999999998224, 12.93301269999999192 ) ) ;
#2855=FACE_OUTER_BOUND ( 'NONE', #14027, .T. ) ;
#2865=EDGE_CURVE ( 'NONE', #12453, #19131, #1489, .T. ) ;
#2868=CARTESIAN_POINT ( 'NONE',  ( -68.80000000109247082, 12.06698730000000275, 14.14382582708705094 ) ) ;
#2878=CARTESIAN_POINT ( 'NONE',  ( 67.20000000109246230, 10.85617417291294551, 17.06698730000000097 ) ) ;
#2879=CARTESIAN_POINT ( 'NONE',  ( -71.59999999999999432, 11.76776695296636888, 16.76776695296636532 ) ) ;
#2886=CARTESIAN_POINT ( 'NONE',  ( 67.05000000218494449, 8.964466094067246260, 17.49999999999999289 ) ) ;
#2905=CARTESIAN_POINT ( 'NONE',  ( -66.85000000218495586, 12.50000000000000000, 16.03553390593273420 ) ) ;
#2911=CARTESIAN_POINT ( 'NONE',  ( 68.80000000109247082, 10.85617417291294551, 17.06698729999999742 ) ) ;
#2918=CARTESIAN_POINT ( 'NONE',  ( -69.35000000109246798, 8.538419263543524096, 13.53841926354352054 ) ) ;
#2935=CARTESIAN_POINT ( 'NONE',  ( 66.80000000109247082, 9.143825827087050939, 12.93301269999999370 ) ) ;
#2937=CARTESIAN_POINT ( 'NONE',  ( 66.70000000109246230, 9.143825827087049163, 17.06698729999999742 ) ) ;
#2949=CARTESIAN_POINT ( 'NONE',  ( -66.90000000000000568, 9.999999999999998224, 17.49999999999999645 ) ) ;
#2958=CARTESIAN_POINT ( 'NONE',  ( 65.80000000218494449, 9.999999999999998224, 12.49999999999999289 ) ) ;
#2962=CARTESIAN_POINT ( 'NONE',  ( 69.95000000218493597, 12.50000000000000000, 13.96446609406725869 ) ) ;
#2966=CARTESIAN_POINT ( 'NONE',  ( 66.90000000109247935, 7.933012699999995476, 14.14382582708705094 ) ) ;
#2972=CARTESIAN_POINT ( 'NONE',  ( 69.95000000109247651, 8.538419263543522320, 16.46158073645647235 ) ) ;
#2979=CARTESIAN_POINT ( 'NONE',  ( 66.65000000000000568, 12.50000000000000000, 13.96446609406725692 ) ) ;
#2985=CARTESIAN_POINT ( 'NONE',  ( -68.60000000109246798, 9.143825827087050939, 12.93301269999999370 ) ) ;
#2995=CARTESIAN_POINT ( 'NONE',  ( -66.75000000218494733, 12.50000000000000000, 13.96446609406725692 ) ) ;
#3000=EDGE_CURVE ( 'NONE', #2788, #20225, #15910, .T. ) ;
#3001=CARTESIAN_POINT ( 'NONE',  ( -69.29999999999999716, 9.999999999999998224, 17.49999999999999645 ) ) ;
#3007=CYLINDRICAL_SURFACE ( 'NONE', #23424, 2.500000000000002220 ) ;
#3010=ORIENTED_EDGE ( 'NONE', *, *, #8593, .F. ) ;
#3012=VERTEX_POINT ( 'NONE', #2949 ) ;
#3014=CARTESIAN_POINT ( 'NONE',  ( -70.35000000109248219, 11.46158073645647235, 16.46158073645647235 ) ) ;
#3016=AXIS2_PLACEMENT_3D ( 'NONE', #5876, #11407, #18684 ) ;
#3027=CARTESIAN_POINT ( 'NONE',  ( -65.95000000218495018, 12.50000000000000000, 13.96446609406725869 ) ) ;
#3030=APPLICATION_CONTEXT ( 'automotive_design' ) ;
#3037=CARTESIAN_POINT ( 'NONE',  ( 66.99999999999998579, 8.232233047033627571, 16.76776695296636532 ) ) ;
#3045=CARTESIAN_POINT ( 'NONE',  ( -69.80000000109247082, 10.85617417291294551, 17.06698730000000097 ) ) ;
#3055=ORIENTED_EDGE ( 'NONE', *, *, #18040, .T. ) ;
#3068=CARTESIAN_POINT ( 'NONE',  ( 67.45000000109246230, 9.999999999999998224, 17.06698730000000097 ) ) ;
#3070=CARTESIAN_POINT ( 'NONE',  ( -65.80000000218494449, 9.999999999999998224, 12.49999999999999289 ) ) ;
#3076=FACE_OUTER_BOUND ( 'NONE', #18732, .T. ) ;
#3086=CARTESIAN_POINT ( 'NONE',  ( -67.64999999999999147, 11.03553390593272887, 17.50000000000001066 ) ) ;
#3092=CARTESIAN_POINT ( 'NONE',  ( 67.70000000218493597, 11.76776695296636888, 16.76776695296636532 ) ) ;
#3093=DIRECTION ( 'NONE',  ( -1.000000000000000000, -0.000000000000000000, -0.000000000000000000 ) ) ;
#3096=CARTESIAN_POINT ( 'NONE',  ( 67.45000000109246230, 9.999999999999998224, 17.06698730000000097 ) ) ;
#3102=CARTESIAN_POINT ( 'NONE',  ( 68.15000000109246514, 11.46158073645647235, 16.46158073645647235 ) ) ;
#3111=CARTESIAN_POINT ( 'NONE',  ( 0.000000000000000000, 0.000000000000000000, 0.000000000000000000 ) ) ;
#3114=DIRECTION ( 'NONE',  ( 0.000000000000000000, 0.000000000000000000, 1.000000000000000000 ) ) ;
#3117=CARTESIAN_POINT ( 'NONE',  ( -65.85000000218495586, 11.03553390593269867, 12.49999999999995559 ) ) ;
#3123=CARTESIAN_POINT ( 'NONE',  ( -67.90000000218495302, 8.232233047033627571, 16.76776695296636532 ) ) ;
#3125=LINE ( 'NONE', #18092, #9851 ) ;
#3126=CARTESIAN_POINT ( 'NONE',  ( -71.29999999999998295, 9.999999999999998224, 12.49999999999999289 ) ) ;
#3130=( BOUNDED_CURVE ( )  B_SPLINE_CURVE ( 2, ( #5109, #16145, #7039, #14355, #21618, #19827, #8970, #16261, #9672 ),
 .UNSPECIFIED., .F., .F. ) 
 B_SPLINE_CURVE_WITH_KNOTS ( ( 3, 2, 2, 2, 3 ),
 ( 0.1875000000000010270, 0.2031250000000009437, 0.2187500000000008327, 0.2343750000000007494, 0.2500000000000006661 ),
 .UNSPECIFIED. ) 
 CURVE ( )  GEOMETRIC_REPRESENTATION_ITEM ( )  RATIONAL_B_SPLINE_CURVE ( ( 0.9999999999999950040, 0.9238795325112917345, 1.000000000000000000, 0.9238795325112867385, 1.000000000000000000, 0.9238795325112867385, 1.000000000000000000, 0.9238795325112835188, 1.000000000000003331 ) ) 
 REPRESENTATION_ITEM ( '' )  );
#3138=CARTESIAN_POINT ( 'NONE',  ( -67.15000000109247935, 11.46158073645647235, 16.46158073645647235 ) ) ;
#3139=CYLINDRICAL_SURFACE ( 'NONE', #17820, 2.500000000000002220 ) ;
#3144=DIRECTION ( 'NONE',  ( 0.000000000000000000, 0.000000000000000000, 1.000000000000000000 ) ) ;
#3147=CARTESIAN_POINT ( 'NONE',  ( -68.90000000218495302, 8.232233047033629347, 13.23223304703362402 ) ) ;
#3168=( BOUNDED_CURVE ( )  B_SPLINE_CURVE ( 2, ( #7000, #18016, #1470, #23150, #17669, #5313, #3037, #14319, #19915 ),
 .UNSPECIFIED., .F., .F. ) 
 B_SPLINE_CURVE_WITH_KNOTS ( ( 3, 2, 2, 2, 3 ),
 ( 0.8124999999999993339, 0.8281249999999992228, 0.8437499999999991118, 0.8593749999999991118, 0.8749999999999990008 ),
 .UNSPECIFIED. ) 
 CURVE ( )  GEOMETRIC_REPRESENTATION_ITEM ( )  RATIONAL_B_SPLINE_CURVE ( ( 1.000000000000003331, 0.9238795325112835188, 1.000000000000000000, 0.9238795325112867385, 1.000000000000000000, 0.9238795325112867385, 1.000000000000000000, 0.9238795325112916235, 0.9999999999999951150 ) ) 
 REPRESENTATION_ITEM ( '' )  );
#3179=CARTESIAN_POINT ( 'NONE',  ( 71.64999999999997726, 11.03553390593273598, 17.50000000000000355 ) ) ;
#3182=CARTESIAN_POINT ( 'NONE',  ( 69.40000000218495302, 9.999999999999998224, 17.49999999999999645 ) ) ;
#3191=CARTESIAN_POINT ( 'NONE',  ( 68.39999999999999147, 11.76776695296636888, 16.76776695296636532 ) ) ;
#3196=CARTESIAN_POINT ( 'NONE',  ( -67.59999999999999432, 11.76776695296636888, 16.76776695296636532 ) ) ;
#3200=CARTESIAN_POINT ( 'NONE',  ( -69.64999999999997726, 8.964466094067285340, 12.49999999999996980 ) ) ;
#3204=CARTESIAN_POINT ( 'NONE',  ( 66.45000000218495018, 7.499999999999995559, 13.96446609406725692 ) ) ;
#3208=CARTESIAN_POINT ( 'NONE',  ( 72.50000000000000000, 9.999999999999998224, 12.49999999999999289 ) ) ;
#3210=VERTEX_POINT ( 'NONE', #20057 ) ;
#3213=CARTESIAN_POINT ( 'NONE',  ( 66.25000000109245946, 9.999999999999998224, 12.93301269999999192 ) ) ;
#3215=CYLINDRICAL_SURFACE ( 'NONE', #16254, 2.500000000000002220 ) ;
#3235=ADVANCED_FACE ( 'NONE', ( #20175 ), #19951, .F. ) ;
#3237=ADVANCED_FACE ( 'NONE', ( #16376 ), #7404, .T. ) ;
#3238=CARTESIAN_POINT ( 'NONE',  ( -68.15000000218495302, 8.964466094067214286, 12.50000000000004086 ) ) ;
#3239=CARTESIAN_POINT ( 'NONE',  ( 67.15000000109247935, 11.46158073645647235, 16.46158073645647235 ) ) ;
#3243=CARTESIAN_POINT ( 'NONE',  ( -70.64999999999999147, 12.50000000000000000, 13.96446609406725869 ) ) ;
#3249=CARTESIAN_POINT ( 'NONE',  ( 67.99999999999998579, 8.232233047033629347, 13.23223304703362402 ) ) ;
#3256=CARTESIAN_POINT ( 'NONE',  ( -66.10000000109248219, 10.85617417291294551, 12.93301269999999370 ) ) ;
#3269=CARTESIAN_POINT ( 'NONE',  ( -66.95000000218496439, 11.03553390593273598, 17.50000000000000355 ) ) ;
#3282=CARTESIAN_POINT ( 'NONE',  ( -68.34999999999999432, 12.50000000000000000, 16.03553390593273775 ) ) ;
#3292=ORIENTED_EDGE ( 'NONE', *, *, #1910, .F. ) ;
#3295=ORIENTED_EDGE ( 'NONE', *, *, #17438, .F. ) ;
#3297=CARTESIAN_POINT ( 'NONE',  ( 72.50000000000000000, 9.999999999999998224, 14.99999999999999645 ) ) ;
#3299=CARTESIAN_POINT ( 'NONE',  ( 66.55000000109247082, 8.538419263543522320, 16.46158073645647235 ) ) ;
#3300=CARTESIAN_POINT ( 'NONE',  ( 71.09999999999999432, 7.499999999999996447, 14.99999999999999645 ) ) ;
#3314=VERTEX_POINT ( 'NONE', #18508 ) ;
#3316=CARTESIAN_POINT ( 'NONE',  ( 71.30000000109248504, 9.143825827087049163, 17.06698729999999742 ) ) ;
#3320=ORIENTED_EDGE ( 'NONE', *, *, #9461, .F. ) ;
#3322=CARTESIAN_POINT ( 'NONE',  ( 68.15000000218495302, 8.964466094067258695, 12.49999999999999289 ) ) ;
#3325=LINE ( 'NONE', #3208, #17521 ) ;
#3328=VECTOR ( 'NONE', #8213, 1000.000000000000000 ) ;
#3329=EDGE_CURVE ( 'NONE', #9434, #23001, #16265, .T. ) ;
#3334=CARTESIAN_POINT ( 'NONE',  ( 68.20000000109246230, 10.85617417291294551, 17.06698729999999742 ) ) ;
#3359=ADVANCED_FACE ( 'NONE', ( #2568 ), #5479, .F. ) ;
#3362=CARTESIAN_POINT ( 'NONE',  ( -68.29999999999999716, 12.50000000000000000, 14.99999999999999645 ) ) ;
#3379=CARTESIAN_POINT ( 'NONE',  ( -67.45000000109246230, 7.933012699999995476, 14.99999999999999645 ) ) ;
#3388=CARTESIAN_POINT ( 'NONE',  ( -65.40000000218495302, 9.999999999999998224, 17.49999999999999645 ) ) ;
#3404=CARTESIAN_POINT ( 'NONE',  ( 70.50000000000000000, 9.999999999999998224, 12.49999999999999289 ) ) ;
#3407=FACE_OUTER_BOUND ( 'NONE', #14859, .T. ) ;
#3425=CARTESIAN_POINT ( 'NONE',  ( 71.95000000000001705, 7.499999999999995559, 13.96446609406725692 ) ) ;
#3435=ORIENTED_EDGE ( 'NONE', *, *, #23408, .F. ) ;
#3451=CARTESIAN_POINT ( 'NONE',  ( 68.60000000218495586, 9.999999999999998224, 17.49999999999999645 ) ) ;
#3462=LINE ( 'NONE', #10799, #9766 ) ;
#3468=CARTESIAN_POINT ( 'NONE',  ( -72.29999999999998295, 12.50000000000000000, 14.99999999999999645 ) ) ;
#3474=CARTESIAN_POINT ( 'NONE',  ( -66.20000000218495018, 9.999999999999998224, 17.49999999999999645 ) ) ;
#3480=CARTESIAN_POINT ( 'NONE',  ( -66.44999999999998863, 8.964466094067219615, 12.50000000000003553 ) ) ;
#3481=CIRCLE ( 'NONE', #18782, 2.500000000000002220 ) ;
#3486=CARTESIAN_POINT ( 'NONE',  ( -67.49999999999998579, 12.50000000000000000, 14.99999999999999645 ) ) ;
#3491=CARTESIAN_POINT ( 'NONE',  ( -66.85000000109246798, 7.933012699999995476, 14.99999999999999645 ) ) ;
#3494=CARTESIAN_POINT ( 'NONE',  ( -66.35000000218495586, 7.499999999999996447, 16.03553390593273775 ) ) ;
#3500=CARTESIAN_POINT ( 'NONE',  ( -66.35000000109248219, 11.46158073645647235, 16.46158073645647235 ) ) ;
#3509=CARTESIAN_POINT ( 'NONE',  ( -70.10000000109246798, 10.85617417291294551, 12.93301269999999370 ) ) ;
#3510=EDGE_CURVE ( 'NONE', #4668, #14091, #23589, .T. ) ;
#3512=CARTESIAN_POINT ( 'NONE',  ( -70.35000000109246798, 11.46158073645647235, 13.53841926354352232 ) ) ;
#3514=DIRECTION ( 'NONE',  ( -1.000000000000000000, -0.000000000000000000, -0.000000000000000000 ) ) ;
#3534=ORIENTED_EDGE ( 'NONE', *, *, #10135, .F. ) ;
#3539=CARTESIAN_POINT ( 'NONE',  ( 65.85000000109246798, 9.999999999999998224, 17.06698730000000097 ) ) ;
#3550=CARTESIAN_POINT ( 'NONE',  ( 72.50000000000000000, 9.999999999999998224, 14.99999999999999645 ) ) ;
#3562=CARTESIAN_POINT ( 'NONE',  ( 66.40000000218495302, 7.499999999999996447, 14.99999999999999645 ) ) ;
#3563=CARTESIAN_POINT ( 'NONE',  ( 72.50000000000000000, 9.999999999999998224, 14.99999999999999645 ) ) ;
#3571=CARTESIAN_POINT ( 'NONE',  ( 66.40000000109247935, 12.06698730000000275, 14.14382582708705094 ) ) ;
#3579=SHAPE_REPRESENTATION_RELATIONSHIP ( 'NONE' , 'NONE' ,  #9307, #19874 ) ;
#3585=CARTESIAN_POINT ( 'NONE',  ( 69.84999999999999432, 12.50000000000000000, 13.96446609406725692 ) ) ;
#3590=CARTESIAN_POINT ( 'NONE',  ( -67.85000000218494165, 8.964466094067287116, 17.50000000000002487 ) ) ;
#3593=CARTESIAN_POINT ( 'NONE',  ( -67.09999999999999432, 7.499999999999996447, 14.99999999999999645 ) ) ;
#3601=CARTESIAN_POINT ( 'NONE',  ( -66.25000000218494733, 8.964466094067207180, 17.49999999999995026 ) ) ;
#3603=CARTESIAN_POINT ( 'NONE',  ( -69.85000000109248219, 7.933012699999995476, 14.99999999999999645 ) ) ;
#3606=CARTESIAN_POINT ( 'NONE',  ( -66.50000000109247367, 9.143825827087049163, 17.06698729999999742 ) ) ;
#3615=CARTESIAN_POINT ( 'NONE',  ( -65.65000000218493881, 7.499999999999995559, 13.96446609406725692 ) ) ;
#3617=CARTESIAN_POINT ( 'NONE',  ( -68.95000000109247651, 11.46158073645647235, 16.46158073645647235 ) ) ;
#3626=CARTESIAN_POINT ( 'NONE',  ( -68.49999999999998579, 9.999999999999998224, 17.49999999999999645 ) ) ;
#3641=ORIENTED_EDGE ( 'NONE', *, *, #2865, .T. ) ;
#3646=CARTESIAN_POINT ( 'NONE',  ( 72.44999999999998863, 11.03553390593273598, 17.50000000000000355 ) ) ;
#3672=CARTESIAN_POINT ( 'NONE',  ( 65.60000000218495586, 7.499999999999996447, 14.99999999999999645 ) ) ;
#3708=CARTESIAN_POINT ( 'NONE',  ( 66.70000000109246230, 7.933012699999995476, 14.14382582708705094 ) ) ;
#3717=CARTESIAN_POINT ( 'NONE',  ( -68.80000000109247082, 10.85617417291294551, 17.06698730000000097 ) ) ;
#3718=VERTEX_POINT ( 'NONE', #691 ) ;
#3720=CARTESIAN_POINT ( 'NONE',  ( -72.05000000109245661, 12.06698730000000097, 14.99999999999999645 ) ) ;
#3724=VECTOR ( 'NONE', #8124, 1000.000000000000000 ) ;
#3726=PRODUCT_DEFINITION ( 'UNKNOWN', '', #11848, #923 ) ;
#3731=CARTESIAN_POINT ( 'NONE',  ( -71.25000000109248788, 9.999999999999998224, 17.06698730000000097 ) ) ;
#3733=CARTESIAN_POINT ( 'NONE',  ( -70.60000000109246798, 10.85617417291294551, 17.06698729999999742 ) ) ;
#3754=( BOUNDED_CURVE ( )  B_SPLINE_CURVE ( 2, ( #22445, #15069, #22326, #5940, #13266, #2339, #4490, #21002, #15544 ),
 .UNSPECIFIED., .F., .F. ) 
 B_SPLINE_CURVE_WITH_KNOTS ( ( 3, 2, 2, 2, 3 ),
 ( 0.3749999999999998890, 0.3906249999999997780, 0.4062499999999996669, 0.4218749999999996114, 0.4374999999999995004 ),
 .UNSPECIFIED. ) 
 CURVE ( )  GEOMETRIC_REPRESENTATION_ITEM ( )  RATIONAL_B_SPLINE_CURVE ( ( 1.000000000000000444, 0.9238795325112861834, 1.000000000000000000, 0.9238795325112867385, 1.000000000000000000, 0.9238795325112867385, 1.000000000000000000, 0.9238795325112891810, 0.9999999999999975575 ) ) 
 REPRESENTATION_ITEM ( '' )  );
#3764=CARTESIAN_POINT ( 'NONE',  ( 69.29999999999999716, 9.999999999999998224, 17.49999999999999645 ) ) ;
#3795=CARTESIAN_POINT ( 'NONE',  ( 70.55000000109247082, 8.538419263543522320, 16.46158073645647235 ) ) ;
#3799=CARTESIAN_POINT ( 'NONE',  ( 71.00000000109245946, 9.143825827087050939, 12.93301269999999370 ) ) ;
#3803=EDGE_CURVE ( 'NONE', #14363, #19081, #18792, .T. ) ;
#3810=CARTESIAN_POINT ( 'NONE',  ( 72.20000000000000284, 11.76776695296636888, 13.23223304703362579 ) ) ;
#3814=CARTESIAN_POINT ( 'NONE',  ( -70.20000000218495018, 9.999999999999998224, 17.49999999999999645 ) ) ;
#3840=CARTESIAN_POINT ( 'NONE',  ( 68.00000000109247367, 10.85617417291294551, 17.06698729999999742 ) ) ;
#3849=CARTESIAN_POINT ( 'NONE',  ( -70.60000000109246798, 7.933012699999995476, 15.85617417291294196 ) ) ;
#3852=CARTESIAN_POINT ( 'NONE',  ( -69.75000000109245946, 11.46158073645647235, 16.46158073645647235 ) ) ;
#3858=CARTESIAN_POINT ( 'NONE',  ( 71.09999999999999432, 7.499999999999996447, 14.99999999999999645 ) ) ;
#3860=CARTESIAN_POINT ( 'NONE',  ( -70.90000000109246514, 10.85617417291294551, 12.93301269999999370 ) ) ;
#3862=CARTESIAN_POINT ( 'NONE',  ( -71.40000000109246514, 10.85617417291294551, 17.06698729999999742 ) ) ;
#3873=CARTESIAN_POINT ( 'NONE',  ( -71.60000000218494165, 12.50000000000000000, 14.99999999999999645 ) ) ;
#3886=CARTESIAN_POINT ( 'NONE',  ( 68.95000000000000284, 11.03553390593273598, 12.49999999999999289 ) ) ;
#3888=CARTESIAN_POINT ( 'NONE',  ( -66.99999999999998579, 8.232233047033627571, 16.76776695296636532 ) ) ;
#3893=CARTESIAN_POINT ( 'NONE',  ( -71.45000000109247651, 9.999999999999998224, 17.06698730000000097 ) ) ;
#3895=CARTESIAN_POINT ( 'NONE',  ( 71.29999999999998295, 9.999999999999998224, 12.49999999999999289 ) ) ;
#3898=( BOUNDED_CURVE ( )  B_SPLINE_CURVE ( 2, ( #6743, #21682, #1212, #12512, #1570, #10832, #21202, #17993, #19772, #6856, #5293, #15856, #14181, #5054, #10716, #14419, #4816, #1447, #8784, #16203, #7102, #1095, #16089, #8441, #23376, #12148, #6979, #21558, #130, #3849, #1686, #23614, #18221, #18345, #11184, #5644, #7577, #7228, #21914, #12978, #16668, #14896, #16790, #22153, #3603, #13211, #10942, #1804, #242, #9491, #14544, #11059, #9030, #18458, #15020, #4082, #12749, #9151, #19, #22274, #5887, #5412, #16437, #20001, #18106, #3717, #5772, #7352, #20480, #14657, #13099, #12858, #2154, #18573, #5524, #21810, #20242, #16323, #3963, #370, #2039, #20114, #16554, #20355, #11299, #9377, #7703, #1925, #9267, #7459, #14775, #22027, #4206, #8058, #15372, #8172, #6244, #15605, #20598, #838, #10093, #6126, #13330, #11547, #13455, #18695, #2285, #603, #17271, #4562, #9849, #11662, #18816, #22640, #13564, #9980, #11898, #9623, #15485, #22395, #9733, #20833, #20717, #16914, #17147, #2636, #4441, #13681, #18930 ),
 .UNSPECIFIED., .F., .F. ) 
 B_SPLINE_CURVE_WITH_KNOTS ( ( 3, 2, 2, 2, 2, 2, 2, 2, 2, 2, 2, 2, 2, 2, 2, 2, 2, 2, 2, 2, 2, 2, 2, 2, 2, 2, 2, 2, 2, 2, 2, 2, 2, 2, 2, 2, 2, 2, 2, 2, 2, 2, 2, 2, 2, 2, 2, 2, 2, 2, 2, 2, 2, 2, 2, 2, 2, 2, 2, 2, 2, 2, 2, 2, 3 ),
 ( 0.000000000000000000, 0.01562500000000000000, 0.03125000000000000000, 0.04687500000000000000, 0.06250000000000000000, 0.07812500000000000000, 0.09375000000000000000, 0.1093750000000000000, 0.1250000000000000000, 0.1406250000000000000, 0.1562500000000000000, 0.1718750000000000000, 0.1875000000000000000, 0.2031250000000000000, 0.2187500000000000000, 0.2343750000000000000, 0.2500000000000000000, 0.2656250000000000000, 0.2812500000000000000, 0.2968750000000000000, 0.3125000000000000000, 0.3281250000000000000, 0.3437500000000000000, 0.3593750000000000000, 0.3750000000000000000, 0.3906250000000000000, 0.4062500000000000000, 0.4218750000000000000, 0.4375000000000000000, 0.4531250000000000000, 0.4687500000000000000, 0.4843750000000000000, 0.5000000000000000000, 0.5156250000000000000, 0.5312500000000000000, 0.5468750000000000000, 0.5625000000000000000, 0.5781250000000000000, 0.5937500000000000000, 0.6093750000000000000, 0.6250000000000000000, 0.6406250000000000000, 0.6562500000000000000, 0.6718750000000000000, 0.6875000000000000000, 0.7031250000000000000, 0.7187500000000000000, 0.7343750000000000000, 0.7500000000000000000, 0.7656250000000000000, 0.7812500000000000000, 0.7968750000000000000, 0.8125000000000000000, 0.8281250000000000000, 0.8437500000000000000, 0.8593750000000000000, 0.8750000000000000000, 0.8906250000000000000, 0.9062500000000000000, 0.9218750000000000000, 0.9375000000000000000, 0.9531250000000000000, 0.9687500000000000000, 0.9843750000000000000, 1.000000000000000000 ),
 .UNSPECIFIED. ) 
 CURVE ( )  GEOMETRIC_REPRESENTATION_ITEM ( )  RATIONAL_B_SPLINE_CURVE ( ( 1.000000000000000000, 0.9238795325112867385, 1.000000000000000000, 0.9238795325112867385, 1.000000000000000000, 0.9238795325112867385, 1.000000000000000000, 0.9238795325112867385, 1.000000000000000000, 0.9238795325112867385, 1.000000000000000000, 0.9238795325112867385, 1.000000000000000000, 0.9238795325112867385, 1.000000000000000000, 0.9238795325112867385, 1.000000000000000000, 0.9238795325112867385, 1.000000000000000000, 0.9238795325112867385, 1.000000000000000000, 0.9238795325112867385, 1.000000000000000000, 0.9238795325112867385, 1.000000000000000000, 0.9238795325112867385, 1.000000000000000000, 0.9238795325112867385, 1.000000000000000000, 0.9238795325112867385, 1.000000000000000000, 0.9238795325112867385, 1.000000000000000000, 0.9238795325112867385, 1.000000000000000000, 0.9238795325112867385, 1.000000000000000000, 0.9238795325112867385, 1.000000000000000000, 0.9238795325112867385, 1.000000000000000000, 0.9238795325112867385, 1.000000000000000000, 0.9238795325112867385, 1.000000000000000000, 0.9238795325112867385, 1.000000000000000000, 0.9238795325112867385, 1.000000000000000000, 0.9238795325112867385, 1.000000000000000000, 0.9238795325112867385, 1.000000000000000000, 0.9238795325112867385, 1.000000000000000000, 0.9238795325112867385, 1.000000000000000000, 0.9238795325112867385, 1.000000000000000000, 0.9238795325112867385, 1.000000000000000000, 0.9238795325112867385, 1.000000000000000000, 0.9238795325112867385, 1.000000000000000000, 0.9238795325112867385, 1.000000000000000000, 0.9238795325112867385, 1.000000000000000000, 0.9238795325112867385, 1.000000000000000000, 0.9238795325112867385, 1.000000000000000000, 0.9238795325112867385, 1.000000000000000000, 0.9238795325112867385, 1.000000000000000000, 0.9238795325112867385, 1.000000000000000000, 0.9238795325112867385, 1.000000000000000000, 0.9238795325112867385, 1.000000000000000000, 0.9238795325112867385, 1.000000000000000000, 0.9238795325112867385, 1.000000000000000000, 0.9238795325112867385, 1.000000000000000000, 0.9238795325112867385, 1.000000000000000000, 0.9238795325112867385, 1.000000000000000000, 0.9238795325112867385, 1.000000000000000000, 0.9238795325112867385, 1.000000000000000000, 0.9238795325112867385, 1.000000000000000000, 0.9238795325112867385, 1.000000000000000000, 0.9238795325112867385, 1.000000000000000000, 0.9238795325112867385, 1.000000000000000000, 0.9238795325112867385, 1.000000000000000000, 0.9238795325112867385, 1.000000000000000000, 0.9238795325112867385, 1.000000000000000000, 0.9238795325112867385, 1.000000000000000000, 0.9238795325112867385, 1.000000000000000000, 0.9238795325112867385, 1.000000000000000000, 0.9238795325112867385, 1.000000000000000000, 0.9238795325112867385, 1.000000000000000000, 0.9238795325112867385, 1.000000000000000000, 0.9238795325112867385, 1.000000000000000000, 0.9238795325112867385, 1.000000000000000000, 0.9238795325112867385, 1.000000000000000000 ) ) 
 REPRESENTATION_ITEM ( '' )  );
#3901=ORIENTED_EDGE ( 'NONE', *, *, #16314, .T. ) ;
#3903=EDGE_CURVE ( 'NONE', #14683, #18117, #17096, .T. ) ;
#3909=CARTESIAN_POINT ( 'NONE',  ( 66.10000000218495586, 11.76776695296636888, 16.76776695296636532 ) ) ;
#3911=CARTESIAN_POINT ( 'NONE',  ( 71.75000000109247367, 8.538419263543524096, 13.53841926354352054 ) ) ;
#3916=DIRECTION ( 'NONE',  ( 1.000000000000000000, 0.000000000000000000, 0.000000000000000000 ) ) ;
#3930=CARTESIAN_POINT ( 'NONE',  ( 70.70000000000000284, 12.50000000000000000, 14.99999999999999645 ) ) ;
#3939=( BOUNDED_CURVE ( )  B_SPLINE_CURVE ( 2, ( #5287, #14653, #12631, #10712, #20110, #16319, #17867, #23609, #11054 ),
 .UNSPECIFIED., .F., .F. ) 
 B_SPLINE_CURVE_WITH_KNOTS ( ( 3, 2, 2, 2, 3 ),
 ( 0.4999999999999991118, 0.5156249999999995559, 0.5312500000000000000, 0.5468750000000004441, 0.5625000000000008882 ),
 .UNSPECIFIED. ) 
 CURVE ( )  GEOMETRIC_REPRESENTATION_ITEM ( )  RATIONAL_B_SPLINE_CURVE ( ( 1.000000000000004219, 0.9238795325112824086, 1.000000000000000000, 0.9238795325112867385, 1.000000000000000000, 0.9238795325112867385, 1.000000000000000000, 0.9238795325112824086, 1.000000000000004219 ) ) 
 REPRESENTATION_ITEM ( '' )  );
#3945=PRESENTATION_STYLE_ASSIGNMENT (( #22624 ) ) ;
#3946=CARTESIAN_POINT ( 'NONE',  ( 70.35000000109246798, 11.46158073645647235, 13.53841926354352232 ) ) ;
#3951=ADVANCED_FACE ( 'NONE', ( #8608 ), #8099, .T. ) ;
#3952=CARTESIAN_POINT ( 'NONE',  ( 66.25000000218494733, 8.964466094067207180, 17.49999999999995026 ) ) ;
#3953=CARTESIAN_POINT ( 'NONE',  ( 67.15000000109247935, 11.46158073645647235, 16.46158073645647235 ) ) ;
#3963=CARTESIAN_POINT ( 'NONE',  ( -68.15000000109247935, 8.538419263543522320, 16.46158073645647235 ) ) ;
#3966=CARTESIAN_POINT ( 'NONE',  ( -70.15000000109246514, 8.538419263543524096, 13.53841926354352054 ) ) ;
#3969=ORIENTED_EDGE ( 'NONE', *, *, #14033, .T. ) ;
#3976=CARTESIAN_POINT ( 'NONE',  ( -67.55000000109247082, 8.538419263543524096, 13.53841926354352054 ) ) ;
#3977=CARTESIAN_POINT ( 'NONE',  ( 69.15000000109247935, 8.538419263543524096, 13.53841926354352054 ) ) ;
#3978=CARTESIAN_POINT ( 'NONE',  ( -68.65000000109246514, 9.999999999999998224, 12.93301269999999192 ) ) ;
#3987=CARTESIAN_POINT ( 'NONE',  ( 68.49999999999998579, 9.999999999999998224, 17.49999999999999645 ) ) ;
#3999=ADVANCED_FACE ( 'NONE', ( #11019 ), #16516, .T. ) ;
#4004=VERTEX_POINT ( 'NONE', #16628 ) ;
#4005=CARTESIAN_POINT ( 'NONE',  ( 72.50000000000000000, 9.999999999999998224, 14.99999999999999645 ) ) ;
#4007=CARTESIAN_POINT ( 'NONE',  ( 68.39999999999999147, 11.76776695296636888, 16.76776695296636532 ) ) ;
#4015=CARTESIAN_POINT ( 'NONE',  ( -72.09999999999999432, 9.999999999999998224, 12.49999999999999289 ) ) ;
#4022=CARTESIAN_POINT ( 'NONE',  ( -69.05000000109247082, 7.933012699999995476, 14.99999999999999645 ) ) ;
#4033=CARTESIAN_POINT ( 'NONE',  ( 65.45000000218496439, 8.964466094067258695, 17.50000000000000355 ) ) ;
#4036=CARTESIAN_POINT ( 'NONE',  ( 71.90000000109246514, 10.85617417291294551, 12.93301269999999370 ) ) ;
#4037=VERTEX_POINT ( 'NONE', #9582 ) ;
#4042=( BOUNDED_CURVE ( )  B_SPLINE_CURVE ( 2, ( #14813, #18033, #18379, #10977, #9414, #10758, #14694, #16588, #21952 ),
 .UNSPECIFIED., .F., .F. ) 
 B_SPLINE_CURVE_WITH_KNOTS ( ( 3, 2, 2, 2, 3 ),
 ( 0.4999999999999991118, 0.5156249999999995559, 0.5312500000000000000, 0.5468750000000004441, 0.5625000000000008882 ),
 .UNSPECIFIED. ) 
 CURVE ( )  GEOMETRIC_REPRESENTATION_ITEM ( )  RATIONAL_B_SPLINE_CURVE ( ( 1.000000000000004219, 0.9238795325112824086, 1.000000000000000000, 0.9238795325112867385, 1.000000000000000000, 0.9238795325112867385, 1.000000000000000000, 0.9238795325112824086, 1.000000000000004219 ) ) 
 REPRESENTATION_ITEM ( '' )  );
#4054=DIRECTION ( 'NONE',  ( 0.5000000000000013323, -0.000000000000000000, -0.8660254037844380415 ) ) ;
#4068=CARTESIAN_POINT ( 'NONE',  ( 70.40000000109247935, 12.06698729999999919, 14.14382582708705094 ) ) ;
#4073=CARTESIAN_POINT ( 'NONE',  ( 71.60000000109246798, 7.933012699999995476, 15.85617417291294196 ) ) ;
#4078=CARTESIAN_POINT ( 'NONE',  ( -71.05000000218497291, 8.964466094067221391, 17.49999999999996447 ) ) ;
#4082=CARTESIAN_POINT ( 'NONE',  ( -69.30000000109247082, 10.85617417291294551, 12.93301269999999192 ) ) ;
#4085=CARTESIAN_POINT ( 'NONE',  ( -65.80000000109247082, 7.933012699999995476, 15.85617417291294196 ) ) ;
#4086=VERTEX_POINT ( 'NONE', #13061 ) ;
#4094=CARTESIAN_POINT ( 'NONE',  ( -67.05000000109247082, 12.06698730000000097, 14.99999999999999645 ) ) ;
#4096=CARTESIAN_POINT ( 'NONE',  ( 68.35000000109248219, 8.538419263543524096, 13.53841926354352054 ) ) ;
#4098=CARTESIAN_POINT ( 'NONE',  ( -66.80000000109247082, 7.933012699999995476, 15.85617417291294196 ) ) ;
#4115=CARTESIAN_POINT ( 'NONE',  ( -71.00000000218494733, 9.999999999999998224, 17.49999999999999645 ) ) ;
#4121=CARTESIAN_POINT ( 'NONE',  ( -71.80000000218494449, 9.999999999999998224, 17.49999999999999645 ) ) ;
#4127=CARTESIAN_POINT ( 'NONE',  ( 66.90000000000000568, 9.999999999999998224, 17.49999999999999645 ) ) ;
#4129=CARTESIAN_POINT ( 'NONE',  ( -71.00000000000000000, 8.232233047033627571, 16.76776695296636532 ) ) ;
#4135=CARTESIAN_POINT ( 'NONE',  ( 68.85000000218495586, 7.499999999999996447, 13.96446609406725514 ) ) ;
#4142=CARTESIAN_POINT ( 'NONE',  ( -71.75000000109248788, 11.46158073645647235, 13.53841926354352232 ) ) ;
#4144=ORIENTED_EDGE ( 'NONE', *, *, #4298, .T. ) ;
#4150=EDGE_LOOP ( 'NONE', ( #1952, #17659, #7793, #22786 ) ) ;
#4152=CARTESIAN_POINT ( 'NONE',  ( 66.05000000218494449, 12.50000000000000000, 16.03553390593273420 ) ) ;
#4156=CARTESIAN_POINT ( 'NONE',  ( 71.70000000109247651, 7.933012699999995476, 14.14382582708705094 ) ) ;
#4165=CARTESIAN_POINT ( 'NONE',  ( -66.70000000109246230, 9.143825827087049163, 17.06698730000000097 ) ) ;
#4189=CARTESIAN_POINT ( 'NONE',  ( 72.10000000109246798, 12.06698729999999919, 15.85617417291294196 ) ) ;
#4195=CARTESIAN_POINT ( 'NONE',  ( 66.05000000109247082, 9.999999999999998224, 12.93301269999999192 ) ) ;
#4204=ORIENTED_EDGE ( 'NONE', *, *, #445, .T. ) ;
#4205=EDGE_CURVE ( 'NONE', #4668, #13655, #21195, .T. ) ;
#4206=CARTESIAN_POINT ( 'NONE',  ( -67.45000000109246230, 7.933012699999995476, 14.99999999999999645 ) ) ;
#4209=CARTESIAN_POINT ( 'NONE',  ( -70.55000000109245661, 11.46158073645647235, 16.46158073645647235 ) ) ;
#4212=CARTESIAN_POINT ( 'NONE',  ( 65.75000000109245946, 9.999999999999998224, 17.06698730000000097 ) ) ;
#4221=CARTESIAN_POINT ( 'NONE',  ( -67.45000000109246230, 7.933012699999995476, 14.99999999999999645 ) ) ;
#4223=CARTESIAN_POINT ( 'NONE',  ( 69.30000000109247082, 10.85617417291294551, 12.93301269999999192 ) ) ;
#4224=CARTESIAN_POINT ( 'NONE',  ( -72.50000000000000000, 9.999999999999998224, 17.49999999999999645 ) ) ;
#4234=ADVANCED_FACE ( 'NONE', ( #16990 ), #6206, .T. ) ;
#4247=VERTEX_POINT ( 'NONE', #4399 ) ;
#4250=CARTESIAN_POINT ( 'NONE',  ( -70.05000000218494449, 12.50000000000000000, 16.03553390593273420 ) ) ;
#4260=CARTESIAN_POINT ( 'NONE',  ( -71.89999999999999147, 7.499999999999996447, 14.99999999999999645 ) ) ;
#4261=CARTESIAN_POINT ( 'NONE',  ( -72.15000000109246514, 11.46158073645647235, 16.46158073645647235 ) ) ;
#4265=DIRECTION ( 'NONE',  ( -1.000000000000000000, -0.000000000000000000, -0.000000000000000000 ) ) ;
#4267=CARTESIAN_POINT ( 'NONE',  ( -69.85000000109248219, 7.933012699999995476, 14.99999999999999645 ) ) ;
#4276=CARTESIAN_POINT ( 'NONE',  ( 68.95000000109247651, 8.538419263543522320, 16.46158073645647235 ) ) ;
#4279=CARTESIAN_POINT ( 'NONE',  ( 71.10000000109246798, 10.85617417291294551, 12.93301269999999370 ) ) ;
#4289=DIRECTION ( 'NONE',  ( -1.000000000000000000, -0.000000000000000000, -0.000000000000000000 ) ) ;
#4294=CARTESIAN_POINT ( 'NONE',  ( 69.00000000218494733, 9.999999999999998224, 12.49999999999999289 ) ) ;
#4298=EDGE_CURVE ( 'NONE', #4468, #19953, #15038, .T. ) ;
#4301=DIRECTION ( 'NONE',  ( 0.000000000000000000, 0.000000000000000000, 1.000000000000000000 ) ) ;
#4303=CARTESIAN_POINT ( 'NONE',  ( 71.25000000109248788, 9.999999999999998224, 17.06698730000000097 ) ) ;
#4308=CARTESIAN_POINT ( 'NONE',  ( 70.85000000109246798, 7.933012699999995476, 14.99999999999999645 ) ) ;
#4312=CARTESIAN_POINT ( 'NONE',  ( 68.60000000109246798, 9.143825827087050939, 12.93301269999999370 ) ) ;
#4320=EDGE_LOOP ( 'NONE', ( #18287, #12181, #1445, #1390 ) ) ;
#4322=ORIENTED_EDGE ( 'NONE', *, *, #2574, .F. ) ;
#4324=CARTESIAN_POINT ( 'NONE',  ( -67.25000000109245946, 12.06698730000000097, 14.99999999999999645 ) ) ;
#4329=ORIENTED_EDGE ( 'NONE', *, *, #21331, .T. ) ;
#4332=CARTESIAN_POINT ( 'NONE',  ( -66.25000000109247367, 12.06698730000000097, 14.99999999999999645 ) ) ;
#4334=CARTESIAN_POINT ( 'NONE',  ( 70.65000000109247935, 7.933012699999995476, 14.99999999999999645 ) ) ;
#4336=CARTESIAN_POINT ( 'NONE',  ( -66.15000000109247935, 8.538419263543524096, 13.53841926354352054 ) ) ;
#4359=CARTESIAN_POINT ( 'NONE',  ( -71.75000000218496155, 11.03553390593273598, 17.50000000000000355 ) ) ;
#4366=CARTESIAN_POINT ( 'NONE',  ( 70.60000000109246798, 7.933012699999995476, 15.85617417291294196 ) ) ;
#4380=CARTESIAN_POINT ( 'NONE',  ( -72.05000000109247082, 9.999999999999998224, 17.06698730000000097 ) ) ;
#4385=ORIENTED_EDGE ( 'NONE', *, *, #8180, .T. ) ;
#4388=CARTESIAN_POINT ( 'NONE',  ( 67.50000000109247367, 7.933012699999995476, 14.14382582708705094 ) ) ;
#4391=CARTESIAN_POINT ( 'NONE',  ( 67.30000000109247082, 12.06698730000000275, 15.85617417291294196 ) ) ;
#4392=EDGE_CURVE ( 'NONE', #21422, #18582, #7946, .T. ) ;
#4394=ORIENTED_EDGE ( 'NONE', *, *, #21186, .T. ) ;
#4398=EDGE_CURVE ( 'NONE', #20854, #5860, #858, .T. ) ;
#4399=CARTESIAN_POINT ( 'NONE',  ( 65.65000000109247935, 9.999999999999998224, 17.06698730000000097 ) ) ;
#4406=CARTESIAN_POINT ( 'NONE',  ( -70.64999999999999147, 12.50000000000000000, 13.96446609406725692 ) ) ;
#4423=CARTESIAN_POINT ( 'NONE',  ( 69.90000000109246514, 9.143825827087049163, 17.06698730000000097 ) ) ;
#4430=CARTESIAN_POINT ( 'NONE',  ( 71.50000000109247367, 9.143825827087049163, 17.06698729999999742 ) ) ;
#4441=CARTESIAN_POINT ( 'NONE',  ( -65.75000000109247367, 8.538419263543522320, 16.46158073645647235 ) ) ;
#4443=CARTESIAN_POINT ( 'NONE',  ( -67.95000000109247651, 11.46158073645647235, 13.53841926354352232 ) ) ;
#4451=CARTESIAN_POINT ( 'NONE',  ( -66.80000000109247082, 9.143825827087050939, 12.93301269999999370 ) ) ;
#4452=CARTESIAN_POINT ( 'NONE',  ( 68.60000000109248219, 12.06698729999999919, 14.14382582708705094 ) ) ;
#4453=CARTESIAN_POINT ( 'NONE',  ( -66.25000000109245946, 9.999999999999998224, 12.93301269999999192 ) ) ;
#4456=DIRECTION ( 'NONE',  ( 0.000000000000000000, 0.000000000000000000, 1.000000000000000000 ) ) ;
#4468=VERTEX_POINT ( 'NONE', #17754 ) ;
#4474=CARTESIAN_POINT ( 'NONE',  ( -69.85000000218495586, 11.03553390593273598, 12.49999999999999289 ) ) ;
#4478=CARTESIAN_POINT ( 'NONE',  ( 66.49999999999998579, 9.999999999999998224, 12.49999999999999289 ) ) ;
#4479=CARTESIAN_POINT ( 'NONE',  ( -71.09999999999999432, 7.499999999999996447, 14.99999999999999645 ) ) ;
#4481=CARTESIAN_POINT ( 'NONE',  ( 70.25000000109247367, 12.06698730000000097, 14.99999999999999645 ) ) ;
#4487=CARTESIAN_POINT ( 'NONE',  ( 67.54999999999999716, 12.50000000000000000, 16.03553390593273775 ) ) ;
#4488=CARTESIAN_POINT ( 'NONE',  ( -68.20000000109246230, 10.85617417291294551, 17.06698730000000097 ) ) ;
#4489=CARTESIAN_POINT ( 'NONE',  ( -70.10000000218494165, 11.76776695296636888, 16.76776695296636532 ) ) ;
#4490=CARTESIAN_POINT ( 'NONE',  ( -69.79999999999999716, 11.76776695296636888, 13.23223304703362579 ) ) ;
#4500=ADVANCED_FACE ( 'NONE', ( #4812 ), #3007, .T. ) ;
#4506=UNCERTAINTY_MEASURE_WITH_UNIT (LENGTH_MEASURE( 1.000000000000000082E-05 ), #7670, 'distance_accuracy_value', 'NONE');
#4508=CARTESIAN_POINT ( 'NONE',  ( 67.00000000109247367, 12.06698730000000275, 14.14382582708705094 ) ) ;
#4510=CARTESIAN_POINT ( 'NONE',  ( 67.15000000109247935, 11.46158073645647235, 13.53841926354352232 ) ) ;
#4532=CARTESIAN_POINT ( 'NONE',  ( 71.35000000218497007, 8.964466094067278235, 12.49999999999997691 ) ) ;
#4534=CARTESIAN_POINT ( 'NONE',  ( -68.55000000218494449, 11.03553390593269157, 17.50000000000004619 ) ) ;
#4537=( BOUNDED_CURVE ( )  B_SPLINE_CURVE ( 2, ( #9111, #1536, #18306, #7189, #7316, #21768, #12718, #1888, #11146 ),
 .UNSPECIFIED., .F., .F. ) 
 B_SPLINE_CURVE_WITH_KNOTS ( ( 3, 2, 2, 2, 3 ),
 ( 0.6875000000000001110, 0.7031250000000000000, 0.7187500000000000000, 0.7343749999999998890, 0.7499999999999997780 ),
 .UNSPECIFIED. ) 
 CURVE ( )  GEOMETRIC_REPRESENTATION_ITEM ( )  RATIONAL_B_SPLINE_CURVE ( ( 0.9999999999999994449, 0.9238795325112872936, 1.000000000000000000, 0.9238795325112867385, 1.000000000000000000, 0.9238795325112867385, 1.000000000000000000, 0.9238795325112878487, 0.9999999999999988898 ) ) 
 REPRESENTATION_ITEM ( '' )  );
#4538=CARTESIAN_POINT ( 'NONE',  ( -69.75000000218496155, 8.964466094067244484, 12.50000000000000711 ) ) ;
#4540=CARTESIAN_POINT ( 'NONE',  ( 70.55000000218495870, 8.964466094067258695, 12.49999999999999289 ) ) ;
#4545=CARTESIAN_POINT ( 'NONE',  ( 68.55000000109247082, 8.538419263543524096, 13.53841926354352054 ) ) ;
#4547=CARTESIAN_POINT ( 'NONE',  ( -68.90000000218495302, 8.232233047033629347, 13.23223304703362402 ) ) ;
#4549=CARTESIAN_POINT ( 'NONE',  ( 69.70000000109246230, 12.06698730000000275, 15.85617417291294196 ) ) ;
#4562=CARTESIAN_POINT ( 'NONE',  ( -66.60000000109248219, 7.933012699999995476, 15.85617417291294196 ) ) ;
#4564=CARTESIAN_POINT ( 'NONE',  ( -67.10000000109246798, 10.85617417291294551, 12.93301269999999370 ) ) ;
#4579=CARTESIAN_POINT ( 'NONE',  ( -68.00000000109245946, 12.06698730000000275, 14.14382582708705094 ) ) ;
#4584=CARTESIAN_POINT ( 'NONE',  ( 72.50000000000000000, 9.999999999999998224, 17.49999999999999645 ) ) ;
#4596=AXIS2_PLACEMENT_3D ( 'NONE', #15071, #9787, #10041 ) ;
#4600=VERTEX_POINT ( 'NONE', #6975 ) ;
#4605=CARTESIAN_POINT ( 'NONE',  ( -71.45000000218495018, 11.03553390593273598, 12.49999999999999289 ) ) ;
#4606=CARTESIAN_POINT ( 'NONE',  ( -71.80000000218494449, 9.999999999999998224, 17.49999999999999645 ) ) ;
#4612=CARTESIAN_POINT ( 'NONE',  ( 70.35000000109248219, 11.46158073645647235, 16.46158073645647235 ) ) ;
#4619=CARTESIAN_POINT ( 'NONE',  ( -68.50000000109245946, 7.933012699999995476, 14.14382582708705094 ) ) ;
#4632=CARTESIAN_POINT ( 'NONE',  ( 69.45000000109247651, 12.06698730000000097, 14.99999999999999645 ) ) ;
#4633=CARTESIAN_POINT ( 'NONE',  ( 67.80000000109247082, 9.143825827087050939, 12.93301269999999370 ) ) ;
#4638=CARTESIAN_POINT ( 'NONE',  ( 71.60000000218494165, 12.50000000000000000, 14.99999999999999645 ) ) ;
#4640=DIRECTION ( 'NONE',  ( 0.000000000000000000, 0.000000000000000000, 1.000000000000000000 ) ) ;
#4645=CARTESIAN_POINT ( 'NONE',  ( 72.25000000109247367, 9.999999999999998224, 17.06698730000000097 ) ) ;
#4653=DIRECTION ( 'NONE',  ( -1.000000000000000000, -0.000000000000000000, -0.000000000000000000 ) ) ;
#4656=CARTESIAN_POINT ( 'NONE',  ( 70.05000000218494449, 12.50000000000000000, 16.03553390593273420 ) ) ;
#4659=CARTESIAN_POINT ( 'NONE',  ( 68.65000000109246514, 9.999999999999998224, 12.93301269999999192 ) ) ;
#4661=EDGE_CURVE ( 'NONE', #19572, #9951, #22893, .T. ) ;
#4662=CARTESIAN_POINT ( 'NONE',  ( -68.65000000218495302, 8.964466094067214286, 17.49999999999996092 ) ) ;
#4663=EDGE_CURVE ( 'NONE', #21869, #16726, #3939, .T. ) ;
#4665=CARTESIAN_POINT ( 'NONE',  ( 70.10000000109245377, 7.933012699999995476, 14.14382582708705094 ) ) ;
#4668=VERTEX_POINT ( 'NONE', #18341 ) ;
#4678=CARTESIAN_POINT ( 'NONE',  ( -66.40000000109247935, 12.06698730000000275, 14.14382582708705094 ) ) ;
#4679=( BOUNDED_CURVE ( )  B_SPLINE_CURVE ( 2, ( #11473, #15179, #22073, #22201, #13383, #20651, #3888, #11108, #9778 ),
 .UNSPECIFIED., .F., .F. ) 
 B_SPLINE_CURVE_WITH_KNOTS ( ( 3, 2, 2, 2, 3 ),
 ( 0.8124999999999993339, 0.8281249999999992228, 0.8437499999999991118, 0.8593749999999991118, 0.8749999999999990008 ),
 .UNSPECIFIED. ) 
 CURVE ( )  GEOMETRIC_REPRESENTATION_ITEM ( )  RATIONAL_B_SPLINE_CURVE ( ( 1.000000000000003331, 0.9238795325112835188, 1.000000000000000000, 0.9238795325112867385, 1.000000000000000000, 0.9238795325112867385, 1.000000000000000000, 0.9238795325112916235, 0.9999999999999951150 ) ) 
 REPRESENTATION_ITEM ( '' )  );
#4688=CARTESIAN_POINT ( 'NONE',  ( 66.45000000109247651, 9.999999999999998224, 17.06698730000000097 ) ) ;
#4690=CARTESIAN_POINT ( 'NONE',  ( -69.89999999999999147, 12.50000000000000000, 14.99999999999999645 ) ) ;
#4695=DIRECTION ( 'NONE',  ( 0.000000000000000000, 1.000000000000000000, 0.000000000000000000 ) ) ;
#4697=CARTESIAN_POINT ( 'NONE',  ( 67.30000000218494449, 8.232233047033629347, 13.23223304703362402 ) ) ;
#4698=CARTESIAN_POINT ( 'NONE',  ( 71.64999999999997726, 11.03553390593269867, 17.50000000000003908 ) ) ;
#4717=CARTESIAN_POINT ( 'NONE',  ( -68.80000000218494449, 7.499999999999996447, 14.99999999999999645 ) ) ;
#4723=CARTESIAN_POINT ( 'NONE',  ( 68.90000000109247935, 9.143825827087049163, 17.06698729999999742 ) ) ;
#4732=CARTESIAN_POINT ( 'NONE',  ( -68.30000000109247082, 9.143825827087049163, 17.06698730000000097 ) ) ;
#4736=CARTESIAN_POINT ( 'NONE',  ( 65.65000000218495302, 7.499999999999996447, 13.96446609406725514 ) ) ;
#4746=CARTESIAN_POINT ( 'NONE',  ( 66.85000000109248219, 9.999999999999998224, 12.93301269999999192 ) ) ;
#4747=CARTESIAN_POINT ( 'NONE',  ( 67.60000000109246798, 7.933012699999995476, 15.85617417291294196 ) ) ;
#4753=CARTESIAN_POINT ( 'NONE',  ( 68.05000000218494449, 7.499999999999996447, 13.96446609406725514 ) ) ;
#4760=VERTEX_POINT ( 'NONE', #9373 ) ;
#4762=CARTESIAN_POINT ( 'NONE',  ( 71.85000000109246798, 12.06698730000000097, 14.99999999999999645 ) ) ;
#4763=CARTESIAN_POINT ( 'NONE',  ( 71.05000000218497291, 8.964466094067221391, 17.49999999999996447 ) ) ;
#4767=EDGE_CURVE ( 'NONE', #7292, #20172, #8865, .T. ) ;
#4771=CARTESIAN_POINT ( 'NONE',  ( 70.35000000218492744, 7.499999999999995559, 16.03553390593273420 ) ) ;
#4774=CARTESIAN_POINT ( 'NONE',  ( 67.35000000109246798, 11.46158073645647235, 16.46158073645647235 ) ) ;
#4777=CARTESIAN_POINT ( 'NONE',  ( 70.75000000109247367, 8.538419263543522320, 16.46158073645647235 ) ) ;
#4785=AXIS2_PLACEMENT_3D ( 'NONE', #14114, #15905, #8368 ) ;
#4791=CARTESIAN_POINT ( 'NONE',  ( -68.35000000109246798, 8.538419263543522320, 16.46158073645647235 ) ) ;
#4794=CARTESIAN_POINT ( 'NONE',  ( -66.10000000218495586, 11.76776695296636888, 16.76776695296636532 ) ) ;
#4801=VECTOR ( 'NONE', #21071, 999.9999999999997726 ) ;
#4802=CARTESIAN_POINT ( 'NONE',  ( -68.05000000218494449, 7.499999999999996447, 13.96446609406725514 ) ) ;
#4804=EDGE_CURVE ( 'NONE', #18480, #22910, #11543, .T. ) ;
#4805=CARTESIAN_POINT ( 'NONE',  ( -69.54999999999999716, 7.499999999999995559, 13.96446609406725692 ) ) ;
#4806=CARTESIAN_POINT ( 'NONE',  ( -71.64999999999997726, 11.03553390593269867, 17.50000000000003908 ) ) ;
#4812=FACE_OUTER_BOUND ( 'NONE', #4150, .T. ) ;
#4816=CARTESIAN_POINT ( 'NONE',  ( -71.25000000109248788, 9.999999999999998224, 17.06698730000000097 ) ) ;
#4819=CARTESIAN_POINT ( 'NONE',  ( -69.30000000109247082, 10.85617417291294551, 12.93301269999999370 ) ) ;
#4829=CARTESIAN_POINT ( 'NONE',  ( -66.10000000218495586, 11.76776695296636888, 16.76776695296636532 ) ) ;
#4833=CARTESIAN_POINT ( 'NONE',  ( -71.70000000109247651, 7.933012699999995476, 14.14382582708705094 ) ) ;
#4837=CARTESIAN_POINT ( 'NONE',  ( 68.20000000109246230, 7.933012699999995476, 15.85617417291294196 ) ) ;
#4841=CARTESIAN_POINT ( 'NONE',  ( 67.55000000218494449, 12.50000000000000000, 13.96446609406725692 ) ) ;
#4843=CARTESIAN_POINT ( 'NONE',  ( -67.95000000109247651, 11.46158073645647235, 13.53841926354352232 ) ) ;
#4847=VERTEX_POINT ( 'NONE', #20828 ) ;
#4855=EDGE_CURVE ( 'NONE', #19246, #14210, #15827, .T. ) ;
#4861=CARTESIAN_POINT ( 'NONE',  ( 65.95000000109247651, 8.538419263543524096, 13.53841926354352054 ) ) ;
#4865=CARTESIAN_POINT ( 'NONE',  ( 68.05000000109247082, 12.06698730000000097, 14.99999999999999645 ) ) ;
#4871=FACE_OUTER_BOUND ( 'NONE', #9488, .T. ) ;
#4876=CARTESIAN_POINT ( 'NONE',  ( 68.09999999999999432, 9.999999999999998224, 12.49999999999999289 ) ) ;
#4882=CARTESIAN_POINT ( 'NONE',  ( -67.54999999999999716, 12.50000000000000000, 16.03553390593273775 ) ) ;
#4885=CARTESIAN_POINT ( 'NONE',  ( -68.35000000218495586, 12.50000000000000000, 13.96446609406725692 ) ) ;
#4891=CARTESIAN_POINT ( 'NONE',  ( 69.70000000218495018, 8.232233047033629347, 13.23223304703362402 ) ) ;
#4895=CARTESIAN_POINT ( 'NONE',  ( 66.50000000109245946, 12.06698729999999919, 15.85617417291294196 ) ) ;
#4898=AXIS2_PLACEMENT_3D ( 'NONE', #2786, #15520, #8204 ) ;
#4901=CARTESIAN_POINT ( 'NONE',  ( 68.30000000109247082, 9.143825827087049163, 17.06698729999999742 ) ) ;
#4903=CARTESIAN_POINT ( 'NONE',  ( -72.05000000109247082, 9.999999999999998224, 17.06698730000000097 ) ) ;
#4910=ORIENTED_EDGE ( 'NONE', *, *, #22388, .T. ) ;
#4922=CARTESIAN_POINT ( 'NONE',  ( -68.00000000218494733, 7.499999999999996447, 14.99999999999999645 ) ) ;
#4923=CARTESIAN_POINT ( 'NONE',  ( 67.40000000109247935, 7.933012699999995476, 15.85617417291294196 ) ) ;
#4927=CARTESIAN_POINT ( 'NONE',  ( -68.79999999999999716, 8.232233047033629347, 13.23223304703362402 ) ) ;
#4941=CARTESIAN_POINT ( 'NONE',  ( -68.50000000109247367, 10.85617417291294551, 12.93301269999999370 ) ) ;
#4942=AXIS2_PLACEMENT_3D ( 'NONE', #14621, #206, #9339 ) ;
#4951=EDGE_LOOP ( 'NONE', ( #21129, #15799, #1189, #3435 ) ) ;
#4954=CARTESIAN_POINT ( 'NONE',  ( -68.40000000218495302, 12.50000000000000000, 14.99999999999999645 ) ) ;
#4987=CYLINDRICAL_SURFACE ( 'NONE', #14059, 2.500000000000002220 ) ;
#4988=ORIENTED_EDGE ( 'NONE', *, *, #19938, .F. ) ;
#4989=CARTESIAN_POINT ( 'NONE',  ( 65.65000000109247935, 9.999999999999998224, 17.06698730000000097 ) ) ;
#4992=CARTESIAN_POINT ( 'NONE',  ( 66.50000000109245946, 12.06698730000000275, 15.85617417291294196 ) ) ;
#5009=CARTESIAN_POINT ( 'NONE',  ( 71.75000000109248788, 11.46158073645647235, 13.53841926354352232 ) ) ;
#5012=CARTESIAN_POINT ( 'NONE',  ( 66.10000000218495586, 11.76776695296636888, 16.76776695296636532 ) ) ;
#5015=CARTESIAN_POINT ( 'NONE',  ( 67.40000000218495302, 9.999999999999998224, 12.49999999999999289 ) ) ;
#5016=LINE ( 'NONE', #22852, #14549 ) ;
#5018=CARTESIAN_POINT ( 'NONE',  ( 67.10000000109246798, 10.85617417291294551, 12.93301269999999192 ) ) ;
#5023=CARTESIAN_POINT ( 'NONE',  ( 67.80000000109247082, 9.143825827087050939, 12.93301269999999370 ) ) ;
#5040=ORIENTED_EDGE ( 'NONE', *, *, #6266, .F. ) ;
#5045=CARTESIAN_POINT ( 'NONE',  ( -69.99999999999998579, 11.76776695296636888, 16.76776695296636532 ) ) ;
#5054=CARTESIAN_POINT ( 'NONE',  ( -71.40000000109249356, 7.933012699999995476, 15.85617417291294196 ) ) ;
#5057=CARTESIAN_POINT ( 'NONE',  ( -67.55000000109247082, 8.538419263543524096, 13.53841926354352054 ) ) ;
#5063=VECTOR ( 'NONE', #22963, 999.9999999999997726 ) ;
#5068=CARTESIAN_POINT ( 'NONE',  ( -67.55000000218494449, 12.50000000000000000, 13.96446609406725869 ) ) ;
#5098=VECTOR ( 'NONE', #5848, 1000.000000000000000 ) ;
#5099=CARTESIAN_POINT ( 'NONE',  ( 71.50000000000000000, 12.50000000000000000, 14.99999999999999645 ) ) ;
#5106=DIRECTION ( 'NONE',  ( 0.000000000000000000, 0.000000000000000000, 1.000000000000000000 ) ) ;
#5109=CARTESIAN_POINT ( 'NONE',  ( -70.60000000218494165, 9.999999999999998224, 12.49999999999999289 ) ) ;
#5116=CARTESIAN_POINT ( 'NONE',  ( 71.45000000109247651, 7.933012699999995476, 14.99999999999999645 ) ) ;
#5124=CARTESIAN_POINT ( 'NONE',  ( 68.00000000218494733, 7.499999999999996447, 14.99999999999999645 ) ) ;
#5134=CARTESIAN_POINT ( 'NONE',  ( 65.90000000109246514, 9.143825827087049163, 17.06698729999999742 ) ) ;
#5137=CARTESIAN_POINT ( 'NONE',  ( 68.89999999999999147, 9.999999999999998224, 12.49999999999999289 ) ) ;
#5145=CARTESIAN_POINT ( 'NONE',  ( -65.85000000109246798, 9.999999999999998224, 17.06698730000000097 ) ) ;
#5160=CARTESIAN_POINT ( 'NONE',  ( -70.74999999999998579, 12.50000000000000000, 16.03553390593273420 ) ) ;
#5165=CARTESIAN_POINT ( 'NONE',  ( 67.20000000218495018, 7.499999999999996447, 14.99999999999999645 ) ) ;
#5174=CARTESIAN_POINT ( 'NONE',  ( -67.50000000109247367, 7.933012699999995476, 14.14382582708705094 ) ) ;
#5180=DIRECTION ( 'NONE',  ( -0.5000000000000013323, 0.000000000000000000, -0.8660254037844380415 ) ) ;
#5183=CARTESIAN_POINT ( 'NONE',  ( -68.50000000218494733, 11.76776695296636888, 16.76776695296636532 ) ) ;
#5187=FACE_OUTER_BOUND ( 'NONE', #13595, .T. ) ;
#5215=CARTESIAN_POINT ( 'NONE',  ( 70.70000000000000284, 12.50000000000000000, 14.99999999999999645 ) ) ;
#5233=CARTESIAN_POINT ( 'NONE',  ( 67.29999999999999716, 9.999999999999998224, 12.49999999999999289 ) ) ;
#5235=CARTESIAN_POINT ( 'NONE',  ( -68.40000000218495302, 12.50000000000000000, 14.99999999999999645 ) ) ;
#5239=CARTESIAN_POINT ( 'NONE',  ( 67.65000000218496723, 12.50000000000000000, 16.03553390593273420 ) ) ;
#5242=CARTESIAN_POINT ( 'NONE',  ( -68.74999999999998579, 7.499999999999996447, 13.96446609406725514 ) ) ;
#5246=MECHANICAL_DESIGN_GEOMETRIC_PRESENTATION_REPRESENTATION('',(#2178),#23613);
#5250=CARTESIAN_POINT ( 'NONE',  ( 67.85000000109246798, 9.999999999999998224, 12.93301269999999192 ) ) ;
#5257=CARTESIAN_POINT ( 'NONE',  ( 72.50000000000000000, 9.999999999999998224, 14.99999999999999645 ) ) ;
#5263=VECTOR ( 'NONE', #10497, 1000.000000000000000 ) ;
#5265=CARTESIAN_POINT ( 'NONE',  ( -65.90000000109246514, 9.143825827087049163, 17.06698729999999742 ) ) ;
#5279=CARTESIAN_POINT ( 'NONE',  ( -67.04999999999999716, 7.499999999999995559, 16.03553390593273420 ) ) ;
#5285=CARTESIAN_POINT ( 'NONE',  ( -66.75000000109245946, 8.538419263543522320, 16.46158073645647235 ) ) ;
#5286=EDGE_CURVE ( 'NONE', #735, #19572, #23004, .T. ) ;
#5287=CARTESIAN_POINT ( 'NONE',  ( 68.60000000218495586, 9.999999999999998224, 17.49999999999999645 ) ) ;
#5293=CARTESIAN_POINT ( 'NONE',  ( -71.55000000109247082, 8.538419263543524096, 13.53841926354352054 ) ) ;
#5296=CARTESIAN_POINT ( 'NONE',  ( -66.60000000109248219, 7.933012699999995476, 15.85617417291294196 ) ) ;
#5307=CARTESIAN_POINT ( 'NONE',  ( -70.35000000109248219, 11.46158073645647235, 16.46158073645647235 ) ) ;
#5308=CARTESIAN_POINT ( 'NONE',  ( -69.10000000109246798, 9.143825827087049163, 17.06698729999999742 ) ) ;
#5313=CARTESIAN_POINT ( 'NONE',  ( 67.04999999999999716, 7.499999999999996447, 16.03553390593273775 ) ) ;
#5341=CARTESIAN_POINT ( 'NONE',  ( 70.50000000000000000, 9.999999999999998224, 12.49999999999999289 ) ) ;
#5352=CARTESIAN_POINT ( 'NONE',  ( 68.34999999999999432, 12.50000000000000000, 16.03553390593273775 ) ) ;
#5355=AXIS2_PLACEMENT_3D ( 'NONE', #22100, #2107, #20309 ) ;
#5361=DIRECTION ( 'NONE',  ( -1.000000000000000000, -0.000000000000000000, -0.000000000000000000 ) ) ;
#5365=CARTESIAN_POINT ( 'NONE',  ( 66.90000000218495302, 11.76776695296636888, 16.76776695296636532 ) ) ;
#5376=CARTESIAN_POINT ( 'NONE',  ( 66.65000000109247935, 9.999999999999998224, 17.06698730000000097 ) ) ;
#5378=CARTESIAN_POINT ( 'NONE',  ( -69.05000000000002558, 12.50000000000000000, 13.96446609406725692 ) ) ;
#5385=CARTESIAN_POINT ( 'NONE',  ( -72.25000000000000000, 12.50000000000000000, 13.96446609406725692 ) ) ;
#5389=DIRECTION ( 'NONE',  ( -1.000000000000000000, -0.000000000000000000, -0.000000000000000000 ) ) ;
#5398=CARTESIAN_POINT ( 'NONE',  ( -67.80000000218494449, 9.999999999999998224, 17.49999999999999645 ) ) ;
#5402=CARTESIAN_POINT ( 'NONE',  ( -66.49999999999998579, 9.999999999999998224, 12.49999999999999289 ) ) ;
#5412=CARTESIAN_POINT ( 'NONE',  ( -69.00000000109247367, 7.933012699999995476, 15.85617417291294196 ) ) ;
#5413=ORIENTED_EDGE ( 'NONE', *, *, #19192, .F. ) ;
#5415=CARTESIAN_POINT ( 'NONE',  ( -68.05000000109247082, 9.999999999999998224, 17.06698730000000097 ) ) ;
#5420=ORIENTED_EDGE ( 'NONE', *, *, #4804, .T. ) ;
#5424=CARTESIAN_POINT ( 'NONE',  ( -70.45000000109247651, 9.999999999999998224, 17.06698730000000097 ) ) ;
#5426=CARTESIAN_POINT ( 'NONE',  ( -69.85000000109246798, 9.999999999999998224, 17.06698730000000097 ) ) ;
#5428=CARTESIAN_POINT ( 'NONE',  ( 72.50000000000000000, 9.999999999999998224, 14.99999999999999645 ) ) ;
#5437=CARTESIAN_POINT ( 'NONE',  ( 69.80000000218494449, 9.999999999999998224, 12.49999999999999289 ) ) ;
#5439=EDGE_LOOP ( 'NONE', ( #22345, #22311, #2758, #21181 ) ) ;
#5443=AXIS2_PLACEMENT_3D ( 'NONE', #18536, #9458, #16756 ) ;
#5448=( BOUNDED_CURVE ( )  B_SPLINE_CURVE ( 2, ( #13425, #11745, #921, #2251, #19010, #20690, #7786, #22244, #4294 ),
 .UNSPECIFIED., .F., .F. ) 
 B_SPLINE_CURVE_WITH_KNOTS ( ( 3, 2, 2, 2, 3 ),
 ( 0.3749999999999998890, 0.3906249999999997780, 0.4062499999999996669, 0.4218749999999996114, 0.4374999999999995004 ),
 .UNSPECIFIED. ) 
 CURVE ( )  GEOMETRIC_REPRESENTATION_ITEM ( )  RATIONAL_B_SPLINE_CURVE ( ( 1.000000000000000444, 0.9238795325112861834, 1.000000000000000000, 0.9238795325112867385, 1.000000000000000000, 0.9238795325112867385, 1.000000000000000000, 0.9238795325112891810, 0.9999999999999975575 ) ) 
 REPRESENTATION_ITEM ( '' )  );
#5454=CARTESIAN_POINT ( 'NONE',  ( 70.14999999999999147, 8.964466094067258695, 17.50000000000000355 ) ) ;
#5458=CARTESIAN_POINT ( 'NONE',  ( 69.39999999999999147, 8.232233047033627571, 16.76776695296636532 ) ) ;
#5462=PLANE ( 'NONE',  #22364 ) ;
#5464=VERTEX_POINT ( 'NONE', #22329 ) ;
#5478=CARTESIAN_POINT ( 'NONE',  ( 67.80000000218494449, 9.999999999999998224, 17.49999999999999645 ) ) ;
#5479=( BOUNDED_SURFACE ( )  B_SPLINE_SURFACE ( 1, 2, ( 
 ( #4380, #22330, #17085, #11602, #18869, #11485, #4142, #18760, #16853, #2454, #13949, #15859, #18632, #2343, #431, #2218, #11358, #11717, #5944, #658, #9789, #7992, #9676, #16966, #543, #7756, #15314, #22586, #7867, #15189, #17655, #20535, #22449, #6062, #3014, #23133, #1215, #15073, #19418, #6189, #13510, #13395, #21205, #20662, #4267, #8121, #20774, #20413, #9559, #18983, #9915, #17212, #790, #15431, #23024, #4819, #6629, #12151, #10366, #6746, #4022, #21813, #10945, #1807, #12515, #14300, #23250, #10719, #19775, #21561, #1450, #4941, #12639, #1329, #12390, #8669, #22, #23379, #10835, #14053, #5415, #21685, #19543, #16092, #16326, #17761, #12752, #16206, #15967, #10603, #5057, #5174, #3379, #6859, #18109, #17877, #17996, #14547, #3138, #20004, #6982, #8787, #23492, #1573, #18224, #14184, #8911, #14422, #7105, #5296, #21444, #3606, #19655, #19898, #3500, #10480, #12277, #1689, #9154, #3256, #16440, #21321, #9033, #23617, #7231, #4085, #9380, #16793, #14660 ),
 ( #9626, #6008, #20117, #7817, #3720, #2288, #22156, #373, #7706, #245, #16917, #494, #20245, #18348, #18576, #15135, #14899, #15023, #22277, #7355, #1928, #18698, #9736, #5890, #21917, #13214, #2404, #22030, #11423, #20483, #14778, #22398, #13333, #20601, #4209, #11062, #11550, #9270, #5647, #18819, #17031, #16671, #3966, #16557, #5527, #12861, #133, #2157, #7462, #12981, #3852, #11187, #18461, #2042, #7580, #5775, #13102, #20358, #11302, #9494, #13684, #955, #21177, #22757, #13810, #17504, #19170, #20835, #10216, #2868, #6129, #11778, #18933, #2985, #9853, #20946, #21067, #2755, #4791, #2519, #6369, #13566, #15487, #840, #15252, #1073, #4443, #17150, #606, #728, #10339, #22519, #8289, #12127, #7932, #19391, #8061, #6489, #15375, #13458, #4324, #8174, #17273, #4564, #2638, #20720, #11900, #10095, #11665, #22642, #22875, #8415, #6246, #19047, #17386, #9982, #15608, #4678, #12012, #19277, #15728, #22998, #6604, #13922, #15939, #19628, #19868, #5265, #5145 ) ),
 .UNSPECIFIED., .F., .F., .F. ) 
 B_SPLINE_SURFACE_WITH_KNOTS ( ( 2, 2 ),
 ( 3, 2, 2, 2, 2, 2, 2, 2, 2, 2, 2, 2, 2, 2, 2, 2, 2, 2, 2, 2, 2, 2, 2, 2, 2, 2, 2, 2, 2, 2, 2, 2, 2, 2, 2, 2, 2, 2, 2, 2, 2, 2, 2, 2, 2, 2, 2, 2, 2, 2, 2, 2, 2, 2, 2, 2, 2, 2, 2, 2, 2, 2, 2, 2, 3 ),
 ( 0.000000000000000000, 1.000000000000000000 ),
 ( 0.000000000000000000, 0.01562500000000000000, 0.03125000000000000000, 0.04687500000000000000, 0.06250000000000000000, 0.07812500000000000000, 0.09375000000000000000, 0.1093750000000000000, 0.1250000000000000000, 0.1406250000000000000, 0.1562500000000000000, 0.1718750000000000000, 0.1875000000000000000, 0.2031250000000000000, 0.2187500000000000000, 0.2343750000000000000, 0.2500000000000000000, 0.2656250000000000000, 0.2812500000000000000, 0.2968750000000000000, 0.3125000000000000000, 0.3281250000000000000, 0.3437500000000000000, 0.3593750000000000000, 0.3750000000000000000, 0.3906250000000000000, 0.4062500000000000000, 0.4218750000000000000, 0.4375000000000000000, 0.4531250000000000000, 0.4687500000000000000, 0.4843750000000000000, 0.5000000000000000000, 0.5156250000000000000, 0.5312500000000000000, 0.5468750000000000000, 0.5625000000000000000, 0.5781250000000000000, 0.5937500000000000000, 0.6093750000000000000, 0.6250000000000000000, 0.6406250000000000000, 0.6562500000000000000, 0.6718750000000000000, 0.6875000000000000000, 0.7031250000000000000, 0.7187500000000000000, 0.7343750000000000000, 0.7500000000000000000, 0.7656250000000000000, 0.7812500000000000000, 0.7968750000000000000, 0.8125000000000000000, 0.8281250000000000000, 0.8437500000000000000, 0.8593750000000000000, 0.8750000000000000000, 0.8906250000000000000, 0.9062500000000000000, 0.9218750000000000000, 0.9375000000000000000, 0.9531250000000000000, 0.9687500000000000000, 0.9843750000000000000, 1.000000000000000000 ),
 .UNSPECIFIED. ) 
 GEOMETRIC_REPRESENTATION_ITEM ( )  RATIONAL_B_SPLINE_SURFACE ( (
 ( 1.000000000000000000, 0.9238795325112867385, 1.000000000000000000, 0.9238795325112867385, 1.000000000000000000, 0.9238795325112867385, 1.000000000000000000, 0.9238795325112867385, 1.000000000000000000, 0.9238795325112867385, 1.000000000000000000, 0.9238795325112867385, 1.000000000000000000, 0.9238795325112867385, 1.000000000000000000, 0.9238795325112867385, 1.000000000000000000, 0.9238795325112867385, 1.000000000000000000, 0.9238795325112867385, 1.000000000000000000, 0.9238795325112867385, 1.000000000000000000, 0.9238795325112867385, 1.000000000000000000, 0.9238795325112867385, 1.000000000000000000, 0.9238795325112867385, 1.000000000000000000, 0.9238795325112867385, 1.000000000000000000, 0.9238795325112867385, 1.000000000000000000, 0.9238795325112867385, 1.000000000000000000, 0.9238795325112867385, 1.000000000000000000, 0.9238795325112867385, 1.000000000000000000, 0.9238795325112867385, 1.000000000000000000, 0.9238795325112867385, 1.000000000000000000, 0.9238795325112867385, 1.000000000000000000, 0.9238795325112867385, 1.000000000000000000, 0.9238795325112867385, 1.000000000000000000, 0.9238795325112867385, 1.000000000000000000, 0.9238795325112867385, 1.000000000000000000, 0.9238795325112867385, 1.000000000000000000, 0.9238795325112867385, 1.000000000000000000, 0.9238795325112867385, 1.000000000000000000, 0.9238795325112867385, 1.000000000000000000, 0.9238795325112867385, 1.000000000000000000, 0.9238795325112867385, 1.000000000000000000, 0.9238795325112867385, 1.000000000000000000, 0.9238795325112867385, 1.000000000000000000, 0.9238795325112867385, 1.000000000000000000, 0.9238795325112867385, 1.000000000000000000, 0.9238795325112867385, 1.000000000000000000, 0.9238795325112867385, 1.000000000000000000, 0.9238795325112867385, 1.000000000000000000, 0.9238795325112867385, 1.000000000000000000, 0.9238795325112867385, 1.000000000000000000, 0.9238795325112867385, 1.000000000000000000, 0.9238795325112867385, 1.000000000000000000, 0.9238795325112867385, 1.000000000000000000, 0.9238795325112867385, 1.000000000000000000, 0.9238795325112867385, 1.000000000000000000, 0.9238795325112867385, 1.000000000000000000, 0.9238795325112867385, 1.000000000000000000, 0.9238795325112867385, 1.000000000000000000, 0.9238795325112867385, 1.000000000000000000, 0.9238795325112867385, 1.000000000000000000, 0.9238795325112867385, 1.000000000000000000, 0.9238795325112867385, 1.000000000000000000, 0.9238795325112867385, 1.000000000000000000, 0.9238795325112867385, 1.000000000000000000, 0.9238795325112867385, 1.000000000000000000, 0.9238795325112867385, 1.000000000000000000, 0.9238795325112867385, 1.000000000000000000, 0.9238795325112867385, 1.000000000000000000, 0.9238795325112867385, 1.000000000000000000, 0.9238795325112867385, 1.000000000000000000, 0.9238795325112867385, 1.000000000000000000, 0.9238795325112867385, 1.000000000000000000, 0.9238795325112867385, 1.000000000000000000),
 ( 1.000000000000000000, 0.9238795325112867385, 1.000000000000000000, 0.9238795325112867385, 1.000000000000000000, 0.9238795325112867385, 1.000000000000000000, 0.9238795325112867385, 1.000000000000000000, 0.9238795325112867385, 1.000000000000000000, 0.9238795325112867385, 1.000000000000000000, 0.9238795325112867385, 1.000000000000000000, 0.9238795325112867385, 1.000000000000000000, 0.9238795325112867385, 1.000000000000000000, 0.9238795325112867385, 1.000000000000000000, 0.9238795325112867385, 1.000000000000000000, 0.9238795325112867385, 1.000000000000000000, 0.9238795325112867385, 1.000000000000000000, 0.9238795325112867385, 1.000000000000000000, 0.9238795325112867385, 1.000000000000000000, 0.9238795325112867385, 1.000000000000000000, 0.9238795325112867385, 1.000000000000000000, 0.9238795325112867385, 1.000000000000000000, 0.9238795325112867385, 1.000000000000000000, 0.9238795325112867385, 1.000000000000000000, 0.9238795325112867385, 1.000000000000000000, 0.9238795325112867385, 1.000000000000000000, 0.9238795325112867385, 1.000000000000000000, 0.9238795325112867385, 1.000000000000000000, 0.9238795325112867385, 1.000000000000000000, 0.9238795325112867385, 1.000000000000000000, 0.9238795325112867385, 1.000000000000000000, 0.9238795325112867385, 1.000000000000000000, 0.9238795325112867385, 1.000000000000000000, 0.9238795325112867385, 1.000000000000000000, 0.9238795325112867385, 1.000000000000000000, 0.9238795325112867385, 1.000000000000000000, 0.9238795325112867385, 1.000000000000000000, 0.9238795325112867385, 1.000000000000000000, 0.9238795325112867385, 1.000000000000000000, 0.9238795325112867385, 1.000000000000000000, 0.9238795325112867385, 1.000000000000000000, 0.9238795325112867385, 1.000000000000000000, 0.9238795325112867385, 1.000000000000000000, 0.9238795325112867385, 1.000000000000000000, 0.9238795325112867385, 1.000000000000000000, 0.9238795325112867385, 1.000000000000000000, 0.9238795325112867385, 1.000000000000000000, 0.9238795325112867385, 1.000000000000000000, 0.9238795325112867385, 1.000000000000000000, 0.9238795325112867385, 1.000000000000000000, 0.9238795325112867385, 1.000000000000000000, 0.9238795325112867385, 1.000000000000000000, 0.9238795325112867385, 1.000000000000000000, 0.9238795325112867385, 1.000000000000000000, 0.9238795325112867385, 1.000000000000000000, 0.9238795325112867385, 1.000000000000000000, 0.9238795325112867385, 1.000000000000000000, 0.9238795325112867385, 1.000000000000000000, 0.9238795325112867385, 1.000000000000000000, 0.9238795325112867385, 1.000000000000000000, 0.9238795325112867385, 1.000000000000000000, 0.9238795325112867385, 1.000000000000000000, 0.9238795325112867385, 1.000000000000000000, 0.9238795325112867385, 1.000000000000000000, 0.9238795325112867385, 1.000000000000000000, 0.9238795325112867385, 1.000000000000000000, 0.9238795325112867385, 1.000000000000000000, 0.9238795325112867385, 1.000000000000000000) ) ) 
 REPRESENTATION_ITEM ( '' )  SURFACE ( )  );
#5505=VERTEX_POINT ( 'NONE', #21860 ) ;
#5512=CARTESIAN_POINT ( 'NONE',  ( -68.34999999999999432, 12.50000000000000000, 16.03553390593273420 ) ) ;
#5514=CARTESIAN_POINT ( 'NONE',  ( 66.30000000109247082, 12.06698730000000275, 15.85617417291294196 ) ) ;
#5524=CARTESIAN_POINT ( 'NONE',  ( -68.35000000109248219, 8.538419263543524096, 13.53841926354352054 ) ) ;
#5527=CARTESIAN_POINT ( 'NONE',  ( -70.05000000109247082, 7.933012699999995476, 14.99999999999999645 ) ) ;
#5538=CARTESIAN_POINT ( 'NONE',  ( -69.30000000109247082, 10.85617417291294551, 12.93301269999999370 ) ) ;
#5539=CIRCLE ( 'NONE', #8616, 2.500000000000002220 ) ;
#5540=CARTESIAN_POINT ( 'NONE',  ( -69.20000000109246230, 7.933012699999995476, 15.85617417291294196 ) ) ;
#5544=CARTESIAN_POINT ( 'NONE',  ( 71.79999999999998295, 8.232233047033627571, 16.76776695296636532 ) ) ;
#5550=CARTESIAN_POINT ( 'NONE',  ( 69.90000000218495302, 11.76776695296636888, 13.23223304703362579 ) ) ;
#5552=DIRECTION ( 'NONE',  ( -1.000000000000000000, -0.000000000000000000, -0.000000000000000000 ) ) ;
#5567=ADVANCED_FACE ( 'NONE', ( #15072 ), #16965, .T. ) ;
#5571=CARTESIAN_POINT ( 'NONE',  ( 67.64999999999999147, 11.03553390593273598, 17.50000000000000355 ) ) ;
#5599=CARTESIAN_POINT ( 'NONE',  ( 71.45000000109247651, 7.933012699999995476, 14.99999999999999645 ) ) ;
#5601=CARTESIAN_POINT ( 'NONE',  ( 72.25000000109247367, 9.999999999999998224, 17.06698730000000097 ) ) ;
#5608=CARTESIAN_POINT ( 'NONE',  ( 66.85000000218495586, 12.50000000000000000, 16.03553390593273775 ) ) ;
#5609=CARTESIAN_POINT ( 'NONE',  ( 72.50000000000000000, 9.999999999999998224, 14.99999999999999645 ) ) ;
#5633=CARTESIAN_POINT ( 'NONE',  ( -66.34999999999999432, 7.499999999999995559, 13.96446609406725692 ) ) ;
#5635=CARTESIAN_POINT ( 'NONE',  ( 71.85000000109246798, 9.999999999999998224, 12.93301269999999192 ) ) ;
#5641=CARTESIAN_POINT ( 'NONE',  ( -67.35000000218495586, 8.964466094067256918, 12.49999999999999822 ) ) ;
#5644=CARTESIAN_POINT ( 'NONE',  ( -70.30000000109247082, 12.06698729999999919, 15.85617417291294196 ) ) ;
#5647=CARTESIAN_POINT ( 'NONE',  ( -70.35000000109246798, 11.46158073645647235, 13.53841926354352232 ) ) ;
#5655=CARTESIAN_POINT ( 'NONE',  ( -65.55000000218494449, 7.499999999999995559, 16.03553390593273420 ) ) ;
#5658=CARTESIAN_POINT ( 'NONE',  ( -71.10000000109246798, 10.85617417291294551, 12.93301269999999370 ) ) ;
#5668=CARTESIAN_POINT ( 'NONE',  ( 68.89999999999999147, 9.999999999999998224, 12.49999999999999289 ) ) ;
#5672=ORIENTED_EDGE ( 'NONE', *, *, #16360, .F. ) ;
#5681=ORIENTED_EDGE ( 'NONE', *, *, #15642, .T. ) ;
#5687=CARTESIAN_POINT ( 'NONE',  ( 68.79999999999999716, 8.232233047033629347, 13.23223304703362402 ) ) ;
#5697=CARTESIAN_POINT ( 'NONE',  ( -71.70000000000000284, 9.999999999999998224, 17.49999999999999645 ) ) ;
#5698=CARTESIAN_POINT ( 'NONE',  ( -71.70000000109247651, 7.933012699999995476, 14.14382582708705094 ) ) ;
#5707=ORIENTED_EDGE ( 'NONE', *, *, #12634, .T. ) ;
#5717=CARTESIAN_POINT ( 'NONE',  ( 71.10000000109246798, 12.06698730000000275, 15.85617417291294196 ) ) ;
#5721=CARTESIAN_POINT ( 'NONE',  ( 72.20000000109246230, 10.85617417291294551, 17.06698729999999742 ) ) ;
#5726=( BOUNDED_CURVE ( )  B_SPLINE_CURVE ( 2, ( #11984, #4532, #9824, #19252, #815, #17937, #14364, #4763, #16154 ),
 .UNSPECIFIED., .F., .F. ) 
 B_SPLINE_CURVE_WITH_KNOTS ( ( 3, 2, 2, 2, 3 ),
 ( 0.06249999999999961836, 0.07812499999999952816, 0.09374999999999943101, 0.1093749999999993339, 0.1249999999999992367 ),
 .UNSPECIFIED. ) 
 CURVE ( )  GEOMETRIC_REPRESENTATION_ITEM ( )  RATIONAL_B_SPLINE_CURVE ( ( 1.000000000000001776, 0.9238795325112848511, 1.000000000000000000, 0.9238795325112867385, 1.000000000000000000, 0.9238795325112867385, 1.000000000000000000, 0.9238795325112904022, 0.9999999999999963363 ) ) 
 REPRESENTATION_ITEM ( '' )  );
#5732=CARTESIAN_POINT ( 'NONE',  ( 72.34999999999999432, 12.50000000000000000, 16.03553390593273775 ) ) ;
#5733=EDGE_CURVE ( 'NONE', #7791, #1264, #20398, .T. ) ;
#5734=CARTESIAN_POINT ( 'NONE',  ( -67.05000000109247082, 9.999999999999998224, 12.93301269999999192 ) ) ;
#5739=FACE_OUTER_BOUND ( 'NONE', #17470, .T. ) ;
#5747=CARTESIAN_POINT ( 'NONE',  ( 69.95000000000001705, 12.50000000000000000, 16.03553390593273775 ) ) ;
#5753=SURFACE_SIDE_STYLE ('',( #13084 ) ) ;
#5754=CARTESIAN_POINT ( 'NONE',  ( 70.80000000109245661, 7.933012699999995476, 15.85617417291294196 ) ) ;
#5755=ORIENTED_EDGE ( 'NONE', *, *, #8429, .T. ) ;
#5758=CARTESIAN_POINT ( 'NONE',  ( -66.54999999999999716, 11.03553390593273598, 12.49999999999999289 ) ) ;
#5762=CARTESIAN_POINT ( 'NONE',  ( 67.75000000109247367, 11.46158073645647235, 13.53841926354352232 ) ) ;
#5772=CARTESIAN_POINT ( 'NONE',  ( -68.75000000109247367, 11.46158073645647235, 16.46158073645647235 ) ) ;
#5775=CARTESIAN_POINT ( 'NONE',  ( -69.50000000109247367, 10.85617417291294551, 12.93301269999999370 ) ) ;
#5782=CARTESIAN_POINT ( 'NONE',  ( -71.40000000109249356, 7.933012699999995476, 15.85617417291294196 ) ) ;
#5783=CARTESIAN_POINT ( 'NONE',  ( 69.65000000109247935, 9.999999999999998224, 17.06698730000000097 ) ) ;
#5784=CARTESIAN_POINT ( 'NONE',  ( -69.30000000109247082, 7.933012699999995476, 14.14382582708705094 ) ) ;
#5793=CARTESIAN_POINT ( 'NONE',  ( -69.25000000218494733, 12.50000000000000000, 16.03553390593273775 ) ) ;
#5795=CARTESIAN_POINT ( 'NONE',  ( 70.10000000218494165, 11.76776695296636888, 16.76776695296636532 ) ) ;
#5796=CARTESIAN_POINT ( 'NONE',  ( -70.45000000000000284, 8.964466094067244484, 12.50000000000000711 ) ) ;
#5810=CARTESIAN_POINT ( 'NONE',  ( 67.04999999999999716, 7.499999999999995559, 16.03553390593273420 ) ) ;
#5835=CARTESIAN_POINT ( 'NONE',  ( 65.95000000218495018, 12.50000000000000000, 13.96446609406725869 ) ) ;
#5836=CARTESIAN_POINT ( 'NONE',  ( 66.29999999999999716, 7.499999999999996447, 14.99999999999999645 ) ) ;
#5837=CARTESIAN_POINT ( 'NONE',  ( 70.20000000109246230, 9.143825827087050939, 12.93301269999999370 ) ) ;
#5848=DIRECTION ( 'NONE',  ( -1.000000000000000000, -0.000000000000000000, -0.000000000000000000 ) ) ;
#5860=VERTEX_POINT ( 'NONE', #20804 ) ;
#5870=DIRECTION ( 'NONE',  ( -1.000000000000000000, -0.000000000000000000, -0.000000000000000000 ) ) ;
#5871=CARTESIAN_POINT ( 'NONE',  ( 69.10000000109246798, 9.143825827087049163, 17.06698730000000097 ) ) ;
#5876=CARTESIAN_POINT ( 'NONE',  ( -72.50000000000000000, 9.999999999999998224, 14.99999999999999645 ) ) ;
#5877=CARTESIAN_POINT ( 'NONE',  ( 71.80000000109245661, 9.143825827087050939, 12.93301269999999370 ) ) ;
#5882=CARTESIAN_POINT ( 'NONE',  ( -71.15000000218496723, 7.499999999999996447, 16.03553390593273775 ) ) ;
#5887=CARTESIAN_POINT ( 'NONE',  ( -69.05000000109247082, 7.933012699999995476, 14.99999999999999645 ) ) ;
#5888=ORIENTED_EDGE ( 'NONE', *, *, #20061, .T. ) ;
#5890=CARTESIAN_POINT ( 'NONE',  ( -71.10000000109246798, 10.85617417291294551, 12.93301269999999370 ) ) ;
#5902=CARTESIAN_POINT ( 'NONE',  ( -68.55000000109247082, 11.46158073645647235, 13.53841926354352232 ) ) ;
#5903=CARTESIAN_POINT ( 'NONE',  ( 68.50000000109247367, 10.85617417291294551, 12.93301269999999192 ) ) ;
#5904=CARTESIAN_POINT ( 'NONE',  ( -68.30000000109247082, 9.143825827087049163, 17.06698729999999742 ) ) ;
#5905=DIRECTION ( 'NONE',  ( 0.000000000000000000, 0.000000000000000000, 1.000000000000000000 ) ) ;
#5911=CARTESIAN_POINT ( 'NONE',  ( -69.15000000218495302, 12.50000000000000000, 13.96446609406725692 ) ) ;
#5927=CARTESIAN_POINT ( 'NONE',  ( -69.05000000218494449, 11.03553390593273598, 12.49999999999999289 ) ) ;
#5929=CARTESIAN_POINT ( 'NONE',  ( 68.59999999999999432, 8.232233047033627571, 16.76776695296636532 ) ) ;
#5938=CARTESIAN_POINT ( 'NONE',  ( 68.75000000218494733, 7.499999999999996447, 16.03553390593273775 ) ) ;
#5939=CARTESIAN_POINT ( 'NONE',  ( -70.55000000109245661, 11.46158073645647235, 16.46158073645647235 ) ) ;
#5940=CARTESIAN_POINT ( 'NONE',  ( -69.95000000000001705, 12.50000000000000000, 16.03553390593273775 ) ) ;
#5944=CARTESIAN_POINT ( 'NONE',  ( -71.15000000109247935, 11.46158073645647235, 16.46158073645647235 ) ) ;
#5952=EDGE_LOOP ( 'NONE', ( #2482, #9297, #8377, #13464 ) ) ;
#5955=CARTESIAN_POINT ( 'NONE',  ( 71.15000000109247935, 11.46158073645647235, 16.46158073645647235 ) ) ;
#5957=CARTESIAN_POINT ( 'NONE',  ( 71.85000000109246798, 9.999999999999998224, 12.93301269999999192 ) ) ;
#5958=ORIENTED_EDGE ( 'NONE', *, *, #9461, .T. ) ;
#5972=CARTESIAN_POINT ( 'NONE',  ( -70.75000000000000000, 12.50000000000000000, 16.03553390593273775 ) ) ;
#5977=CARTESIAN_POINT ( 'NONE',  ( -70.85000000218494165, 12.50000000000000000, 16.03553390593273775 ) ) ;
#5987=CARTESIAN_POINT ( 'NONE',  ( 70.45000000109247651, 12.06698730000000097, 14.99999999999999645 ) ) ;
#5990=LINE ( 'NONE', #13551, #16425 ) ;
#5993=CARTESIAN_POINT ( 'NONE',  ( 66.15000000109247935, 11.46158073645647235, 13.53841926354352232 ) ) ;
#6008=CARTESIAN_POINT ( 'NONE',  ( -72.20000000109246230, 10.85617417291294551, 17.06698729999999742 ) ) ;
#6012=ORIENTED_EDGE ( 'NONE', *, *, #8298, .F. ) ;
#6017=CARTESIAN_POINT ( 'NONE',  ( -66.70000000109246230, 7.933012699999995476, 14.14382582708705094 ) ) ;
#6018=CARTESIAN_POINT ( 'NONE',  ( 69.05000000109247082, 7.933012699999995476, 14.99999999999999645 ) ) ;
#6019=CARTESIAN_POINT ( 'NONE',  ( -66.00000000109245946, 7.933012699999995476, 15.85617417291294196 ) ) ;
#6044=CARTESIAN_POINT ( 'NONE',  ( -70.00000000218494733, 12.50000000000000000, 14.99999999999999645 ) ) ;
#6049=CARTESIAN_POINT ( 'NONE',  ( 68.49999999999998579, 9.999999999999998224, 17.49999999999999645 ) ) ;
#6056=CARTESIAN_POINT ( 'NONE',  ( 68.80000000218494449, 7.499999999999996447, 14.99999999999999645 ) ) ;
#6057=CARTESIAN_POINT ( 'NONE',  ( -70.35000000109246798, 11.46158073645647235, 13.53841926354352232 ) ) ;
#6062=CARTESIAN_POINT ( 'NONE',  ( -70.40000000109250777, 10.85617417291294551, 17.06698729999999742 ) ) ;
#6071=CARTESIAN_POINT ( 'NONE',  ( 69.90000000109247935, 7.933012699999995476, 14.14382582708705094 ) ) ;
#6076=VERTEX_POINT ( 'NONE', #19597 ) ;
#6095=CARTESIAN_POINT ( 'NONE',  ( -70.65000000218495302, 11.03553390593268269, 12.49999999999994138 ) ) ;
#6097=LINE ( 'NONE', #8264, #19462 ) ;
#6101=CARTESIAN_POINT ( 'NONE',  ( 71.60000000109246798, 9.143825827087052716, 12.93301269999999192 ) ) ;
#6106=DIRECTION ( 'NONE',  ( -1.000000000000000000, -0.000000000000000000, -0.000000000000000000 ) ) ;
#6108=CARTESIAN_POINT ( 'NONE',  ( 69.40000000109246514, 9.143825827087052716, 12.93301269999999192 ) ) ;
#6115=CARTESIAN_POINT ( 'NONE',  ( 70.15000000109246514, 8.538419263543524096, 13.53841926354352054 ) ) ;
#6126=CARTESIAN_POINT ( 'NONE',  ( -67.00000000109247367, 12.06698729999999919, 14.14382582708705094 ) ) ;
#6129=CARTESIAN_POINT ( 'NONE',  ( -68.75000000109245946, 11.46158073645647235, 13.53841926354352232 ) ) ;
#6135=VECTOR ( 'NONE', #21460, 1000.000000000000000 ) ;
#6143=CARTESIAN_POINT ( 'NONE',  ( -66.60000000109248219, 7.933012699999995476, 15.85617417291294196 ) ) ;
#6145=CARTESIAN_POINT ( 'NONE',  ( 67.55000000109247082, 8.538419263543524096, 13.53841926354352054 ) ) ;
#6147=CARTESIAN_POINT ( 'NONE',  ( -66.65000000109247935, 9.999999999999998224, 17.06698730000000097 ) ) ;
#6164=ORIENTED_EDGE ( 'NONE', *, *, #15403, .F. ) ;
#6170=CARTESIAN_POINT ( 'NONE',  ( -69.75000000218496155, 8.964466094067258695, 12.49999999999999289 ) ) ;
#6176=CARTESIAN_POINT ( 'NONE',  ( 66.64999999999999147, 12.50000000000000000, 13.96446609406725869 ) ) ;
#6178=CARTESIAN_POINT ( 'NONE',  ( 68.70000000109246230, 12.06698730000000275, 15.85617417291294196 ) ) ;
#6184=CARTESIAN_POINT ( 'NONE',  ( -71.00000000109247367, 9.143825827087052716, 12.93301269999999192 ) ) ;
#6185=CARTESIAN_POINT ( 'NONE',  ( 65.55000000218494449, 7.499999999999996447, 16.03553390593273775 ) ) ;
#6189=CARTESIAN_POINT ( 'NONE',  ( -70.10000000109246798, 10.85617417291294551, 12.93301269999999370 ) ) ;
#6199=CARTESIAN_POINT ( 'NONE',  ( 67.60000000109248219, 9.143825827087050939, 12.93301269999999370 ) ) ;
#6201=CARTESIAN_POINT ( 'NONE',  ( 68.55000000109247082, 8.538419263543524096, 13.53841926354352054 ) ) ;
#6206=CYLINDRICAL_SURFACE ( 'NONE', #2838, 2.500000000000002220 ) ;
#6222=CARTESIAN_POINT ( 'NONE',  ( 70.90000000109247935, 10.85617417291294551, 12.93301269999999192 ) ) ;
#6223=( BOUNDED_CURVE ( )  B_SPLINE_CURVE ( 2, ( #12562, #23662, #16018, #12794, #7151, #12435, #5458, #21851, #10876 ),
 .UNSPECIFIED., .F., .F. ) 
 B_SPLINE_CURVE_WITH_KNOTS ( ( 3, 2, 2, 2, 3 ),
 ( 0.4374999999999995004, 0.4531249999999993894, 0.4687499999999993339, 0.4843749999999992228, 0.4999999999999991118 ),
 .UNSPECIFIED. ) 
 CURVE ( )  GEOMETRIC_REPRESENTATION_ITEM ( )  RATIONAL_B_SPLINE_CURVE ( ( 1.000000000000002442, 0.9238795325112842960, 1.000000000000000000, 0.9238795325112867385, 1.000000000000000000, 0.9238795325112867385, 1.000000000000000000, 0.9238795325112910684, 0.9999999999999956701 ) ) 
 REPRESENTATION_ITEM ( '' )  );
#6228=CARTESIAN_POINT ( 'NONE',  ( 71.05000000109245661, 9.999999999999998224, 12.93301269999999192 ) ) ;
#6232=CARTESIAN_POINT ( 'NONE',  ( 69.25000000109245946, 7.933012699999995476, 14.99999999999999645 ) ) ;
#6244=CARTESIAN_POINT ( 'NONE',  ( -67.25000000109247367, 9.999999999999998224, 17.06698730000000097 ) ) ;
#6246=CARTESIAN_POINT ( 'NONE',  ( -66.65000000109247935, 9.999999999999998224, 17.06698730000000097 ) ) ;
#6248=ORIENTED_EDGE ( 'NONE', *, *, #7341, .F. ) ;
#6255=CARTESIAN_POINT ( 'NONE',  ( -69.10000000109248219, 7.933012699999995476, 14.14382582708705094 ) ) ;
#6257=CARTESIAN_POINT ( 'NONE',  ( 67.85000000109248219, 12.06698730000000097, 14.99999999999999645 ) ) ;
#6258=CARTESIAN_POINT ( 'NONE',  ( -68.15000000109246514, 11.46158073645647235, 16.46158073645647235 ) ) ;
#6266=EDGE_CURVE ( 'NONE', #1904, #13424, #15192, .T. ) ;
#6277=EDGE_CURVE ( 'NONE', #4086, #22517, #7407, .T. ) ;
#6285=CARTESIAN_POINT ( 'NONE',  ( -70.15000000218495302, 11.03553390593273598, 17.50000000000000355 ) ) ;
#6292=CARTESIAN_POINT ( 'NONE',  ( 68.55000000109247082, 11.46158073645647235, 13.53841926354352232 ) ) ;
#6294=DIRECTION ( 'NONE',  ( -1.000000000000000000, -0.000000000000000000, -0.000000000000000000 ) ) ;
#6300=CARTESIAN_POINT ( 'NONE',  ( -68.15000000109246514, 11.46158073645647235, 16.46158073645647235 ) ) ;
#6301=CARTESIAN_POINT ( 'NONE',  ( -70.00000000218494733, 12.50000000000000000, 14.99999999999999645 ) ) ;
#6316=CARTESIAN_POINT ( 'NONE',  ( 67.30000000109247082, 9.143825827087049163, 17.06698729999999742 ) ) ;
#6319=CARTESIAN_POINT ( 'NONE',  ( 69.30000000109247082, 7.933012699999995476, 14.14382582708705094 ) ) ;
#6333=CARTESIAN_POINT ( 'NONE',  ( -70.50000000000000000, 9.999999999999998224, 12.49999999999999289 ) ) ;
#6343=CARTESIAN_POINT ( 'NONE',  ( -68.60000000218495586, 9.999999999999998224, 17.49999999999999645 ) ) ;
#6344=ORIENTED_EDGE ( 'NONE', *, *, #21389, .F. ) ;
#6347=CARTESIAN_POINT ( 'NONE',  ( 70.10000000218494165, 11.76776695296636888, 16.76776695296636532 ) ) ;
#6350=CARTESIAN_POINT ( 'NONE',  ( 66.80000000109247082, 7.933012699999995476, 15.85617417291294196 ) ) ;
#6356=CARTESIAN_POINT ( 'NONE',  ( 69.35000000109246798, 8.538419263543524096, 13.53841926354352054 ) ) ;
#6360=ORIENTED_EDGE ( 'NONE', *, *, #19192, .T. ) ;
#6369=CARTESIAN_POINT ( 'NONE',  ( -68.25000000109245946, 9.999999999999998224, 17.06698730000000097 ) ) ;
#6372=DIRECTION ( 'NONE',  ( -1.000000000000000000, -0.000000000000000000, -0.000000000000000000 ) ) ;
#6377=CARTESIAN_POINT ( 'NONE',  ( -67.80000000109247082, 12.06698730000000275, 14.14382582708705094 ) ) ;
#6378=CARTESIAN_POINT ( 'NONE',  ( 66.75000000109247367, 8.538419263543524096, 13.53841926354352054 ) ) ;
#6379=CARTESIAN_POINT ( 'NONE',  ( -65.85000000109246798, 9.999999999999998224, 17.06698730000000097 ) ) ;
#6394=DIRECTION ( 'NONE',  ( -1.000000000000000000, -0.000000000000000000, -0.000000000000000000 ) ) ;
#6404=CARTESIAN_POINT ( 'NONE',  ( -70.60000000218494165, 9.999999999999998224, 12.49999999999999289 ) ) ;
#6413=CARTESIAN_POINT ( 'NONE',  ( 70.10000000109246798, 10.85617417291294551, 12.93301269999999370 ) ) ;
#6415=CARTESIAN_POINT ( 'NONE',  ( 72.50000000000000000, 9.999999999999998224, 14.99999999999999645 ) ) ;
#6419=CARTESIAN_POINT ( 'NONE',  ( -68.05000000109247082, 12.06698730000000097, 14.99999999999999645 ) ) ;
#6420=CARTESIAN_POINT ( 'NONE',  ( 72.50000000000000000, 9.999999999999998224, 17.49999999999999645 ) ) ;
#6434=EDGE_CURVE ( 'NONE', #3314, #683, #19114, .T. ) ;
#6435=CARTESIAN_POINT ( 'NONE',  ( 68.35000000109248219, 8.538419263543524096, 13.53841926354352054 ) ) ;
#6436=CARTESIAN_POINT ( 'NONE',  ( 69.40000000109246514, 9.143825827087050939, 12.93301269999999370 ) ) ;
#6448=ORIENTED_EDGE ( 'NONE', *, *, #2055, .F. ) ;
#6459=ORIENTED_EDGE ( 'NONE', *, *, #2192, .T. ) ;
#6463=CARTESIAN_POINT ( 'NONE',  ( 71.65000000109247935, 9.999999999999998224, 12.93301269999999192 ) ) ;
#6464=EDGE_CURVE ( 'NONE', #433, #3718, #8350, .T. ) ;
#6465=CARTESIAN_POINT ( 'NONE',  ( 71.10000000218494165, 8.232233047033627571, 16.76776695296636532 ) ) ;
#6469=CARTESIAN_POINT ( 'NONE',  ( 66.70000000109246230, 9.143825827087049163, 17.06698730000000097 ) ) ;
#6475=CARTESIAN_POINT ( 'NONE',  ( 68.95000000109247651, 11.46158073645647235, 16.46158073645647235 ) ) ;
#6477=CARTESIAN_POINT ( 'NONE',  ( 71.00000000218494733, 9.999999999999998224, 17.49999999999999645 ) ) ;
#6489=CARTESIAN_POINT ( 'NONE',  ( -67.40000000109247935, 10.85617417291294551, 17.06698729999999742 ) ) ;
#6497=DIRECTION ( 'NONE',  ( 1.000000000000000000, -0.000000000000000000, -0.000000000000000000 ) ) ;
#6499=CARTESIAN_POINT ( 'NONE',  ( -66.80000000218494449, 12.50000000000000000, 14.99999999999999645 ) ) ;
#6500=CARTESIAN_POINT ( 'NONE',  ( 66.00000000109247367, 9.143825827087052716, 12.93301269999999192 ) ) ;
#6503=CARTESIAN_POINT ( 'NONE',  ( -70.45000000000000284, 8.964466094067258695, 12.49999999999999289 ) ) ;
#6508=( BOUNDED_CURVE ( )  B_SPLINE_CURVE ( 2, ( #19962, #23689, #1395, #5242, #21874, #16278, #7179, #21757, #12346 ),
 .UNSPECIFIED., .F., .F. ) 
 B_SPLINE_CURVE_WITH_KNOTS ( ( 3, 2, 2, 2, 3 ),
 ( 0.5625000000000008882, 0.5781250000000007772, 0.5937500000000006661, 0.6093750000000006661, 0.6250000000000005551 ),
 .UNSPECIFIED. ) 
 CURVE ( )  GEOMETRIC_REPRESENTATION_ITEM ( )  RATIONAL_B_SPLINE_CURVE ( ( 0.9999999999999956701, 0.9238795325112910684, 1.000000000000000000, 0.9238795325112867385, 1.000000000000000000, 0.9238795325112867385, 1.000000000000000000, 0.9238795325112840739, 1.000000000000002665 ) ) 
 REPRESENTATION_ITEM ( '' )  );
#6523=VECTOR ( 'NONE', #19072, 1000.000000000000000 ) ;
#6528=CARTESIAN_POINT ( 'NONE',  ( -67.95000000218495018, 7.499999999999995559, 16.03553390593273420 ) ) ;
#6530=CARTESIAN_POINT ( 'NONE',  ( -72.00000000109245946, 12.06698730000000275, 14.14382582708705094 ) ) ;
#6535=CARTESIAN_POINT ( 'NONE',  ( 69.70000000109246230, 9.143825827087049163, 17.06698729999999742 ) ) ;
#6536=CARTESIAN_POINT ( 'NONE',  ( 71.00000000218494733, 9.999999999999998224, 17.49999999999999645 ) ) ;
#6543=CARTESIAN_POINT ( 'NONE',  ( -69.85000000109246798, 9.999999999999998224, 17.06698730000000097 ) ) ;
#6558=CARTESIAN_POINT ( 'NONE',  ( 68.00000000109247367, 10.85617417291294551, 17.06698729999999742 ) ) ;
#6559=CARTESIAN_POINT ( 'NONE',  ( 66.65000000109247935, 9.999999999999998224, 17.06698730000000097 ) ) ;
#6582=CARTESIAN_POINT ( 'NONE',  ( 71.80000000109247082, 12.06698729999999919, 14.14382582708705094 ) ) ;
#6583=CARTESIAN_POINT ( 'NONE',  ( 71.80000000218494449, 9.999999999999998224, 17.49999999999999645 ) ) ;
#6586=CARTESIAN_POINT ( 'NONE',  ( 68.20000000109246230, 10.85617417291294551, 17.06698730000000097 ) ) ;
#6591=CARTESIAN_POINT ( 'NONE',  ( 69.90000000109246514, 9.143825827087049163, 17.06698729999999742 ) ) ;
#6604=CARTESIAN_POINT ( 'NONE',  ( -66.15000000109247935, 8.538419263543524096, 13.53841926354352054 ) ) ;
#6608=CARTESIAN_POINT ( 'NONE',  ( -66.15000000218496723, 11.03553390593268624, 17.50000000000005329 ) ) ;
#6616=CARTESIAN_POINT ( 'NONE',  ( -69.64999999999999147, 8.964466094067258695, 12.49999999999999289 ) ) ;
#6629=CARTESIAN_POINT ( 'NONE',  ( -69.25000000109247367, 9.999999999999998224, 12.93301269999999192 ) ) ;
#6643=CARTESIAN_POINT ( 'NONE',  ( -66.45000000218495018, 7.499999999999995559, 13.96446609406725692 ) ) ;
#6645=CARTESIAN_POINT ( 'NONE',  ( -71.90000000109246514, 10.85617417291294551, 12.93301269999999370 ) ) ;
#6650=CARTESIAN_POINT ( 'NONE',  ( 68.35000000109248219, 8.538419263543524096, 13.53841926354352054 ) ) ;
#6656=CARTESIAN_POINT ( 'NONE',  ( 67.49999999999998579, 12.50000000000000000, 14.99999999999999645 ) ) ;
#6657=CARTESIAN_POINT ( 'NONE',  ( -69.20000000109246230, 7.933012699999995476, 15.85617417291294196 ) ) ;
#6672=CARTESIAN_POINT ( 'NONE',  ( 68.75000000109245946, 11.46158073645647235, 13.53841926354352232 ) ) ;
#6680=CARTESIAN_POINT ( 'NONE',  ( -66.60000000218495586, 9.999999999999998224, 12.49999999999999289 ) ) ;
#6685=CARTESIAN_POINT ( 'NONE',  ( -67.49999999999998579, 12.50000000000000000, 14.99999999999999645 ) ) ;
#6698=CARTESIAN_POINT ( 'NONE',  ( 66.65000000109247935, 9.999999999999998224, 17.06698730000000097 ) ) ;
#6700=CARTESIAN_POINT ( 'NONE',  ( -68.95000000218495018, 8.964466094067285340, 12.49999999999996980 ) ) ;
#6703=CARTESIAN_POINT ( 'NONE',  ( 67.65000000109247935, 7.933012699999995476, 14.99999999999999645 ) ) ;
#6705=DIRECTION ( 'NONE',  ( 0.000000000000000000, 0.000000000000000000, 1.000000000000000000 ) ) ;
#6716=ORIENTED_EDGE ( 'NONE', *, *, #11282, .F. ) ;
#6717=CARTESIAN_POINT ( 'NONE',  ( 72.50000000000000000, 9.999999999999998224, 17.49999999999999645 ) ) ;
#6727=CARTESIAN_POINT ( 'NONE',  ( -66.95000000218496439, 11.03553390593272887, 17.50000000000001066 ) ) ;
#6731=CARTESIAN_POINT ( 'NONE',  ( -68.95000000000000284, 11.03553390593273598, 12.49999999999999289 ) ) ;
#6738=CARTESIAN_POINT ( 'NONE',  ( -67.55000000218494449, 12.50000000000000000, 13.96446609406725692 ) ) ;
#6743=CARTESIAN_POINT ( 'NONE',  ( -72.05000000109247082, 9.999999999999998224, 17.06698730000000097 ) ) ;
#6744=ORIENTED_EDGE ( 'NONE', *, *, #20068, .F. ) ;
#6746=CARTESIAN_POINT ( 'NONE',  ( -69.10000000109248219, 7.933012699999995476, 14.14382582708705094 ) ) ;
#6748=DIRECTION ( 'NONE',  ( -1.000000000000000000, -0.000000000000000000, -0.000000000000000000 ) ) ;
#6752=CARTESIAN_POINT ( 'NONE',  ( 72.50000000000000000, 9.999999999999998224, 14.99999999999999645 ) ) ;
#6755=CARTESIAN_POINT ( 'NONE',  ( -67.70000000218493597, 11.76776695296636888, 16.76776695296636532 ) ) ;
#6783=CARTESIAN_POINT ( 'NONE',  ( 66.40000000109247935, 10.85617417291294551, 17.06698729999999742 ) ) ;
#6785=CARTESIAN_POINT ( 'NONE',  ( 71.84999999999999432, 7.499999999999995559, 16.03553390593273420 ) ) ;
#6787=CARTESIAN_POINT ( 'NONE',  ( -65.65000000218495302, 7.499999999999996447, 13.96446609406725514 ) ) ;
#6804=CARTESIAN_POINT ( 'NONE',  ( 72.05000000109247082, 9.999999999999998224, 17.06698730000000097 ) ) ;
#6807=CARTESIAN_POINT ( 'NONE',  ( -69.34999999999999432, 8.964466094067214286, 17.49999999999996092 ) ) ;
#6810=CARTESIAN_POINT ( 'NONE',  ( 68.20000000218495018, 9.999999999999998224, 12.49999999999999289 ) ) ;
#6814=CARTESIAN_POINT ( 'NONE',  ( 67.75000000109245946, 8.538419263543524096, 13.53841926354352054 ) ) ;
#6817=CARTESIAN_POINT ( 'NONE',  ( 72.50000000000000000, 9.999999999999998224, 17.49999999999999645 ) ) ;
#6839=ADVANCED_FACE ( 'NONE', ( #2677 ), #7968, .T. ) ;
#6840=CARTESIAN_POINT ( 'NONE',  ( -66.24999999999998579, 7.499999999999996447, 16.03553390593273775 ) ) ;
#6842=CARTESIAN_POINT ( 'NONE',  ( -67.70000000000000284, 9.999999999999998224, 17.49999999999999645 ) ) ;
#6845=CARTESIAN_POINT ( 'NONE',  ( -71.79999999999998295, 8.232233047033627571, 16.76776695296636532 ) ) ;
#6856=CARTESIAN_POINT ( 'NONE',  ( -71.60000000109246798, 9.143825827087052716, 12.93301269999999192 ) ) ;
#6859=CARTESIAN_POINT ( 'NONE',  ( -67.40000000109247935, 7.933012699999995476, 15.85617417291294196 ) ) ;
#6874=CARTESIAN_POINT ( 'NONE',  ( -67.60000000218495586, 12.50000000000000000, 14.99999999999999645 ) ) ;
#6902=CARTESIAN_POINT ( 'NONE',  ( -66.65000000000000568, 12.50000000000000000, 13.96446609406725692 ) ) ;
#6906=EDGE_CURVE ( 'NONE', #23355, #4600, #635, .T. ) ;
#6908=VERTEX_POINT ( 'NONE', #15287 ) ;
#6913=CARTESIAN_POINT ( 'NONE',  ( 65.95000000109246230, 8.538419263543522320, 16.46158073645647235 ) ) ;
#6938=ADVANCED_FACE ( 'NONE', ( #17535 ), #22787, .T. ) ;
#6940=CARTESIAN_POINT ( 'NONE',  ( 67.05000000218494449, 8.964466094067258695, 17.50000000000000355 ) ) ;
#6948=CARTESIAN_POINT ( 'NONE',  ( 67.95000000109247651, 11.46158073645647235, 13.53841926354352232 ) ) ;
#6960=EDGE_LOOP ( 'NONE', ( #2435, #16090, #11270, #13105, #17113, #10008, #17939, #2509, #23416, #18931, #11003, #8122, #14786, #21542, #9440, #21180, #467, #9827, #2600 ) ) ;
#6962=ORIENTED_EDGE ( 'NONE', *, *, #3510, .F. ) ;
#6970=CARTESIAN_POINT ( 'NONE',  ( -70.84999999999998010, 11.03553390593273598, 17.50000000000000355 ) ) ;
#6975=CARTESIAN_POINT ( 'NONE',  ( -65.80000000218494449, 9.999999999999998224, 12.49999999999999289 ) ) ;
#6979=CARTESIAN_POINT ( 'NONE',  ( -70.75000000109247367, 8.538419263543524096, 13.53841926354352054 ) ) ;
#6980=ORIENTED_EDGE ( 'NONE', *, *, #12634, .F. ) ;
#6982=CARTESIAN_POINT ( 'NONE',  ( -67.05000000109247082, 12.06698730000000097, 14.99999999999999645 ) ) ;
#6988=CARTESIAN_POINT ( 'NONE',  ( 71.24999999999998579, 8.964466094067205404, 12.50000000000004263 ) ) ;
#6991=CARTESIAN_POINT ( 'NONE',  ( -66.70000000218495018, 11.76776695296636888, 13.23223304703362579 ) ) ;
#6993=CARTESIAN_POINT ( 'NONE',  ( 72.50000000000000000, 9.999999999999998224, 17.49999999999999645 ) ) ;
#6998=CARTESIAN_POINT ( 'NONE',  ( -67.00000000218494733, 9.999999999999998224, 17.49999999999999645 ) ) ;
#7000=CARTESIAN_POINT ( 'NONE',  ( 67.29999999999999716, 9.999999999999998224, 12.49999999999999289 ) ) ;
#7006=CARTESIAN_POINT ( 'NONE',  ( 70.50000000218494733, 8.232233047033629347, 13.23223304703362402 ) ) ;
#7017=ORIENTED_EDGE ( 'NONE', *, *, #8863, .T. ) ;
#7025=CARTESIAN_POINT ( 'NONE',  ( 65.85000000109248219, 7.933012699999995476, 14.99999999999999645 ) ) ;
#7028=CARTESIAN_POINT ( 'NONE',  ( 70.74999999999998579, 12.50000000000000000, 16.03553390593273420 ) ) ;
#7031=CARTESIAN_POINT ( 'NONE',  ( -65.70000000218495018, 8.232233047033629347, 13.23223304703362402 ) ) ;
#7039=CARTESIAN_POINT ( 'NONE',  ( -70.50000000218494733, 8.232233047033629347, 13.23223304703362402 ) ) ;
#7049=CARTESIAN_POINT ( 'NONE',  ( 66.15000000218496723, 11.03553390593268624, 17.50000000000005329 ) ) ;
#7052=CARTESIAN_POINT ( 'NONE',  ( 68.05000000218494449, 7.499999999999995559, 13.96446609406725692 ) ) ;
#7063=CARTESIAN_POINT ( 'NONE',  ( 65.85000000109246798, 9.999999999999998224, 17.06698730000000097 ) ) ;
#7064=CARTESIAN_POINT ( 'NONE',  ( -69.25000000000000000, 11.03553390593269157, 17.50000000000004619 ) ) ;
#7090=CARTESIAN_POINT ( 'NONE',  ( -66.69999999999998863, 12.50000000000000000, 14.99999999999999645 ) ) ;
#7097=CARTESIAN_POINT ( 'NONE',  ( -66.35000000109246798, 11.46158073645647235, 13.53841926354352232 ) ) ;
#7102=CARTESIAN_POINT ( 'NONE',  ( -71.05000000109247082, 12.06698730000000097, 14.99999999999999645 ) ) ;
#7103=ORIENTED_EDGE ( 'NONE', *, *, #19938, .T. ) ;
#7105=CARTESIAN_POINT ( 'NONE',  ( -66.65000000109247935, 7.933012699999995476, 14.99999999999999645 ) ) ;
#7108=ORIENTED_EDGE ( 'NONE', *, *, #10504, .F. ) ;
#7116=CARTESIAN_POINT ( 'NONE',  ( -70.00000000109248788, 9.143825827087050939, 12.93301269999999370 ) ) ;
#7119=CARTESIAN_POINT ( 'NONE',  ( -70.90000000109245093, 7.933012699999995476, 14.14382582708705094 ) ) ;
#7121=DIRECTION ( 'NONE',  ( 0.000000000000000000, 0.000000000000000000, 1.000000000000000000 ) ) ;
#7148=CARTESIAN_POINT ( 'NONE',  ( 66.30000000109247082, 12.06698730000000275, 15.85617417291294196 ) ) ;
#7149=CARTESIAN_POINT ( 'NONE',  ( 70.84999999999998010, 11.03553390593273598, 17.50000000000000355 ) ) ;
#7151=CARTESIAN_POINT ( 'NONE',  ( 69.49999999999998579, 7.499999999999996447, 14.99999999999999645 ) ) ;
#7175=CARTESIAN_POINT ( 'NONE',  ( 69.10000000218495586, 11.76776695296636888, 13.23223304703362579 ) ) ;
#7178=FACE_OUTER_BOUND ( 'NONE', #4320, .T. ) ;
#7179=CARTESIAN_POINT ( 'NONE',  ( -68.59999999999999432, 8.232233047033627571, 16.76776695296636532 ) ) ;
#7187=CARTESIAN_POINT ( 'NONE',  ( 67.00000000109247367, 9.143825827087050939, 12.93301269999999370 ) ) ;
#7188=VECTOR ( 'NONE', #21975, 1000.000000000000000 ) ;
#7189=CARTESIAN_POINT ( 'NONE',  ( -67.95000000000001705, 7.499999999999996447, 13.96446609406725514 ) ) ;
#7217=CARTESIAN_POINT ( 'NONE',  ( -66.15000000000000568, 8.964466094067258695, 17.50000000000000355 ) ) ;
#7228=CARTESIAN_POINT ( 'NONE',  ( -70.20000000109246230, 12.06698729999999919, 14.14382582708705094 ) ) ;
#7231=CARTESIAN_POINT ( 'NONE',  ( -65.85000000109248219, 7.933012699999995476, 14.99999999999999645 ) ) ;
#7241=CARTESIAN_POINT ( 'NONE',  ( -71.90000000109247935, 12.06698730000000275, 15.85617417291294196 ) ) ;
#7242=CARTESIAN_POINT ( 'NONE',  ( -71.35000000109246798, 11.46158073645647235, 16.46158073645647235 ) ) ;
#7245=CARTESIAN_POINT ( 'NONE',  ( 72.50000000000000000, 9.999999999999998224, 12.49999999999999289 ) ) ;
#7274=CARTESIAN_POINT ( 'NONE',  ( 70.20000000000000284, 8.232233047033627571, 16.76776695296636532 ) ) ;
#7276=DIRECTION ( 'NONE',  ( -1.000000000000000000, -0.000000000000000000, -0.000000000000000000 ) ) ;
#7282=CYLINDRICAL_SURFACE ( 'NONE', #18714, 2.500000000000002220 ) ;
#7292=VERTEX_POINT ( 'NONE', #10608 ) ;
#7303=CARTESIAN_POINT ( 'NONE',  ( 69.30000000218494449, 11.76776695296636888, 16.76776695296636532 ) ) ;
#7305=DIRECTION ( 'NONE',  ( -1.000000000000000000, -0.000000000000000000, -0.000000000000000000 ) ) ;
#7316=CARTESIAN_POINT ( 'NONE',  ( -67.89999999999999147, 7.499999999999996447, 14.99999999999999645 ) ) ;
#7318=AXIS2_PLACEMENT_3D ( 'NONE', #3111, #10686, #17843 ) ;
#7340=CARTESIAN_POINT ( 'NONE',  ( -68.05000000000002558, 8.964466094067258695, 12.49999999999999289 ) ) ;
#7341=EDGE_CURVE ( 'NONE', #20172, #13175, #11425, .T. ) ;
#7346=CARTESIAN_POINT ( 'NONE',  ( 67.74999999999997158, 8.964466094067246260, 17.49999999999999289 ) ) ;
#7348=CYLINDRICAL_SURFACE ( 'NONE', #14949, 2.500000000000002220 ) ;
#7352=CARTESIAN_POINT ( 'NONE',  ( -68.70000000109247651, 12.06698729999999919, 15.85617417291294196 ) ) ;
#7355=CARTESIAN_POINT ( 'NONE',  ( -71.30000000109247082, 12.06698730000000275, 15.85617417291294196 ) ) ;
#7362=CARTESIAN_POINT ( 'NONE',  ( -70.15000000109247935, 11.46158073645647235, 13.53841926354352232 ) ) ;
#7363=CARTESIAN_POINT ( 'NONE',  ( -69.50000000109247367, 10.85617417291294551, 12.93301269999999370 ) ) ;
#7366=DIRECTION ( 'NONE',  ( 0.000000000000000000, 1.000000000000000000, -0.000000000000000000 ) ) ;
#7391=CARTESIAN_POINT ( 'NONE',  ( 68.25000000000000000, 12.50000000000000000, 13.96446609406725869 ) ) ;
#7404=CYLINDRICAL_SURFACE ( 'NONE', #9763, 2.500000000000002220 ) ;
#7407=LINE ( 'NONE', #11237, #7188 ) ;
#7415=CARTESIAN_POINT ( 'NONE',  ( 71.80000000109247082, 12.06698730000000275, 14.14382582708705094 ) ) ;
#7417=CARTESIAN_POINT ( 'NONE',  ( 71.25000000109247367, 12.06698730000000097, 14.99999999999999645 ) ) ;
#7422=( BOUNDED_SURFACE ( )  B_SPLINE_SURFACE ( 1, 2, ( 
 ( #5601, #5721, #11138, #12927, #20189, #15088, #9330, #4036, #5957, #14975, #3911, #4156, #16981, #16740, #320, #2355, #18412, #2234, #17094, #555, #7417, #2466, #22343, #4279, #11613, #3799, #13407, #20426, #444, #16622, #200, #7531, #14847, #22101, #13053, #11247, #18523, #2108, #9576, #11503, #9445, #5837, #11369, #7769, #18774, #9686, #7880, #15198, #18881, #9803, #22707, #18994, #10411, #10051, #21133, #668, #10287, #6436, #9927, #6319, #8004, #15441, #15789, #2823, #21247, #13875, #8243, #17339, #21018, #17226, #6672, #799, #13755, #1144, #6201, #23060, #907, #11845, #10170, #19123, #22596, #15562, #1025, #19347, #4865, #19470, #13634, #17462, #13985, #4633, #20785, #8130, #13519, #4747, #12200, #20895, #3068, #15327, #8486, #4391, #11730, #2583, #4510, #8359, #2710, #22822, #11968, #19233, #12080, #15676, #22952, #2937, #6559, #17576, #8710, #4992, #15898, #16014, #21370, #23176, #8591, #1616, #19582, #14344, #16248, #17918, #6913, #14463, #3539 ),
 ( #12559, #3646, #10874, #17691, #12791, #8958, #14590, #21849, #14107, #16364, #23420, #3425, #1253, #6785, #17801, #12320, #1372, #3179, #21486, #10525, #5099, #19820, #23539, #23304, #14230, #21607, #12433, #19697, #3300, #10644, #1501, #8843, #16138, #7149, #18148, #7028, #5215, #10765, #18041, #21728, #5341, #1732, #12684, #19937, #9072, #23659, #7274, #5454, #20043, #7744, #10983, #20520, #16711, #20159, #9304, #18262, #1964, #2330, #13137, #7852, #417, #18496, #20285, #7621, #3764, #16953, #11105, #289, #11469, #16481, #9663, #3886, #22070, #20400, #5687, #9196, #2079, #11346, #5929, #15177, #6049, #16595, #4007, #531, #14944, #7391, #18385, #59, #15059, #22435, #170, #13377, #20648, #18746, #1846, #14701, #21957, #5571, #18615, #12898, #7505, #14819, #13024, #22316, #11220, #2205, #13259, #9420, #22198, #5810, #9543, #16838, #4127, #7978, #2440, #18854, #11944, #6176, #881, #2797, #4478, #17194, #997, #13850, #13606, #20870, #22919, #15296, #22797 ) ),
 .UNSPECIFIED., .F., .F., .F. ) 
 B_SPLINE_SURFACE_WITH_KNOTS ( ( 2, 2 ),
 ( 3, 2, 2, 2, 2, 2, 2, 2, 2, 2, 2, 2, 2, 2, 2, 2, 2, 2, 2, 2, 2, 2, 2, 2, 2, 2, 2, 2, 2, 2, 2, 2, 2, 2, 2, 2, 2, 2, 2, 2, 2, 2, 2, 2, 2, 2, 2, 2, 2, 2, 2, 2, 2, 2, 2, 2, 2, 2, 2, 2, 2, 2, 2, 2, 3 ),
 ( 0.000000000000000000, 1.000000000000000000 ),
 ( 0.000000000000000000, 0.01562500000000000000, 0.03125000000000000000, 0.04687500000000000000, 0.06250000000000000000, 0.07812500000000000000, 0.09375000000000000000, 0.1093750000000000000, 0.1250000000000000000, 0.1406250000000000000, 0.1562500000000000000, 0.1718750000000000000, 0.1875000000000000000, 0.2031250000000000000, 0.2187500000000000000, 0.2343750000000000000, 0.2500000000000000000, 0.2656250000000000000, 0.2812500000000000000, 0.2968750000000000000, 0.3125000000000000000, 0.3281250000000000000, 0.3437500000000000000, 0.3593750000000000000, 0.3750000000000000000, 0.3906250000000000000, 0.4062500000000000000, 0.4218750000000000000, 0.4375000000000000000, 0.4531250000000000000, 0.4687500000000000000, 0.4843750000000000000, 0.5000000000000000000, 0.5156250000000000000, 0.5312500000000000000, 0.5468750000000000000, 0.5625000000000000000, 0.5781250000000000000, 0.5937500000000000000, 0.6093750000000000000, 0.6250000000000000000, 0.6406250000000000000, 0.6562500000000000000, 0.6718750000000000000, 0.6875000000000000000, 0.7031250000000000000, 0.7187500000000000000, 0.7343750000000000000, 0.7500000000000000000, 0.7656250000000000000, 0.7812500000000000000, 0.7968750000000000000, 0.8125000000000000000, 0.8281250000000000000, 0.8437500000000000000, 0.8593750000000000000, 0.8750000000000000000, 0.8906250000000000000, 0.9062500000000000000, 0.9218750000000000000, 0.9375000000000000000, 0.9531250000000000000, 0.9687500000000000000, 0.9843750000000000000, 1.000000000000000000 ),
 .UNSPECIFIED. ) 
 GEOMETRIC_REPRESENTATION_ITEM ( )  RATIONAL_B_SPLINE_SURFACE ( (
 ( 1.000000000000000000, 0.9238795325112867385, 1.000000000000000000, 0.9238795325112867385, 1.000000000000000000, 0.9238795325112867385, 1.000000000000000000, 0.9238795325112867385, 1.000000000000000000, 0.9238795325112867385, 1.000000000000000000, 0.9238795325112867385, 1.000000000000000000, 0.9238795325112867385, 1.000000000000000000, 0.9238795325112867385, 1.000000000000000000, 0.9238795325112867385, 1.000000000000000000, 0.9238795325112867385, 1.000000000000000000, 0.9238795325112867385, 1.000000000000000000, 0.9238795325112867385, 1.000000000000000000, 0.9238795325112867385, 1.000000000000000000, 0.9238795325112867385, 1.000000000000000000, 0.9238795325112867385, 1.000000000000000000, 0.9238795325112867385, 1.000000000000000000, 0.9238795325112867385, 1.000000000000000000, 0.9238795325112867385, 1.000000000000000000, 0.9238795325112867385, 1.000000000000000000, 0.9238795325112867385, 1.000000000000000000, 0.9238795325112867385, 1.000000000000000000, 0.9238795325112867385, 1.000000000000000000, 0.9238795325112867385, 1.000000000000000000, 0.9238795325112867385, 1.000000000000000000, 0.9238795325112867385, 1.000000000000000000, 0.9238795325112867385, 1.000000000000000000, 0.9238795325112867385, 1.000000000000000000, 0.9238795325112867385, 1.000000000000000000, 0.9238795325112867385, 1.000000000000000000, 0.9238795325112867385, 1.000000000000000000, 0.9238795325112867385, 1.000000000000000000, 0.9238795325112867385, 1.000000000000000000, 0.9238795325112867385, 1.000000000000000000, 0.9238795325112867385, 1.000000000000000000, 0.9238795325112867385, 1.000000000000000000, 0.9238795325112867385, 1.000000000000000000, 0.9238795325112867385, 1.000000000000000000, 0.9238795325112867385, 1.000000000000000000, 0.9238795325112867385, 1.000000000000000000, 0.9238795325112867385, 1.000000000000000000, 0.9238795325112867385, 1.000000000000000000, 0.9238795325112867385, 1.000000000000000000, 0.9238795325112867385, 1.000000000000000000, 0.9238795325112867385, 1.000000000000000000, 0.9238795325112867385, 1.000000000000000000, 0.9238795325112867385, 1.000000000000000000, 0.9238795325112867385, 1.000000000000000000, 0.9238795325112867385, 1.000000000000000000, 0.9238795325112867385, 1.000000000000000000, 0.9238795325112867385, 1.000000000000000000, 0.9238795325112867385, 1.000000000000000000, 0.9238795325112867385, 1.000000000000000000, 0.9238795325112867385, 1.000000000000000000, 0.9238795325112867385, 1.000000000000000000, 0.9238795325112867385, 1.000000000000000000, 0.9238795325112867385, 1.000000000000000000, 0.9238795325112867385, 1.000000000000000000, 0.9238795325112867385, 1.000000000000000000, 0.9238795325112867385, 1.000000000000000000, 0.9238795325112867385, 1.000000000000000000, 0.9238795325112867385, 1.000000000000000000, 0.9238795325112867385, 1.000000000000000000, 0.9238795325112867385, 1.000000000000000000, 0.9238795325112867385, 1.000000000000000000),
 ( 1.000000000000000000, 0.9238795325112867385, 1.000000000000000000, 0.9238795325112867385, 1.000000000000000000, 0.9238795325112867385, 1.000000000000000000, 0.9238795325112867385, 1.000000000000000000, 0.9238795325112867385, 1.000000000000000000, 0.9238795325112867385, 1.000000000000000000, 0.9238795325112867385, 1.000000000000000000, 0.9238795325112867385, 1.000000000000000000, 0.9238795325112867385, 1.000000000000000000, 0.9238795325112867385, 1.000000000000000000, 0.9238795325112867385, 1.000000000000000000, 0.9238795325112867385, 1.000000000000000000, 0.9238795325112867385, 1.000000000000000000, 0.9238795325112867385, 1.000000000000000000, 0.9238795325112867385, 1.000000000000000000, 0.9238795325112867385, 1.000000000000000000, 0.9238795325112867385, 1.000000000000000000, 0.9238795325112867385, 1.000000000000000000, 0.9238795325112867385, 1.000000000000000000, 0.9238795325112867385, 1.000000000000000000, 0.9238795325112867385, 1.000000000000000000, 0.9238795325112867385, 1.000000000000000000, 0.9238795325112867385, 1.000000000000000000, 0.9238795325112867385, 1.000000000000000000, 0.9238795325112867385, 1.000000000000000000, 0.9238795325112867385, 1.000000000000000000, 0.9238795325112867385, 1.000000000000000000, 0.9238795325112867385, 1.000000000000000000, 0.9238795325112867385, 1.000000000000000000, 0.9238795325112867385, 1.000000000000000000, 0.9238795325112867385, 1.000000000000000000, 0.9238795325112867385, 1.000000000000000000, 0.9238795325112867385, 1.000000000000000000, 0.9238795325112867385, 1.000000000000000000, 0.9238795325112867385, 1.000000000000000000, 0.9238795325112867385, 1.000000000000000000, 0.9238795325112867385, 1.000000000000000000, 0.9238795325112867385, 1.000000000000000000, 0.9238795325112867385, 1.000000000000000000, 0.9238795325112867385, 1.000000000000000000, 0.9238795325112867385, 1.000000000000000000, 0.9238795325112867385, 1.000000000000000000, 0.9238795325112867385, 1.000000000000000000, 0.9238795325112867385, 1.000000000000000000, 0.9238795325112867385, 1.000000000000000000, 0.9238795325112867385, 1.000000000000000000, 0.9238795325112867385, 1.000000000000000000, 0.9238795325112867385, 1.000000000000000000, 0.9238795325112867385, 1.000000000000000000, 0.9238795325112867385, 1.000000000000000000, 0.9238795325112867385, 1.000000000000000000, 0.9238795325112867385, 1.000000000000000000, 0.9238795325112867385, 1.000000000000000000, 0.9238795325112867385, 1.000000000000000000, 0.9238795325112867385, 1.000000000000000000, 0.9238795325112867385, 1.000000000000000000, 0.9238795325112867385, 1.000000000000000000, 0.9238795325112867385, 1.000000000000000000, 0.9238795325112867385, 1.000000000000000000, 0.9238795325112867385, 1.000000000000000000, 0.9238795325112867385, 1.000000000000000000, 0.9238795325112867385, 1.000000000000000000, 0.9238795325112867385, 1.000000000000000000, 0.9238795325112867385, 1.000000000000000000) ) ) 
 REPRESENTATION_ITEM ( '' )  SURFACE ( )  );
#7425=CARTESIAN_POINT ( 'NONE',  ( 66.95000000218496439, 11.03553390593272887, 17.50000000000001066 ) ) ;
#7426=CARTESIAN_POINT ( 'NONE',  ( -69.09999999999999432, 12.50000000000000000, 14.99999999999999645 ) ) ;
#7446=EDGE_CURVE ( 'NONE', #23552, #17274, #5726, .T. ) ;
#7448=CARTESIAN_POINT ( 'NONE',  ( -66.44999999999998863, 8.964466094067258695, 12.49999999999999289 ) ) ;
#7449=CARTESIAN_POINT ( 'NONE',  ( 66.35000000218495586, 7.499999999999996447, 16.03553390593273775 ) ) ;
#7450=CARTESIAN_POINT ( 'NONE',  ( 67.50000000109247367, 7.933012699999995476, 14.14382582708705094 ) ) ;
#7459=CARTESIAN_POINT ( 'NONE',  ( -67.60000000109248219, 9.143825827087052716, 12.93301269999999192 ) ) ;
#7462=CARTESIAN_POINT ( 'NONE',  ( -69.85000000109246798, 9.999999999999998224, 17.06698730000000097 ) ) ;
#7472=CARTESIAN_POINT ( 'NONE',  ( -65.70000000218495018, 8.232233047033629347, 13.23223304703362402 ) ) ;
#7476=CARTESIAN_POINT ( 'NONE',  ( -68.75000000109245946, 11.46158073645647235, 13.53841926354352232 ) ) ;
#7486=CARTESIAN_POINT ( 'NONE',  ( -71.75000000218496155, 11.03553390593273953, 17.50000000000000355 ) ) ;
#7505=CARTESIAN_POINT ( 'NONE',  ( 67.49999999999998579, 12.50000000000000000, 14.99999999999999645 ) ) ;
#7513=CARTESIAN_POINT ( 'NONE',  ( -71.85000000109246798, 9.999999999999998224, 12.93301269999999192 ) ) ;
#7519=VERTEX_POINT ( 'NONE', #5233 ) ;
#7528=CARTESIAN_POINT ( 'NONE',  ( 70.45000000109247651, 9.999999999999998224, 17.06698730000000097 ) ) ;
#7531=CARTESIAN_POINT ( 'NONE',  ( 70.70000000109247651, 9.143825827087049163, 17.06698729999999742 ) ) ;
#7550=CARTESIAN_POINT ( 'NONE',  ( 70.09999999999999432, 9.999999999999998224, 17.49999999999999645 ) ) ;
#7557=CARTESIAN_POINT ( 'NONE',  ( 65.85000000109246798, 9.999999999999998224, 17.06698730000000097 ) ) ;
#7560=CARTESIAN_POINT ( 'NONE',  ( 71.55000000109245661, 8.538419263543522320, 16.46158073645647235 ) ) ;
#7566=CARTESIAN_POINT ( 'NONE',  ( 72.10000000109246798, 12.06698730000000275, 15.85617417291294196 ) ) ;
#7572=CARTESIAN_POINT ( 'NONE',  ( -71.40000000218495302, 9.999999999999998224, 12.49999999999999289 ) ) ;
#7577=CARTESIAN_POINT ( 'NONE',  ( -70.25000000109247367, 12.06698730000000097, 14.99999999999999645 ) ) ;
#7580=CARTESIAN_POINT ( 'NONE',  ( -69.55000000109247082, 11.46158073645647235, 13.53841926354352232 ) ) ;
#7589=CARTESIAN_POINT ( 'NONE',  ( -69.90000000109247935, 7.933012699999995476, 14.14382582708705094 ) ) ;
#7590=CARTESIAN_POINT ( 'NONE',  ( -69.70000000109246230, 12.06698730000000275, 15.85617417291294196 ) ) ;
#7594=CARTESIAN_POINT ( 'NONE',  ( 72.09999999999999432, 9.999999999999998224, 12.49999999999999289 ) ) ;
#7603=CARTESIAN_POINT ( 'NONE',  ( -69.30000000218494449, 11.76776695296636888, 16.76776695296636532 ) ) ;
#7619=FACE_OUTER_BOUND ( 'NONE', #1340, .T. ) ;
#7621=CARTESIAN_POINT ( 'NONE',  ( 69.34999999999999432, 8.964466094067258695, 17.50000000000000355 ) ) ;
#7647=VERTEX_POINT ( 'NONE', #17090 ) ;
#7652=CARTESIAN_POINT ( 'NONE',  ( 70.20000000109246230, 12.06698730000000275, 14.14382582708705094 ) ) ;
#7670=( LENGTH_UNIT ( ) NAMED_UNIT ( * ) SI_UNIT ( .MILLI., .METRE. ) );
#7686=DIRECTION ( 'NONE',  ( 0.000000000000000000, 0.000000000000000000, 1.000000000000000000 ) ) ;
#7688=CARTESIAN_POINT ( 'NONE',  ( 69.70000000109247651, 12.06698729999999919, 15.85617417291294196 ) ) ;
#7694=CARTESIAN_POINT ( 'NONE',  ( 65.70000000109249072, 9.143825827087049163, 17.06698729999999742 ) ) ;
#7703=CARTESIAN_POINT ( 'NONE',  ( -67.75000000109247367, 11.46158073645647235, 13.53841926354352232 ) ) ;
#7706=CARTESIAN_POINT ( 'NONE',  ( -71.85000000109246798, 9.999999999999998224, 12.93301269999999192 ) ) ;
#7707=PRODUCT_CONTEXT ( 'NONE', #8871, 'mechanical' ) ;
#7716=CARTESIAN_POINT ( 'NONE',  ( -67.10000000109248219, 12.06698730000000275, 15.85617417291294196 ) ) ;
#7717=CARTESIAN_POINT ( 'NONE',  ( 68.70000000109247651, 12.06698729999999919, 15.85617417291294196 ) ) ;
#7719=CARTESIAN_POINT ( 'NONE',  ( -68.20000000109246230, 10.85617417291294551, 17.06698729999999742 ) ) ;
#7730=CARTESIAN_POINT ( 'NONE',  ( -70.34999999999999432, 7.499999999999996447, 13.96446609406725514 ) ) ;
#7741=CARTESIAN_POINT ( 'NONE',  ( -70.95000000218495018, 11.03553390593273598, 17.50000000000000355 ) ) ;
#7744=CARTESIAN_POINT ( 'NONE',  ( 70.05000000000002558, 11.03553390593273598, 17.50000000000000355 ) ) ;
#7752=DIRECTION ( 'NONE',  ( 0.000000000000000000, -1.000000000000000000, 0.000000000000000000 ) ) ;
#7754=FACE_OUTER_BOUND ( 'NONE', #14602, .T. ) ;
#7756=CARTESIAN_POINT ( 'NONE',  ( -70.80000000109248504, 9.143825827087050939, 12.93301269999999370 ) ) ;
#7757=VERTEX_POINT ( 'NONE', #16129 ) ;
#7767=CARTESIAN_POINT ( 'NONE',  ( 65.75000000218494733, 8.964466094067258695, 12.49999999999999289 ) ) ;
#7769=CARTESIAN_POINT ( 'NONE',  ( 70.10000000109245377, 7.933012699999995476, 14.14382582708705094 ) ) ;
#7774=CARTESIAN_POINT ( 'NONE',  ( -67.80000000218494449, 9.999999999999998224, 17.49999999999999645 ) ) ;
#7779=CARTESIAN_POINT ( 'NONE',  ( -67.25000000109245946, 12.06698730000000097, 14.99999999999999645 ) ) ;
#7781=ORIENTED_EDGE ( 'NONE', *, *, #906, .F. ) ;
#7786=CARTESIAN_POINT ( 'NONE',  ( 69.10000000218495586, 11.76776695296636888, 13.23223304703362579 ) ) ;
#7791=VERTEX_POINT ( 'NONE', #17796 ) ;
#7793=ORIENTED_EDGE ( 'NONE', *, *, #3510, .T. ) ;
#7799=CARTESIAN_POINT ( 'NONE',  ( 71.65000000109246514, 7.933012699999995476, 14.99999999999999645 ) ) ;
#7805=CARTESIAN_POINT ( 'NONE',  ( 66.35000000109248219, 11.46158073645647235, 16.46158073645647235 ) ) ;
#7812=CARTESIAN_POINT ( 'NONE',  ( 72.50000000000000000, 9.999999999999998224, 14.99999999999999645 ) ) ;
#7817=CARTESIAN_POINT ( 'NONE',  ( -72.10000000109246798, 12.06698730000000275, 15.85617417291294196 ) ) ;
#7825=CARTESIAN_POINT ( 'NONE',  ( -66.55000000109247082, 8.538419263543522320, 16.46158073645647235 ) ) ;
#7826=CARTESIAN_POINT ( 'NONE',  ( 70.00000000109247367, 9.143825827087052716, 12.93301269999999192 ) ) ;
#7828=CARTESIAN_POINT ( 'NONE',  ( -66.95000000109246230, 8.538419263543524096, 13.53841926354352054 ) ) ;
#7835=CARTESIAN_POINT ( 'NONE',  ( -69.10000000218495586, 11.76776695296636888, 13.23223304703362579 ) ) ;
#7838=ORIENTED_EDGE ( 'NONE', *, *, #17416, .F. ) ;
#7849=CARTESIAN_POINT ( 'NONE',  ( -69.15000000218495302, 12.50000000000000000, 13.96446609406725869 ) ) ;
#7852=CARTESIAN_POINT ( 'NONE',  ( 69.54999999999999716, 7.499999999999995559, 13.96446609406725692 ) ) ;
#7861=CARTESIAN_POINT ( 'NONE',  ( -71.80000000109245661, 9.143825827087052716, 12.93301269999999192 ) ) ;
#7862=EDGE_CURVE ( 'NONE', #3012, #6076, #21446, .T. ) ;
#7867=CARTESIAN_POINT ( 'NONE',  ( -70.65000000109247935, 7.933012699999995476, 14.99999999999999645 ) ) ;
#7868=ORIENTED_EDGE ( 'NONE', *, *, #8593, .T. ) ;
#7878=CARTESIAN_POINT ( 'NONE',  ( 69.95000000109247651, 8.538419263543524096, 13.53841926354352054 ) ) ;
#7879=CARTESIAN_POINT ( 'NONE',  ( 66.34999999999999432, 7.499999999999996447, 13.96446609406725514 ) ) ;
#7880=CARTESIAN_POINT ( 'NONE',  ( 69.95000000109247651, 8.538419263543522320, 16.46158073645647235 ) ) ;
#7890=CARTESIAN_POINT ( 'NONE',  ( -66.45000000109246230, 12.06698730000000097, 14.99999999999999645 ) ) ;
#7892=CARTESIAN_POINT ( 'NONE',  ( 72.50000000000000000, 9.999999999999998224, 14.99999999999999645 ) ) ;
#7901=ADVANCED_FACE ( 'NONE', ( #8585 ), #14223, .T. ) ;
#7907=( BOUNDED_CURVE ( )  B_SPLINE_CURVE ( 2, ( #9002, #14511, #21775, #16296, #3468, #5385, #12724, #1188, #15829 ),
 .UNSPECIFIED., .F., .F. ) 
 B_SPLINE_CURVE_WITH_KNOTS ( ( 3, 2, 2, 2, 3 ),
 ( 0.000000000000000000, 0.01562499999999990459, 0.03124999999999980918, 0.04687499999999971551, 0.06249999999999961836 ),
 .UNSPECIFIED. ) 
 CURVE ( )  GEOMETRIC_REPRESENTATION_ITEM ( )  RATIONAL_B_SPLINE_CURVE ( ( 1.000000000000000000, 0.9238795325112867385, 1.000000000000000000, 0.9238795325112867385, 1.000000000000000000, 0.9238795325112867385, 1.000000000000000000, 0.9238795325112886259, 0.9999999999999981126 ) ) 
 REPRESENTATION_ITEM ( '' )  );
#7912=FILL_AREA_STYLE_COLOUR ( '', #9473 ) ;
#7913=CARTESIAN_POINT ( 'NONE',  ( 70.90000000109246514, 7.933012699999995476, 14.14382582708705094 ) ) ;
#7918=CARTESIAN_POINT ( 'NONE',  ( 69.40000000109246514, 9.143825827087050939, 12.93301269999999370 ) ) ;
#7932=CARTESIAN_POINT ( 'NONE',  ( -67.55000000109247082, 8.538419263543522320, 16.46158073645647235 ) ) ;
#7933=SHAPE_DEFINITION_REPRESENTATION ( #22708, #9307 ) ;
#7935=VERTEX_POINT ( 'NONE', #14454 ) ;
#7942=AXIS2_PLACEMENT_3D ( 'NONE', #10042, #4265, #22693 ) ;
#7944=CARTESIAN_POINT ( 'NONE',  ( -66.50000000109247367, 9.143825827087049163, 17.06698729999999742 ) ) ;
#7945=CARTESIAN_POINT ( 'NONE',  ( 69.25000000109247367, 9.999999999999998224, 12.93301269999999192 ) ) ;
#7946=( BOUNDED_CURVE ( )  B_SPLINE_CURVE ( 2, ( #12033, #4698, #22896, #2774, #19070, #13940, #2660, #13702, #17293 ),
 .UNSPECIFIED., .F., .F. ) 
 B_SPLINE_CURVE_WITH_KNOTS ( ( 3, 2, 2, 2, 3 ),
 ( 0.1249999999999992367, 0.1406249999999996947, 0.1562500000000001388, 0.1718750000000005829, 0.1875000000000010270 ),
 .UNSPECIFIED. ) 
 CURVE ( )  GEOMETRIC_REPRESENTATION_ITEM ( )  RATIONAL_B_SPLINE_CURVE ( ( 1.000000000000003775, 0.9238795325112830747, 1.000000000000000000, 0.9238795325112867385, 1.000000000000000000, 0.9238795325112867385, 1.000000000000000000, 0.9238795325112817425, 1.000000000000005107 ) ) 
 REPRESENTATION_ITEM ( '' )  );
#7947=CARTESIAN_POINT ( 'NONE',  ( -72.00000000000000000, 8.232233047033629347, 13.23223304703362402 ) ) ;
#7963=EDGE_CURVE ( 'NONE', #5505, #11622, #4042, .T. ) ;
#7968=CYLINDRICAL_SURFACE ( 'NONE', #4898, 2.500000000000002220 ) ;
#7973=CARTESIAN_POINT ( 'NONE',  ( -70.85000000218494165, 12.50000000000000000, 16.03553390593273420 ) ) ;
#7974=LINE ( 'NONE', #19207, #3328 ) ;
#7978=CARTESIAN_POINT ( 'NONE',  ( 66.84999999999999432, 11.03553390593273598, 17.50000000000000355 ) ) ;
#7980=CARTESIAN_POINT ( 'NONE',  ( 70.20000000109246230, 12.06698730000000275, 14.14382582708705094 ) ) ;
#7986=CARTESIAN_POINT ( 'NONE',  ( -71.55000000109245661, 8.538419263543522320, 16.46158073645647235 ) ) ;
#7992=CARTESIAN_POINT ( 'NONE',  ( -71.00000000109247367, 12.06698730000000275, 14.14382582708705094 ) ) ;
#8001=CARTESIAN_POINT ( 'NONE',  ( 68.55000000109247082, 11.46158073645647235, 13.53841926354352232 ) ) ;
#8004=CARTESIAN_POINT ( 'NONE',  ( 69.25000000109245946, 7.933012699999995476, 14.99999999999999645 ) ) ;
#8021=ORIENTED_EDGE ( 'NONE', *, *, #13604, .T. ) ;
#8025=CARTESIAN_POINT ( 'NONE',  ( -70.95000000218495018, 11.03553390593269867, 17.50000000000003908 ) ) ;
#8040=CARTESIAN_POINT ( 'NONE',  ( 71.75000000109247367, 8.538419263543524096, 13.53841926354352054 ) ) ;
#8047=CARTESIAN_POINT ( 'NONE',  ( 70.45000000109247651, 12.06698730000000097, 14.99999999999999645 ) ) ;
#8058=CARTESIAN_POINT ( 'NONE',  ( -67.40000000109247935, 7.933012699999995476, 15.85617417291294196 ) ) ;
#8061=CARTESIAN_POINT ( 'NONE',  ( -67.45000000109246230, 9.999999999999998224, 17.06698730000000097 ) ) ;
#8062=( BOUNDED_CURVE ( )  B_SPLINE_CURVE ( 2, ( #3626, #14323, #8818, #3282, #21582, #23639, #19920, #19800, #18240 ),
 .UNSPECIFIED., .F., .F. ) 
 B_SPLINE_CURVE_WITH_KNOTS ( ( 3, 2, 2, 2, 3 ),
 ( 0.6250000000000005551, 0.6406250000000004441, 0.6562500000000003331, 0.6718750000000002220, 0.6875000000000001110 ),
 .UNSPECIFIED. ) 
 CURVE ( )  GEOMETRIC_REPRESENTATION_ITEM ( )  RATIONAL_B_SPLINE_CURVE ( ( 0.9999999999999973355, 0.9238795325112894030, 1.000000000000000000, 0.9238795325112867385, 1.000000000000000000, 0.9238795325112867385, 1.000000000000000000, 0.9238795325112861834, 1.000000000000000444 ) ) 
 REPRESENTATION_ITEM ( '' )  );
#8067=EDGE_CURVE ( 'NONE', #23046, #3718, #14479, .T. ) ;
#8068=ORIENTED_EDGE ( 'NONE', *, *, #445, .F. ) ;
#8071=VECTOR ( 'NONE', #9813, 1000.000000000000000 ) ;
#8073=CARTESIAN_POINT ( 'NONE',  ( -67.65000000109247935, 9.999999999999998224, 12.93301269999999192 ) ) ;
#8076=CARTESIAN_POINT ( 'NONE',  ( 69.90000000109247935, 7.933012699999995476, 14.14382582708705094 ) ) ;
#8077=CARTESIAN_POINT ( 'NONE',  ( -66.60000000109246798, 10.85617417291294551, 17.06698729999999742 ) ) ;
#8084=DIRECTION ( 'NONE',  ( -1.000000000000000000, -0.000000000000000000, -0.000000000000000000 ) ) ;
#8099=( BOUNDED_SURFACE ( )  B_SPLINE_SURFACE ( 1, 2, ( 
 ( #6804, #21262, #14124, #21388, #4762, #21506, #5009, #8501, #21148, #15805, #19362, #1160, #5116, #10308, #12338, #3316, #13498, #1000, #18972, #15768, #22572, #19096, #11821, #15532, #20873, #9776, #882, #2688, #2443, #4366, #17434, #12056, #646, #775, #4612, #17197, #4481, #7980, #13729, #6413, #15652, #10029, #8333, #22679, #8108, #17316, #21108, #6535, #20992, #8217, #15418, #17073, #15299, #13853, #22800, #11947, #19212, #2800, #13963, #9903, #22923, #10143, #2554, #4723, #19322, #2911, #17552, #6178, #10259, #20759, #6292, #1117, #8462, #23039, #6650, #11703, #21222, #4837, #18857, #13609, #14886, #3840, #11408, #12968, #11049, #20346, #5762, #22019, #20230, #11537, #16544, #7450, #16658, #20588, #2390, #18807, #18335, #13320, #3953, #11287, #9367, #15121, #233, #14765, #2274, #18562, #14649, #3708, #18447, #9480, #13201, #2145, #1917, #20105, #7805, #5514, #16779, #22383, #5993, #9614, #4195, #9722, #17017, #13090, #22143, #120, #360, #7694, #15010 ),
 ( #11175, #9258, #593, #7566, #18685, #21906, #12848, #22265, #5635, #5877, #16904, #2027, #20467, #4073, #481, #4430, #22629, #8162, #13670, #17135, #11999, #11765, #20933, #8397, #13445, #22986, #17261, #19034, #17371, #2623, #4777, #711, #829, #8278, #19156, #10083, #8047, #13907, #18916, #939, #15593, #20707, #6115, #4665, #12114, #15362, #2972, #6591, #15714, #10324, #15473, #4549, #21165, #1059, #19265, #19376, #17614, #7918, #6356, #22743, #6232, #11885, #2743, #22861, #9967, #22505, #6475, #2505, #13553, #9839, #15238, #13796, #2853, #4312, #11650, #21053, #20820, #10203, #17491, #4901, #16286, #3334, #3102, #21405, #15929, #1402, #6948, #10444, #5250, #5023, #14263, #1652, #6703, #23579, #10560, #12353, #10678, #19615, #21767, #17724, #17835, #1533, #12471, #17953, #1287, #7187, #12237, #8875, #16169, #14017, #23092, #21644, #5376, #8625, #19969, #14502, #8996, #3571, #8744, #12597, #3213, #23455, #8517, #12717, #10907, #14140, #23205, #5134, #7063 ) ),
 .UNSPECIFIED., .F., .F., .F. ) 
 B_SPLINE_SURFACE_WITH_KNOTS ( ( 2, 2 ),
 ( 3, 2, 2, 2, 2, 2, 2, 2, 2, 2, 2, 2, 2, 2, 2, 2, 2, 2, 2, 2, 2, 2, 2, 2, 2, 2, 2, 2, 2, 2, 2, 2, 2, 2, 2, 2, 2, 2, 2, 2, 2, 2, 2, 2, 2, 2, 2, 2, 2, 2, 2, 2, 2, 2, 2, 2, 2, 2, 2, 2, 2, 2, 2, 2, 3 ),
 ( 0.000000000000000000, 1.000000000000000000 ),
 ( 0.000000000000000000, 0.01562500000000000000, 0.03125000000000000000, 0.04687500000000000000, 0.06250000000000000000, 0.07812500000000000000, 0.09375000000000000000, 0.1093750000000000000, 0.1250000000000000000, 0.1406250000000000000, 0.1562500000000000000, 0.1718750000000000000, 0.1875000000000000000, 0.2031250000000000000, 0.2187500000000000000, 0.2343750000000000000, 0.2500000000000000000, 0.2656250000000000000, 0.2812500000000000000, 0.2968750000000000000, 0.3125000000000000000, 0.3281250000000000000, 0.3437500000000000000, 0.3593750000000000000, 0.3750000000000000000, 0.3906250000000000000, 0.4062500000000000000, 0.4218750000000000000, 0.4375000000000000000, 0.4531250000000000000, 0.4687500000000000000, 0.4843750000000000000, 0.5000000000000000000, 0.5156250000000000000, 0.5312500000000000000, 0.5468750000000000000, 0.5625000000000000000, 0.5781250000000000000, 0.5937500000000000000, 0.6093750000000000000, 0.6250000000000000000, 0.6406250000000000000, 0.6562500000000000000, 0.6718750000000000000, 0.6875000000000000000, 0.7031250000000000000, 0.7187500000000000000, 0.7343750000000000000, 0.7500000000000000000, 0.7656250000000000000, 0.7812500000000000000, 0.7968750000000000000, 0.8125000000000000000, 0.8281250000000000000, 0.8437500000000000000, 0.8593750000000000000, 0.8750000000000000000, 0.8906250000000000000, 0.9062500000000000000, 0.9218750000000000000, 0.9375000000000000000, 0.9531250000000000000, 0.9687500000000000000, 0.9843750000000000000, 1.000000000000000000 ),
 .UNSPECIFIED. ) 
 GEOMETRIC_REPRESENTATION_ITEM ( )  RATIONAL_B_SPLINE_SURFACE ( (
 ( 1.000000000000000000, 0.9238795325112867385, 1.000000000000000000, 0.9238795325112867385, 1.000000000000000000, 0.9238795325112867385, 1.000000000000000000, 0.9238795325112867385, 1.000000000000000000, 0.9238795325112867385, 1.000000000000000000, 0.9238795325112867385, 1.000000000000000000, 0.9238795325112867385, 1.000000000000000000, 0.9238795325112867385, 1.000000000000000000, 0.9238795325112867385, 1.000000000000000000, 0.9238795325112867385, 1.000000000000000000, 0.9238795325112867385, 1.000000000000000000, 0.9238795325112867385, 1.000000000000000000, 0.9238795325112867385, 1.000000000000000000, 0.9238795325112867385, 1.000000000000000000, 0.9238795325112867385, 1.000000000000000000, 0.9238795325112867385, 1.000000000000000000, 0.9238795325112867385, 1.000000000000000000, 0.9238795325112867385, 1.000000000000000000, 0.9238795325112867385, 1.000000000000000000, 0.9238795325112867385, 1.000000000000000000, 0.9238795325112867385, 1.000000000000000000, 0.9238795325112867385, 1.000000000000000000, 0.9238795325112867385, 1.000000000000000000, 0.9238795325112867385, 1.000000000000000000, 0.9238795325112867385, 1.000000000000000000, 0.9238795325112867385, 1.000000000000000000, 0.9238795325112867385, 1.000000000000000000, 0.9238795325112867385, 1.000000000000000000, 0.9238795325112867385, 1.000000000000000000, 0.9238795325112867385, 1.000000000000000000, 0.9238795325112867385, 1.000000000000000000, 0.9238795325112867385, 1.000000000000000000, 0.9238795325112867385, 1.000000000000000000, 0.9238795325112867385, 1.000000000000000000, 0.9238795325112867385, 1.000000000000000000, 0.9238795325112867385, 1.000000000000000000, 0.9238795325112867385, 1.000000000000000000, 0.9238795325112867385, 1.000000000000000000, 0.9238795325112867385, 1.000000000000000000, 0.9238795325112867385, 1.000000000000000000, 0.9238795325112867385, 1.000000000000000000, 0.9238795325112867385, 1.000000000000000000, 0.9238795325112867385, 1.000000000000000000, 0.9238795325112867385, 1.000000000000000000, 0.9238795325112867385, 1.000000000000000000, 0.9238795325112867385, 1.000000000000000000, 0.9238795325112867385, 1.000000000000000000, 0.9238795325112867385, 1.000000000000000000, 0.9238795325112867385, 1.000000000000000000, 0.9238795325112867385, 1.000000000000000000, 0.9238795325112867385, 1.000000000000000000, 0.9238795325112867385, 1.000000000000000000, 0.9238795325112867385, 1.000000000000000000, 0.9238795325112867385, 1.000000000000000000, 0.9238795325112867385, 1.000000000000000000, 0.9238795325112867385, 1.000000000000000000, 0.9238795325112867385, 1.000000000000000000, 0.9238795325112867385, 1.000000000000000000, 0.9238795325112867385, 1.000000000000000000, 0.9238795325112867385, 1.000000000000000000, 0.9238795325112867385, 1.000000000000000000, 0.9238795325112867385, 1.000000000000000000, 0.9238795325112867385, 1.000000000000000000, 0.9238795325112867385, 1.000000000000000000),
 ( 1.000000000000000000, 0.9238795325112867385, 1.000000000000000000, 0.9238795325112867385, 1.000000000000000000, 0.9238795325112867385, 1.000000000000000000, 0.9238795325112867385, 1.000000000000000000, 0.9238795325112867385, 1.000000000000000000, 0.9238795325112867385, 1.000000000000000000, 0.9238795325112867385, 1.000000000000000000, 0.9238795325112867385, 1.000000000000000000, 0.9238795325112867385, 1.000000000000000000, 0.9238795325112867385, 1.000000000000000000, 0.9238795325112867385, 1.000000000000000000, 0.9238795325112867385, 1.000000000000000000, 0.9238795325112867385, 1.000000000000000000, 0.9238795325112867385, 1.000000000000000000, 0.9238795325112867385, 1.000000000000000000, 0.9238795325112867385, 1.000000000000000000, 0.9238795325112867385, 1.000000000000000000, 0.9238795325112867385, 1.000000000000000000, 0.9238795325112867385, 1.000000000000000000, 0.9238795325112867385, 1.000000000000000000, 0.9238795325112867385, 1.000000000000000000, 0.9238795325112867385, 1.000000000000000000, 0.9238795325112867385, 1.000000000000000000, 0.9238795325112867385, 1.000000000000000000, 0.9238795325112867385, 1.000000000000000000, 0.9238795325112867385, 1.000000000000000000, 0.9238795325112867385, 1.000000000000000000, 0.9238795325112867385, 1.000000000000000000, 0.9238795325112867385, 1.000000000000000000, 0.9238795325112867385, 1.000000000000000000, 0.9238795325112867385, 1.000000000000000000, 0.9238795325112867385, 1.000000000000000000, 0.9238795325112867385, 1.000000000000000000, 0.9238795325112867385, 1.000000000000000000, 0.9238795325112867385, 1.000000000000000000, 0.9238795325112867385, 1.000000000000000000, 0.9238795325112867385, 1.000000000000000000, 0.9238795325112867385, 1.000000000000000000, 0.9238795325112867385, 1.000000000000000000, 0.9238795325112867385, 1.000000000000000000, 0.9238795325112867385, 1.000000000000000000, 0.9238795325112867385, 1.000000000000000000, 0.9238795325112867385, 1.000000000000000000, 0.9238795325112867385, 1.000000000000000000, 0.9238795325112867385, 1.000000000000000000, 0.9238795325112867385, 1.000000000000000000, 0.9238795325112867385, 1.000000000000000000, 0.9238795325112867385, 1.000000000000000000, 0.9238795325112867385, 1.000000000000000000, 0.9238795325112867385, 1.000000000000000000, 0.9238795325112867385, 1.000000000000000000, 0.9238795325112867385, 1.000000000000000000, 0.9238795325112867385, 1.000000000000000000, 0.9238795325112867385, 1.000000000000000000, 0.9238795325112867385, 1.000000000000000000, 0.9238795325112867385, 1.000000000000000000, 0.9238795325112867385, 1.000000000000000000, 0.9238795325112867385, 1.000000000000000000, 0.9238795325112867385, 1.000000000000000000, 0.9238795325112867385, 1.000000000000000000, 0.9238795325112867385, 1.000000000000000000, 0.9238795325112867385, 1.000000000000000000, 0.9238795325112867385, 1.000000000000000000, 0.9238795325112867385, 1.000000000000000000) ) ) 
 REPRESENTATION_ITEM ( '' )  SURFACE ( )  );
#8100=CARTESIAN_POINT ( 'NONE',  ( -69.10000000218495586, 11.76776695296636888, 13.23223304703362579 ) ) ;
#8108=CARTESIAN_POINT ( 'NONE',  ( 69.85000000109248219, 7.933012699999995476, 14.99999999999999645 ) ) ;
#8115=CARTESIAN_POINT ( 'NONE',  ( -68.80000000109247082, 12.06698729999999919, 14.14382582708705094 ) ) ;
#8121=CARTESIAN_POINT ( 'NONE',  ( -69.80000000109247082, 7.933012699999995476, 15.85617417291294196 ) ) ;
#8122=ORIENTED_EDGE ( 'NONE', *, *, #5286, .T. ) ;
#8124=DIRECTION ( 'NONE',  ( -1.000000000000000000, -0.000000000000000000, -0.000000000000000000 ) ) ;
#8129=CARTESIAN_POINT ( 'NONE',  ( 68.40000000109249356, 9.143825827087050939, 12.93301269999999370 ) ) ;
#8130=CARTESIAN_POINT ( 'NONE',  ( 67.70000000109246230, 7.933012699999995476, 14.14382582708705094 ) ) ;
#8135=CARTESIAN_POINT ( 'NONE',  ( 71.50000000218496155, 11.76776695296636888, 13.23223304703362579 ) ) ;
#8151=ORIENTED_EDGE ( 'NONE', *, *, #16575, .F. ) ;
#8154=CARTESIAN_POINT ( 'NONE',  ( 71.55000000218494449, 12.50000000000000000, 13.96446609406725869 ) ) ;
#8158=CARTESIAN_POINT ( 'NONE',  ( 66.95000000109246230, 8.538419263543524096, 13.53841926354352054 ) ) ;
#8162=CARTESIAN_POINT ( 'NONE',  ( 71.40000000109246514, 10.85617417291294551, 17.06698729999999742 ) ) ;
#8172=CARTESIAN_POINT ( 'NONE',  ( -67.30000000109247082, 9.143825827087049163, 17.06698730000000097 ) ) ;
#8174=CARTESIAN_POINT ( 'NONE',  ( -67.20000000109247651, 12.06698730000000275, 14.14382582708705094 ) ) ;
#8180=EDGE_CURVE ( 'NONE', #5464, #14452, #11461, .T. ) ;
#8183=CARTESIAN_POINT ( 'NONE',  ( -67.85000000109248219, 12.06698730000000097, 14.99999999999999645 ) ) ;
#8185=CARTESIAN_POINT ( 'NONE',  ( 70.30000000109247082, 12.06698729999999919, 15.85617417291294196 ) ) ;
#8186=CARTESIAN_POINT ( 'NONE',  ( -66.05000000109247082, 7.933012699999995476, 14.99999999999999645 ) ) ;
#8204=DIRECTION ( 'NONE',  ( 0.000000000000000000, 0.000000000000000000, 1.000000000000000000 ) ) ;
#8212=CARTESIAN_POINT ( 'NONE',  ( -70.50000000218494733, 8.232233047033629347, 13.23223304703362402 ) ) ;
#8213=DIRECTION ( 'NONE',  ( -1.000000000000000000, 0.000000000000000000, 0.000000000000000000 ) ) ;
#8217=CARTESIAN_POINT ( 'NONE',  ( 69.60000000109249640, 10.85617417291294551, 17.06698729999999742 ) ) ;
#8224=CARTESIAN_POINT ( 'NONE',  ( -69.05000000109247082, 9.999999999999998224, 17.06698730000000097 ) ) ;
#8241=CARTESIAN_POINT ( 'NONE',  ( 69.70000000109246230, 9.143825827087049163, 17.06698729999999742 ) ) ;
#8242=VECTOR ( 'NONE', #5389, 1000.000000000000000 ) ;
#8243=CARTESIAN_POINT ( 'NONE',  ( 68.95000000109247651, 11.46158073645647235, 16.46158073645647235 ) ) ;
#8256=VERTEX_POINT ( 'NONE', #8675 ) ;
#8264=CARTESIAN_POINT ( 'NONE',  ( 72.50000000000000000, 9.999999999999998224, 17.49999999999999645 ) ) ;
#8267=CARTESIAN_POINT ( 'NONE',  ( 71.75000000109248788, 11.46158073645647235, 13.53841926354352232 ) ) ;
#8268=CARTESIAN_POINT ( 'NONE',  ( 70.45000000218493597, 7.499999999999995559, 13.96446609406725692 ) ) ;
#8273=CARTESIAN_POINT ( 'NONE',  ( 66.60000000109246798, 10.85617417291294551, 17.06698730000000097 ) ) ;
#8278=CARTESIAN_POINT ( 'NONE',  ( 70.60000000109246798, 10.85617417291294551, 17.06698729999999742 ) ) ;
#8281=DIRECTION ( 'NONE',  ( -1.000000000000000000, -0.000000000000000000, -0.000000000000000000 ) ) ;
#8289=CARTESIAN_POINT ( 'NONE',  ( -67.65000000109247935, 7.933012699999995476, 14.99999999999999645 ) ) ;
#8298=EDGE_CURVE ( 'NONE', #23552, #18582, #10130, .T. ) ;
#8299=CARTESIAN_POINT ( 'NONE',  ( -71.45000000000000284, 12.50000000000000000, 13.96446609406725869 ) ) ;
#8316=CARTESIAN_POINT ( 'NONE',  ( 72.50000000000000000, 9.999999999999998224, 14.99999999999999645 ) ) ;
#8321=CARTESIAN_POINT ( 'NONE',  ( -67.30000000218494449, 8.232233047033629347, 13.23223304703362402 ) ) ;
#8324=ADVANCED_FACE ( 'NONE', ( #15759 ), #14193, .T. ) ;
#8333=CARTESIAN_POINT ( 'NONE',  ( 69.95000000109247651, 8.538419263543524096, 13.53841926354352054 ) ) ;
#8340=CARTESIAN_POINT ( 'NONE',  ( -70.15000000109246514, 8.538419263543524096, 13.53841926354352054 ) ) ;
#8342=CARTESIAN_POINT ( 'NONE',  ( 65.80000000218494449, 9.999999999999998224, 12.49999999999999289 ) ) ;
#8344=CARTESIAN_POINT ( 'NONE',  ( 72.50000000000000000, 9.999999999999998224, 12.49999999999999289 ) ) ;
#8347=ORIENTED_EDGE ( 'NONE', *, *, #18759, .T. ) ;
#8350=LINE ( 'NONE', #793, #3724 ) ;
#8352=ORIENTED_EDGE ( 'NONE', *, *, #17460, .F. ) ;
#8358=CARTESIAN_POINT ( 'NONE',  ( 69.80000000109247082, 7.933012699999995476, 15.85617417291294196 ) ) ;
#8359=CARTESIAN_POINT ( 'NONE',  ( 67.10000000109246798, 10.85617417291294551, 12.93301269999999370 ) ) ;
#8360=ADVANCED_FACE ( 'NONE', ( #19662 ), #17882, .T. ) ;
#8361=ORIENTED_EDGE ( 'NONE', *, *, #985, .F. ) ;
#8367=CARTESIAN_POINT ( 'NONE',  ( 66.65000000218496723, 11.03553390593276973, 12.50000000000002665 ) ) ;
#8368=DIRECTION ( 'NONE',  ( 0.000000000000000000, 0.000000000000000000, 1.000000000000000000 ) ) ;
#8377=ORIENTED_EDGE ( 'NONE', *, *, #5733, .F. ) ;
#8385=CARTESIAN_POINT ( 'NONE',  ( 71.95000000109247651, 11.46158073645647235, 16.46158073645647235 ) ) ;
#8390=CARTESIAN_POINT ( 'NONE',  ( 68.15000000109246514, 11.46158073645647235, 16.46158073645647235 ) ) ;
#8392=CARTESIAN_POINT ( 'NONE',  ( 72.50000000000000000, 9.999999999999998224, 17.49999999999999645 ) ) ;
#8397=CARTESIAN_POINT ( 'NONE',  ( 71.10000000109246798, 10.85617417291294551, 12.93301269999999370 ) ) ;
#8399=CARTESIAN_POINT ( 'NONE',  ( 72.50000000000000000, 9.999999999999998224, 14.99999999999999645 ) ) ;
#8407=CARTESIAN_POINT ( 'NONE',  ( 65.75000000109245946, 9.999999999999998224, 17.49999999999999645 ) ) ;
#8414=EDGE_LOOP ( 'NONE', ( #21266, #6448, #19522, #8753 ) ) ;
#8415=CARTESIAN_POINT ( 'NONE',  ( -66.70000000109246230, 9.143825827087049163, 17.06698729999999742 ) ) ;
#8426=CARTESIAN_POINT ( 'NONE',  ( 66.25000000109247367, 12.06698730000000097, 14.99999999999999645 ) ) ;
#8427=CARTESIAN_POINT ( 'NONE',  ( -69.84999999999999432, 12.50000000000000000, 13.96446609406725869 ) ) ;
#8429=EDGE_CURVE ( 'NONE', #13424, #17245, #16101, .T. ) ;
#8434=CARTESIAN_POINT ( 'NONE',  ( -67.45000000218493597, 11.03553390593273420, 12.49999999999998934 ) ) ;
#8441=CARTESIAN_POINT ( 'NONE',  ( -70.90000000109247935, 10.85617417291294551, 12.93301269999999192 ) ) ;
#8452=DIRECTION ( 'NONE',  ( 0.000000000000000000, 0.000000000000000000, 1.000000000000000000 ) ) ;
#8455=CARTESIAN_POINT ( 'NONE',  ( -67.90000000218495302, 8.232233047033627571, 16.76776695296636532 ) ) ;
#8462=CARTESIAN_POINT ( 'NONE',  ( 68.45000000109247651, 9.999999999999998224, 12.93301269999999192 ) ) ;
#8463=CARTESIAN_POINT ( 'NONE',  ( 70.60000000218494165, 9.999999999999998224, 12.49999999999999289 ) ) ;
#8469=CARTESIAN_POINT ( 'NONE',  ( -68.90000000109246514, 12.06698729999999919, 15.85617417291294196 ) ) ;
#8478=EDGE_CURVE ( 'NONE', #18582, #7791, #16442, .T. ) ;
#8485=CARTESIAN_POINT ( 'NONE',  ( 69.50000000109248788, 12.06698730000000275, 15.85617417291294196 ) ) ;
#8486=CARTESIAN_POINT ( 'NONE',  ( 67.35000000109246798, 11.46158073645647235, 16.46158073645647235 ) ) ;
#8495=CYLINDRICAL_SURFACE ( 'NONE', #7, 2.500000000000002220 ) ;
#8501=CARTESIAN_POINT ( 'NONE',  ( 71.70000000109247651, 10.85617417291294551, 12.93301269999999370 ) ) ;
#8509=CARTESIAN_POINT ( 'NONE',  ( 70.75000000218496155, 12.50000000000000000, 13.96446609406725869 ) ) ;
#8513=CARTESIAN_POINT ( 'NONE',  ( 68.75000000109245946, 11.46158073645647235, 13.53841926354352232 ) ) ;
#8517=CARTESIAN_POINT ( 'NONE',  ( 66.15000000109247935, 8.538419263543524096, 13.53841926354352054 ) ) ;
#8534=ORIENTED_EDGE ( 'NONE', *, *, #22795, .T. ) ;
#8539=CARTESIAN_POINT ( 'NONE',  ( 67.05000000109247082, 12.06698730000000097, 14.99999999999999645 ) ) ;
#8540=CARTESIAN_POINT ( 'NONE',  ( -71.09999999999999432, 7.499999999999996447, 14.99999999999999645 ) ) ;
#8544=CARTESIAN_POINT ( 'NONE',  ( 67.10000000218495586, 8.232233047033627571, 16.76776695296636532 ) ) ;
#8545=DIRECTION ( 'NONE',  ( -1.000000000000000000, -0.000000000000000000, -0.000000000000000000 ) ) ;
#8562=CARTESIAN_POINT ( 'NONE',  ( -66.65000000218493881, 11.03553390593273598, 12.49999999999999289 ) ) ;
#8573=CARTESIAN_POINT ( 'NONE',  ( 67.70000000000000284, 9.999999999999998224, 17.49999999999999645 ) ) ;
#8574=CARTESIAN_POINT ( 'NONE',  ( -68.55000000109247082, 8.538419263543524096, 13.53841926354352054 ) ) ;
#8585=FACE_OUTER_BOUND ( 'NONE', #15166, .T. ) ;
#8589=CARTESIAN_POINT ( 'NONE',  ( -69.45000000218495018, 8.964466094067256918, 17.49999999999999289 ) ) ;
#8591=CARTESIAN_POINT ( 'NONE',  ( 66.25000000109245946, 9.999999999999998224, 12.93301269999999192 ) ) ;
#8593=EDGE_CURVE ( 'NONE', #14452, #4468, #8706, .T. ) ;
#8608=FACE_OUTER_BOUND ( 'NONE', #2543, .T. ) ;
#8611=CARTESIAN_POINT ( 'NONE',  ( -69.59999999999999432, 8.232233047033629347, 13.23223304703362402 ) ) ;
#8616=AXIS2_PLACEMENT_3D ( 'NONE', #5609, #18419, #1998 ) ;
#8617=CARTESIAN_POINT ( 'NONE',  ( 68.75000000218496155, 7.499999999999995559, 16.03553390593273420 ) ) ;
#8619=CARTESIAN_POINT ( 'NONE',  ( 67.85000000109246798, 9.999999999999998224, 12.93301269999999192 ) ) ;
#8622=CARTESIAN_POINT ( 'NONE',  ( -68.85000000218495586, 7.499999999999996447, 13.96446609406725514 ) ) ;
#8625=CARTESIAN_POINT ( 'NONE',  ( 66.60000000109246798, 10.85617417291294551, 17.06698729999999742 ) ) ;
#8635=EDGE_CURVE ( 'NONE', #21124, #5860, #191, .T. ) ;
#8649=CARTESIAN_POINT ( 'NONE',  ( -66.90000000218495302, 11.76776695296636888, 16.76776695296636532 ) ) ;
#8650=ADVANCED_FACE ( 'NONE', ( #21365 ), #4987, .T. ) ;
#8652=CARTESIAN_POINT ( 'NONE',  ( 66.35000000109248219, 11.46158073645647235, 16.46158073645647235 ) ) ;
#8654=CARTESIAN_POINT ( 'NONE',  ( -71.54999999999999716, 12.50000000000000000, 16.03553390593273420 ) ) ;
#8655=ADVANCED_FACE ( 'NONE', ( #7619 ), #22194, .T. ) ;
#8662=CARTESIAN_POINT ( 'NONE',  ( -66.55000000218494449, 8.964466094067294222, 12.49999999999996092 ) ) ;
#8669=CARTESIAN_POINT ( 'NONE',  ( -68.30000000109247082, 7.933012699999995476, 14.14382582708705094 ) ) ;
#8672=ORIENTED_EDGE ( 'NONE', *, *, #21355, .T. ) ;
#8675=CARTESIAN_POINT ( 'NONE',  ( -65.85000000109246798, 9.999999999999998224, 17.06698730000000097 ) ) ;
#8678=CARTESIAN_POINT ( 'NONE',  ( -68.25000000218494733, 11.03553390593273598, 12.49999999999999289 ) ) ;
#8679=( BOUNDED_CURVE ( )  B_SPLINE_CURVE ( 2, ( #1443, #8662, #19769, #23611, #10714, #3494, #17991, #3601, #23487 ),
 .UNSPECIFIED., .F., .F. ) 
 B_SPLINE_CURVE_WITH_KNOTS ( ( 3, 2, 2, 2, 3 ),
 ( 0.8124999999999993339, 0.8281249999999992228, 0.8437499999999991118, 0.8593749999999991118, 0.8749999999999990008 ),
 .UNSPECIFIED. ) 
 CURVE ( )  GEOMETRIC_REPRESENTATION_ITEM ( )  RATIONAL_B_SPLINE_CURVE ( ( 1.000000000000003331, 0.9238795325112835188, 1.000000000000000000, 0.9238795325112867385, 1.000000000000000000, 0.9238795325112867385, 1.000000000000000000, 0.9238795325112916235, 0.9999999999999951150 ) ) 
 REPRESENTATION_ITEM ( '' )  );
#8695=ORIENTED_EDGE ( 'NONE', *, *, #13673, .F. ) ;
#8706=LINE ( 'NONE', #15464, #13693 ) ;
#8710=CARTESIAN_POINT ( 'NONE',  ( 66.55000000109247082, 11.46158073645647235, 16.46158073645647235 ) ) ;
#8712=CARTESIAN_POINT ( 'NONE',  ( 69.75000000218496155, 8.964466094067244484, 12.50000000000000711 ) ) ;
#8716=CARTESIAN_POINT ( 'NONE',  ( 67.90000000218495302, 8.232233047033627571, 16.76776695296636532 ) ) ;
#8726=CARTESIAN_POINT ( 'NONE',  ( -67.39999999999999147, 11.76776695296636888, 13.23223304703362579 ) ) ;
#8730=ORIENTED_EDGE ( 'NONE', *, *, #11102, .F. ) ;
#8733=CARTESIAN_POINT ( 'NONE',  ( 68.35000000218495586, 12.50000000000000000, 13.96446609406725869 ) ) ;
#8735=DIRECTION ( 'NONE',  ( 0.000000000000000000, 0.000000000000000000, 1.000000000000000000 ) ) ;
#8741=CARTESIAN_POINT ( 'NONE',  ( -69.00000000218494733, 9.999999999999998224, 12.49999999999999289 ) ) ;
#8744=CARTESIAN_POINT ( 'NONE',  ( 66.35000000109246798, 11.46158073645647235, 13.53841926354352232 ) ) ;
#8753=ORIENTED_EDGE ( 'NONE', *, *, #1468, .F. ) ;
#8767=CARTESIAN_POINT ( 'NONE',  ( -66.49999999999998579, 9.999999999999998224, 12.49999999999999289 ) ) ;
#8768=CARTESIAN_POINT ( 'NONE',  ( -65.65000000109247935, 9.999999999999998224, 17.06698730000000097 ) ) ;
#8774=CARTESIAN_POINT ( 'NONE',  ( -70.70000000000000284, 12.50000000000000000, 14.99999999999999645 ) ) ;
#8783=ORIENTED_EDGE ( 'NONE', *, *, #7862, .T. ) ;
#8784=CARTESIAN_POINT ( 'NONE',  ( -71.15000000109247935, 11.46158073645647235, 16.46158073645647235 ) ) ;
#8787=CARTESIAN_POINT ( 'NONE',  ( -67.00000000109247367, 12.06698730000000275, 14.14382582708705094 ) ) ;
#8804=CARTESIAN_POINT ( 'NONE',  ( -68.10000000218495586, 8.232233047033629347, 13.23223304703362402 ) ) ;
#8818=CARTESIAN_POINT ( 'NONE',  ( -68.39999999999999147, 11.76776695296636888, 16.76776695296636532 ) ) ;
#8823=EDGE_LOOP ( 'NONE', ( #18823, #17003, #10751, #6744, #21091 ) ) ;
#8834=CARTESIAN_POINT ( 'NONE',  ( -66.74999999999998579, 12.50000000000000000, 16.03553390593273775 ) ) ;
#8835=ORIENTED_EDGE ( 'NONE', *, *, #1266, .F. ) ;
#8841=ADVANCED_FACE ( 'NONE', ( #17309 ), #15689, .F. ) ;
#8843=CARTESIAN_POINT ( 'NONE',  ( 70.95000000000000284, 8.964466094067258695, 17.50000000000000355 ) ) ;
#8860=CARTESIAN_POINT ( 'NONE',  ( 65.95000000218495018, 12.50000000000000000, 13.96446609406725692 ) ) ;
#8863=EDGE_CURVE ( 'NONE', #9892, #18376, #10026, .T. ) ;
#8864=CARTESIAN_POINT ( 'NONE',  ( 69.05000000218494449, 11.03553390593273598, 12.49999999999999289 ) ) ;
#8865=( BOUNDED_CURVE ( )  B_SPLINE_CURVE ( 2, ( #7572, #22149, #366, #15016, #9619, #5882, #20472, #4078, #16910 ),
 .UNSPECIFIED., .F., .F. ) 
 B_SPLINE_CURVE_WITH_KNOTS ( ( 3, 2, 2, 2, 3 ),
 ( 0.06249999999999961836, 0.07812499999999952816, 0.09374999999999943101, 0.1093749999999993339, 0.1249999999999992367 ),
 .UNSPECIFIED. ) 
 CURVE ( )  GEOMETRIC_REPRESENTATION_ITEM ( )  RATIONAL_B_SPLINE_CURVE ( ( 1.000000000000001776, 0.9238795325112848511, 1.000000000000000000, 0.9238795325112867385, 1.000000000000000000, 0.9238795325112867385, 1.000000000000000000, 0.9238795325112904022, 0.9999999999999963363 ) ) 
 REPRESENTATION_ITEM ( '' )  );
#8871=APPLICATION_CONTEXT ( 'automotive_design' ) ;
#8875=CARTESIAN_POINT ( 'NONE',  ( 66.90000000109246514, 7.933012699999995476, 14.14382582708705094 ) ) ;
#8877=CARTESIAN_POINT ( 'NONE',  ( -69.14999999999999147, 12.50000000000000000, 16.03553390593273775 ) ) ;
#8884=CARTESIAN_POINT ( 'NONE',  ( 68.09999999999999432, 9.999999999999998224, 12.49999999999999289 ) ) ;
#8887=ORIENTED_EDGE ( 'NONE', *, *, #19191, .F. ) ;
#8896=CARTESIAN_POINT ( 'NONE',  ( -67.95000000000000284, 7.499999999999995559, 13.96446609406725692 ) ) ;
#8897=CARTESIAN_POINT ( 'NONE',  ( 66.50000000218494733, 8.232233047033629347, 13.23223304703362402 ) ) ;
#8902=CARTESIAN_POINT ( 'NONE',  ( -67.70000000218493597, 11.76776695296636888, 16.76776695296636532 ) ) ;
#8911=CARTESIAN_POINT ( 'NONE',  ( -66.75000000109247367, 8.538419263543524096, 13.53841926354352054 ) ) ;
#8923=CARTESIAN_POINT ( 'NONE',  ( -70.05000000109247082, 9.999999999999998224, 12.93301269999999192 ) ) ;
#8947=ORIENTED_EDGE ( 'NONE', *, *, #1468, .T. ) ;
#8952=DIRECTION ( 'NONE',  ( -1.000000000000000000, -0.000000000000000000, -0.000000000000000000 ) ) ;
#8958=CARTESIAN_POINT ( 'NONE',  ( 72.25000000000000000, 12.50000000000000000, 13.96446609406725869 ) ) ;
#8970=CARTESIAN_POINT ( 'NONE',  ( -70.30000000218494449, 8.232233047033627571, 16.76776695296636532 ) ) ;
#8973=( BOUNDED_SURFACE ( )  B_SPLINE_SURFACE ( 1, 2, ( 
 ( #6583, #9831, #19368, #22850, #2612, #8154, #17124, #822, #1169, #11989, #21268, #22977, #17364, #2733, #6465, #9956, #15812, #15465, #13787, #10315, #15353, #8509, #932, #20922, #19258, #4540, #22620, #8268, #10193, #4771, #21155, #22736, #12226, #23084, #6347, #4656, #13897, #2962, #17484, #17604, #13660, #1050, #4891, #19495, #11877, #9096, #10897, #23447, #23568, #21635, #7303, #12344, #16276, #1758, #7175, #8864, #16389, #1392, #16041, #8987, #18177, #8617, #19725, #17716, #3451, #23686, #12813, #21398, #10552, #8733, #14610, #21872, #6810, #3322, #10667, #7052, #5124, #1278, #16160, #1525, #5478, #14373, #3092, #5239, #17826, #15919, #23197, #12461, #5015, #10435, #17943, #14132, #12583, #14490, #19606, #6940, #23331, #19843, #5365, #21753, #10788, #18063, #14255, #21513, #12708, #1643, #19960, #3204, #3562, #552, #16619, #2230, #22340, #81, #3909, #4152, #11245, #5835, #13161, #20072, #14724, #7767, #22459, #11367, #3672, #20423, #15196, #4033, #14973 ),
 ( #18644, #11008, #2353, #9442, #11135, #7415, #18291, #18410, #21985, #1874, #9222, #9573, #5599, #16737, #16867, #20308, #9327, #442, #5955, #5717, #13051, #15086, #12925, #22224, #13279, #16504, #9684, #318, #1988, #20186, #3795, #198, #7528, #14844, #22098, #20548, #18519, #7652, #11499, #2106, #18772, #16978, #7878, #6071, #22706, #8358, #17093, #8241, #23058, #22950, #13404, #8485, #4632, #10286, #17574, #9802, #12078, #19120, #22820, #20671, #18880, #13518, #4276, #20784, #15325, #17222, #2463, #798, #15561, #11966, #8001, #11610, #17338, #8129, #6435, #1023, #19345, #15674, #667, #2581, #19232, #6558, #11843, #13633, #22595, #10050, #905, #2822, #13874, #6199, #10166, #4388, #11729, #18993, #9925, #6316, #17461, #15439, #21131, #2708, #20894, #4508, #13753, #21015, #4746, #2935, #1141, #15788, #14229, #16013, #3299, #15896, #12681, #6783, #12432, #7148, #12198, #21727, #23301, #17800, #16137, #1371, #4861, #21484, #7025, #1615, #10873, #1729, #4989 ) ),
 .UNSPECIFIED., .F., .F., .F. ) 
 B_SPLINE_SURFACE_WITH_KNOTS ( ( 2, 2 ),
 ( 3, 2, 2, 2, 2, 2, 2, 2, 2, 2, 2, 2, 2, 2, 2, 2, 2, 2, 2, 2, 2, 2, 2, 2, 2, 2, 2, 2, 2, 2, 2, 2, 2, 2, 2, 2, 2, 2, 2, 2, 2, 2, 2, 2, 2, 2, 2, 2, 2, 2, 2, 2, 2, 2, 2, 2, 2, 2, 2, 2, 2, 2, 2, 2, 3 ),
 ( 0.000000000000000000, 1.000000000000000000 ),
 ( 0.000000000000000000, 0.01562500000000000000, 0.03125000000000000000, 0.04687500000000000000, 0.06250000000000000000, 0.07812500000000000000, 0.09375000000000000000, 0.1093750000000000000, 0.1250000000000000000, 0.1406250000000000000, 0.1562500000000000000, 0.1718750000000000000, 0.1875000000000000000, 0.2031250000000000000, 0.2187500000000000000, 0.2343750000000000000, 0.2500000000000000000, 0.2656250000000000000, 0.2812500000000000000, 0.2968750000000000000, 0.3125000000000000000, 0.3281250000000000000, 0.3437500000000000000, 0.3593750000000000000, 0.3750000000000000000, 0.3906250000000000000, 0.4062500000000000000, 0.4218750000000000000, 0.4375000000000000000, 0.4531250000000000000, 0.4687500000000000000, 0.4843750000000000000, 0.5000000000000000000, 0.5156250000000000000, 0.5312500000000000000, 0.5468750000000000000, 0.5625000000000000000, 0.5781250000000000000, 0.5937500000000000000, 0.6093750000000000000, 0.6250000000000000000, 0.6406250000000000000, 0.6562500000000000000, 0.6718750000000000000, 0.6875000000000000000, 0.7031250000000000000, 0.7187500000000000000, 0.7343750000000000000, 0.7500000000000000000, 0.7656250000000000000, 0.7812500000000000000, 0.7968750000000000000, 0.8125000000000000000, 0.8281250000000000000, 0.8437500000000000000, 0.8593750000000000000, 0.8750000000000000000, 0.8906250000000000000, 0.9062500000000000000, 0.9218750000000000000, 0.9375000000000000000, 0.9531250000000000000, 0.9687500000000000000, 0.9843750000000000000, 1.000000000000000000 ),
 .UNSPECIFIED. ) 
 GEOMETRIC_REPRESENTATION_ITEM ( )  RATIONAL_B_SPLINE_SURFACE ( (
 ( 1.000000000000000000, 0.9238795325112867385, 1.000000000000000000, 0.9238795325112867385, 1.000000000000000000, 0.9238795325112867385, 1.000000000000000000, 0.9238795325112867385, 1.000000000000000000, 0.9238795325112867385, 1.000000000000000000, 0.9238795325112867385, 1.000000000000000000, 0.9238795325112867385, 1.000000000000000000, 0.9238795325112867385, 1.000000000000000000, 0.9238795325112867385, 1.000000000000000000, 0.9238795325112867385, 1.000000000000000000, 0.9238795325112867385, 1.000000000000000000, 0.9238795325112867385, 1.000000000000000000, 0.9238795325112867385, 1.000000000000000000, 0.9238795325112867385, 1.000000000000000000, 0.9238795325112867385, 1.000000000000000000, 0.9238795325112867385, 1.000000000000000000, 0.9238795325112867385, 1.000000000000000000, 0.9238795325112867385, 1.000000000000000000, 0.9238795325112867385, 1.000000000000000000, 0.9238795325112867385, 1.000000000000000000, 0.9238795325112867385, 1.000000000000000000, 0.9238795325112867385, 1.000000000000000000, 0.9238795325112867385, 1.000000000000000000, 0.9238795325112867385, 1.000000000000000000, 0.9238795325112867385, 1.000000000000000000, 0.9238795325112867385, 1.000000000000000000, 0.9238795325112867385, 1.000000000000000000, 0.9238795325112867385, 1.000000000000000000, 0.9238795325112867385, 1.000000000000000000, 0.9238795325112867385, 1.000000000000000000, 0.9238795325112867385, 1.000000000000000000, 0.9238795325112867385, 1.000000000000000000, 0.9238795325112867385, 1.000000000000000000, 0.9238795325112867385, 1.000000000000000000, 0.9238795325112867385, 1.000000000000000000, 0.9238795325112867385, 1.000000000000000000, 0.9238795325112867385, 1.000000000000000000, 0.9238795325112867385, 1.000000000000000000, 0.9238795325112867385, 1.000000000000000000, 0.9238795325112867385, 1.000000000000000000, 0.9238795325112867385, 1.000000000000000000, 0.9238795325112867385, 1.000000000000000000, 0.9238795325112867385, 1.000000000000000000, 0.9238795325112867385, 1.000000000000000000, 0.9238795325112867385, 1.000000000000000000, 0.9238795325112867385, 1.000000000000000000, 0.9238795325112867385, 1.000000000000000000, 0.9238795325112867385, 1.000000000000000000, 0.9238795325112867385, 1.000000000000000000, 0.9238795325112867385, 1.000000000000000000, 0.9238795325112867385, 1.000000000000000000, 0.9238795325112867385, 1.000000000000000000, 0.9238795325112867385, 1.000000000000000000, 0.9238795325112867385, 1.000000000000000000, 0.9238795325112867385, 1.000000000000000000, 0.9238795325112867385, 1.000000000000000000, 0.9238795325112867385, 1.000000000000000000, 0.9238795325112867385, 1.000000000000000000, 0.9238795325112867385, 1.000000000000000000, 0.9238795325112867385, 1.000000000000000000, 0.9238795325112867385, 1.000000000000000000, 0.9238795325112867385, 1.000000000000000000, 0.9238795325112867385, 1.000000000000000000, 0.9238795325112867385, 1.000000000000000000),
 ( 1.000000000000000000, 0.9238795325112867385, 1.000000000000000000, 0.9238795325112867385, 1.000000000000000000, 0.9238795325112867385, 1.000000000000000000, 0.9238795325112867385, 1.000000000000000000, 0.9238795325112867385, 1.000000000000000000, 0.9238795325112867385, 1.000000000000000000, 0.9238795325112867385, 1.000000000000000000, 0.9238795325112867385, 1.000000000000000000, 0.9238795325112867385, 1.000000000000000000, 0.9238795325112867385, 1.000000000000000000, 0.9238795325112867385, 1.000000000000000000, 0.9238795325112867385, 1.000000000000000000, 0.9238795325112867385, 1.000000000000000000, 0.9238795325112867385, 1.000000000000000000, 0.9238795325112867385, 1.000000000000000000, 0.9238795325112867385, 1.000000000000000000, 0.9238795325112867385, 1.000000000000000000, 0.9238795325112867385, 1.000000000000000000, 0.9238795325112867385, 1.000000000000000000, 0.9238795325112867385, 1.000000000000000000, 0.9238795325112867385, 1.000000000000000000, 0.9238795325112867385, 1.000000000000000000, 0.9238795325112867385, 1.000000000000000000, 0.9238795325112867385, 1.000000000000000000, 0.9238795325112867385, 1.000000000000000000, 0.9238795325112867385, 1.000000000000000000, 0.9238795325112867385, 1.000000000000000000, 0.9238795325112867385, 1.000000000000000000, 0.9238795325112867385, 1.000000000000000000, 0.9238795325112867385, 1.000000000000000000, 0.9238795325112867385, 1.000000000000000000, 0.9238795325112867385, 1.000000000000000000, 0.9238795325112867385, 1.000000000000000000, 0.9238795325112867385, 1.000000000000000000, 0.9238795325112867385, 1.000000000000000000, 0.9238795325112867385, 1.000000000000000000, 0.9238795325112867385, 1.000000000000000000, 0.9238795325112867385, 1.000000000000000000, 0.9238795325112867385, 1.000000000000000000, 0.9238795325112867385, 1.000000000000000000, 0.9238795325112867385, 1.000000000000000000, 0.9238795325112867385, 1.000000000000000000, 0.9238795325112867385, 1.000000000000000000, 0.9238795325112867385, 1.000000000000000000, 0.9238795325112867385, 1.000000000000000000, 0.9238795325112867385, 1.000000000000000000, 0.9238795325112867385, 1.000000000000000000, 0.9238795325112867385, 1.000000000000000000, 0.9238795325112867385, 1.000000000000000000, 0.9238795325112867385, 1.000000000000000000, 0.9238795325112867385, 1.000000000000000000, 0.9238795325112867385, 1.000000000000000000, 0.9238795325112867385, 1.000000000000000000, 0.9238795325112867385, 1.000000000000000000, 0.9238795325112867385, 1.000000000000000000, 0.9238795325112867385, 1.000000000000000000, 0.9238795325112867385, 1.000000000000000000, 0.9238795325112867385, 1.000000000000000000, 0.9238795325112867385, 1.000000000000000000, 0.9238795325112867385, 1.000000000000000000, 0.9238795325112867385, 1.000000000000000000, 0.9238795325112867385, 1.000000000000000000, 0.9238795325112867385, 1.000000000000000000, 0.9238795325112867385, 1.000000000000000000) ) ) 
 REPRESENTATION_ITEM ( '' )  SURFACE ( )  );
#8978=EDGE_CURVE ( 'NONE', #4760, #16067, #9253, .T. ) ;
#8979=ORIENTED_EDGE ( 'NONE', *, *, #8635, .F. ) ;
#8987=CARTESIAN_POINT ( 'NONE',  ( 68.85000000218495586, 7.499999999999995559, 13.96446609406725692 ) ) ;
#8996=CARTESIAN_POINT ( 'NONE',  ( 66.45000000109246230, 12.06698730000000097, 14.99999999999999645 ) ) ;
#9002=CARTESIAN_POINT ( 'NONE',  ( -72.50000000000000000, 9.999999999999998224, 17.49999999999999645 ) ) ;
#9010=CARTESIAN_POINT ( 'NONE',  ( 70.04999999999999716, 11.03553390593273420, 17.50000000000000711 ) ) ;
#9019=CARTESIAN_POINT ( 'NONE',  ( -67.29999999999999716, 9.999999999999998224, 12.49999999999999289 ) ) ;
#9026=CARTESIAN_POINT ( 'NONE',  ( 67.95000000000001705, 7.499999999999996447, 13.96446609406725514 ) ) ;
#9030=CARTESIAN_POINT ( 'NONE',  ( -69.45000000109247651, 12.06698730000000097, 14.99999999999999645 ) ) ;
#9033=CARTESIAN_POINT ( 'NONE',  ( -65.95000000109247651, 8.538419263543524096, 13.53841926354352054 ) ) ;
#9041=CARTESIAN_POINT ( 'NONE',  ( -69.75000000109247367, 8.538419263543522320, 16.46158073645647235 ) ) ;
#9044=CARTESIAN_POINT ( 'NONE',  ( -70.65000000109246514, 9.999999999999998224, 17.06698730000000097 ) ) ;
#9072=CARTESIAN_POINT ( 'NONE',  ( 70.29999999999999716, 7.499999999999996447, 14.99999999999999645 ) ) ;
#9079=FACE_OUTER_BOUND ( 'NONE', #22218, .T. ) ;
#9086=EDGE_LOOP ( 'NONE', ( #20204, #19567, #8361, #19972 ) ) ;
#9096=CARTESIAN_POINT ( 'NONE',  ( 69.55000000218495870, 7.499999999999995559, 16.03553390593273420 ) ) ;
#9109=CARTESIAN_POINT ( 'NONE',  ( 67.00000000218494733, 9.999999999999998224, 17.49999999999999645 ) ) ;
#9111=CARTESIAN_POINT ( 'NONE',  ( -68.09999999999999432, 9.999999999999998224, 12.49999999999999289 ) ) ;
#9118=SURFACE_STYLE_FILL_AREA ( #16523 ) ;
#9124=ORIENTED_EDGE ( 'NONE', *, *, #22569, .F. ) ;
#9128=CARTESIAN_POINT ( 'NONE',  ( 72.50000000000000000, 9.999999999999998224, 12.49999999999999289 ) ) ;
#9140=CARTESIAN_POINT ( 'NONE',  ( -66.29999999999999716, 7.499999999999996447, 14.99999999999999645 ) ) ;
#9151=CARTESIAN_POINT ( 'NONE',  ( -69.20000000109246230, 9.143825827087052716, 12.93301269999999192 ) ) ;
#9154=CARTESIAN_POINT ( 'NONE',  ( -66.15000000109247935, 11.46158073645647235, 13.53841926354352232 ) ) ;
#9164=CARTESIAN_POINT ( 'NONE',  ( -69.35000000109248219, 11.46158073645647235, 13.53841926354352232 ) ) ;
#9166=CARTESIAN_POINT ( 'NONE',  ( -70.70000000109247651, 9.143825827087049163, 17.06698729999999742 ) ) ;
#9196=CARTESIAN_POINT ( 'NONE',  ( 68.74999999999998579, 7.499999999999995559, 13.96446609406725692 ) ) ;
#9222=CARTESIAN_POINT ( 'NONE',  ( 71.55000000109247082, 8.538419263543524096, 13.53841926354352054 ) ) ;
#9229=DIRECTION ( 'NONE',  ( 0.000000000000000000, 0.000000000000000000, -1.000000000000000000 ) ) ;
#9234=VERTEX_POINT ( 'NONE', #7557 ) ;
#9244=ORIENTED_EDGE ( 'NONE', *, *, #22966, .T. ) ;
#9253=( BOUNDED_CURVE ( )  B_SPLINE_CURVE ( 2, ( #19638, #3238, #21185, #4802, #4922, #19526, #3123, #3590, #5398 ),
 .UNSPECIFIED., .F., .F. ) 
 B_SPLINE_CURVE_WITH_KNOTS ( ( 3, 2, 2, 2, 3 ),
 ( 0.5625000000000008882, 0.5781250000000007772, 0.5937500000000006661, 0.6093750000000006661, 0.6250000000000005551 ),
 .UNSPECIFIED. ) 
 CURVE ( )  GEOMETRIC_REPRESENTATION_ITEM ( )  RATIONAL_B_SPLINE_CURVE ( ( 0.9999999999999956701, 0.9238795325112910684, 1.000000000000000000, 0.9238795325112867385, 1.000000000000000000, 0.9238795325112867385, 1.000000000000000000, 0.9238795325112840739, 1.000000000000002665 ) ) 
 REPRESENTATION_ITEM ( '' )  );
#9256=CARTESIAN_POINT ( 'NONE',  ( -67.99999999999998579, 8.232233047033629347, 13.23223304703362402 ) ) ;
#9258=CARTESIAN_POINT ( 'NONE',  ( 72.20000000109246230, 10.85617417291294551, 17.06698729999999742 ) ) ;
#9267=CARTESIAN_POINT ( 'NONE',  ( -67.65000000109247935, 9.999999999999998224, 12.93301269999999192 ) ) ;
#9270=CARTESIAN_POINT ( 'NONE',  ( -70.40000000109247935, 12.06698730000000275, 14.14382582708705094 ) ) ;
#9278=CARTESIAN_POINT ( 'NONE',  ( -70.55000000109247082, 8.538419263543522320, 16.46158073645647235 ) ) ;
#9279=CARTESIAN_POINT ( 'NONE',  ( -71.50000000109247367, 9.143825827087049163, 17.06698729999999742 ) ) ;
#9289=CARTESIAN_POINT ( 'NONE',  ( -71.80000000218494449, 9.999999999999998224, 17.49999999999999645 ) ) ;
#9297=ORIENTED_EDGE ( 'NONE', *, *, #10504, .T. ) ;
#9304=CARTESIAN_POINT ( 'NONE',  ( 69.79999999999999716, 11.76776695296636888, 13.23223304703362579 ) ) ;
#9307=SHAPE_REPRESENTATION ( 'Linear Guide Rail Blocks', ( #7318 ), #14589 ) ;
#9316=DIRECTION ( 'NONE',  ( -1.000000000000000000, -0.000000000000000000, -0.000000000000000000 ) ) ;
#9318=ORIENTED_EDGE ( 'NONE', *, *, #14039, .T. ) ;
#9327=CARTESIAN_POINT ( 'NONE',  ( 71.25000000109248788, 9.999999999999998224, 17.06698730000000097 ) ) ;
#9328=ADVANCED_FACE ( 'NONE', ( #20458 ), #11277, .T. ) ;
#9330=CARTESIAN_POINT ( 'NONE',  ( 71.95000000109247651, 11.46158073645647235, 13.53841926354352232 ) ) ;
#9339=DIRECTION ( 'NONE',  ( 0.000000000000000000, 0.000000000000000000, 1.000000000000000000 ) ) ;
#9340=DIRECTION ( 'NONE',  ( -0.5000000000000013323, 0.000000000000000000, 0.8660254037844380415 ) ) ;
#9349=CARTESIAN_POINT ( 'NONE',  ( 70.64999999999999147, 12.50000000000000000, 13.96446609406725692 ) ) ;
#9362=CARTESIAN_POINT ( 'NONE',  ( 72.25000000109247367, 9.999999999999998224, 17.06698730000000097 ) ) ;
#9367=CARTESIAN_POINT ( 'NONE',  ( 67.05000000109247082, 12.06698730000000097, 14.99999999999999645 ) ) ;
#9373=CARTESIAN_POINT ( 'NONE',  ( -68.20000000218495018, 9.999999999999998224, 12.49999999999999289 ) ) ;
#9375=CARTESIAN_POINT ( 'NONE',  ( -67.15000000218495302, 7.499999999999996447, 16.03553390593273775 ) ) ;
#9377=CARTESIAN_POINT ( 'NONE',  ( -67.80000000109247082, 12.06698729999999919, 14.14382582708705094 ) ) ;
#9380=CARTESIAN_POINT ( 'NONE',  ( -65.75000000109247367, 8.538419263543522320, 16.46158073645647235 ) ) ;
#9389=CARTESIAN_POINT ( 'NONE',  ( -70.80000000109248504, 9.143825827087050939, 12.93301269999999370 ) ) ;
#9391=CARTESIAN_POINT ( 'NONE',  ( -71.05000000109245661, 9.999999999999998224, 12.93301269999999192 ) ) ;
#9403=CARTESIAN_POINT ( 'NONE',  ( 70.15000000218495302, 11.03553390593276973, 17.49999999999997158 ) ) ;
#9414=CARTESIAN_POINT ( 'NONE',  ( 69.09999999999999432, 12.50000000000000000, 14.99999999999999645 ) ) ;
#9419=VECTOR ( 'NONE', #6372, 1000.000000000000000 ) ;
#9420=CARTESIAN_POINT ( 'NONE',  ( 67.14999999999999147, 7.499999999999995559, 13.96446609406725692 ) ) ;
#9428=CARTESIAN_POINT ( 'NONE',  ( -71.20000000109246230, 12.06698729999999919, 14.14382582708705094 ) ) ;
#9433=DIRECTION ( 'NONE',  ( 0.5000000000000013323, 0.000000000000000000, -0.8660254037844380415 ) ) ;
#9434=VERTEX_POINT ( 'NONE', #12228 ) ;
#9440=ORIENTED_EDGE ( 'NONE', *, *, #1612, .T. ) ;
#9442=CARTESIAN_POINT ( 'NONE',  ( 71.90000000109247935, 12.06698730000000275, 15.85617417291294196 ) ) ;
#9445=CARTESIAN_POINT ( 'NONE',  ( 70.25000000109245946, 9.999999999999998224, 12.93301269999999192 ) ) ;
#9453=CARTESIAN_POINT ( 'NONE',  ( -67.35000000109246798, 11.46158073645647235, 16.46158073645647235 ) ) ;
#9458=DIRECTION ( 'NONE',  ( -1.000000000000000000, -0.000000000000000000, -0.000000000000000000 ) ) ;
#9461=EDGE_CURVE ( 'NONE', #15027, #7292, #5016, .T. ) ;
#9473=COLOUR_RGB ( '', 0.40784314, 0.44705882, 0.49803922) ;
#9475=CARTESIAN_POINT ( 'NONE',  ( 70.30000000109247082, 10.85617417291294551, 12.93301269999999192 ) ) ;
#9480=CARTESIAN_POINT ( 'NONE',  ( 66.60000000109248219, 7.933012699999995476, 15.85617417291294196 ) ) ;
#9488=EDGE_LOOP ( 'NONE', ( #6012, #17822, #8021, #22355 ) ) ;
#9491=CARTESIAN_POINT ( 'NONE',  ( -69.60000000109248219, 10.85617417291294551, 17.06698730000000097 ) ) ;
#9494=CARTESIAN_POINT ( 'NONE',  ( -69.30000000109247082, 7.933012699999995476, 14.14382582708705094 ) ) ;
#9507=CARTESIAN_POINT ( 'NONE',  ( -67.95000000109247651, 11.46158073645647235, 16.46158073645647235 ) ) ;
#9508=CARTESIAN_POINT ( 'NONE',  ( 70.45000000109247651, 9.999999999999998224, 17.06698730000000097 ) ) ;
#9510=CARTESIAN_POINT ( 'NONE',  ( -67.50000000109245946, 9.143825827087049163, 17.06698729999999742 ) ) ;
#9514=CARTESIAN_POINT ( 'NONE',  ( 71.70000000000000284, 9.999999999999998224, 17.49999999999999645 ) ) ;
#9543=CARTESIAN_POINT ( 'NONE',  ( 66.99999999999998579, 8.232233047033627571, 16.76776695296636532 ) ) ;
#9551=CARTESIAN_POINT ( 'NONE',  ( -72.05000000109245661, 12.06698730000000097, 14.99999999999999645 ) ) ;
#9559=CARTESIAN_POINT ( 'NONE',  ( -69.65000000109247935, 9.999999999999998224, 17.06698730000000097 ) ) ;
#9573=CARTESIAN_POINT ( 'NONE',  ( 71.50000000109248788, 7.933012699999995476, 14.14382582708705094 ) ) ;
#9576=CARTESIAN_POINT ( 'NONE',  ( 70.35000000109246798, 11.46158073645647235, 13.53841926354352232 ) ) ;
#9582=CARTESIAN_POINT ( 'NONE',  ( 69.00000000218494733, 9.999999999999998224, 12.49999999999999289 ) ) ;
#9588=ORIENTED_EDGE ( 'NONE', *, *, #18040, .F. ) ;
#9603=( BOUNDED_CURVE ( )  B_SPLINE_CURVE ( 2, ( #23240, #21553, #8902, #16198, #1207, #6738, #19765, #8434, #17753 ),
 .UNSPECIFIED., .F., .F. ) 
 B_SPLINE_CURVE_WITH_KNOTS ( ( 3, 2, 2, 2, 3 ),
 ( 0.6250000000000005551, 0.6406250000000004441, 0.6562500000000003331, 0.6718750000000002220, 0.6875000000000001110 ),
 .UNSPECIFIED. ) 
 CURVE ( )  GEOMETRIC_REPRESENTATION_ITEM ( )  RATIONAL_B_SPLINE_CURVE ( ( 0.9999999999999973355, 0.9238795325112894030, 1.000000000000000000, 0.9238795325112867385, 1.000000000000000000, 0.9238795325112867385, 1.000000000000000000, 0.9238795325112861834, 1.000000000000000444 ) ) 
 REPRESENTATION_ITEM ( '' )  );
#9607=LINE ( 'NONE', #13312, #12931 ) ;
#9608=CARTESIAN_POINT ( 'NONE',  ( 71.95000000109247651, 11.46158073645647235, 13.53841926354352232 ) ) ;
#9612=( GEOMETRIC_REPRESENTATION_CONTEXT ( 3 ) GLOBAL_UNCERTAINTY_ASSIGNED_CONTEXT ( ( #4506 ) ) GLOBAL_UNIT_ASSIGNED_CONTEXT ( ( #7670, #99, #22003 ) ) REPRESENTATION_CONTEXT ( 'NONE', 'WORKASPACE' ) );
#9614=CARTESIAN_POINT ( 'NONE',  ( 66.10000000109248219, 10.85617417291294551, 12.93301269999999370 ) ) ;
#9619=CARTESIAN_POINT ( 'NONE',  ( -71.20000000218495018, 7.499999999999996447, 14.99999999999999645 ) ) ;
#9623=CARTESIAN_POINT ( 'NONE',  ( -66.20000000109247651, 12.06698729999999919, 14.14382582708705094 ) ) ;
#9626=CARTESIAN_POINT ( 'NONE',  ( -72.25000000109247367, 9.999999999999998224, 17.06698730000000097 ) ) ;
#9635=CARTESIAN_POINT ( 'NONE',  ( -68.20000000109246230, 7.933012699999995476, 15.85617417291294196 ) ) ;
#9636=CARTESIAN_POINT ( 'NONE',  ( 67.90000000109247935, 12.06698729999999919, 15.85617417291294196 ) ) ;
#9638=CARTESIAN_POINT ( 'NONE',  ( -66.20000000109246230, 9.143825827087050939, 12.93301269999999370 ) ) ;
#9645=ADVANCED_FACE ( 'NONE', ( #7178 ), #12709, .T. ) ;
#9659=CARTESIAN_POINT ( 'NONE',  ( -70.10000000218494165, 11.76776695296636888, 16.76776695296636532 ) ) ;
#9663=CARTESIAN_POINT ( 'NONE',  ( 68.99999999999998579, 11.76776695296636888, 13.23223304703362579 ) ) ;
#9671=CARTESIAN_POINT ( 'NONE',  ( -70.85000000109246798, 7.933012699999995476, 14.99999999999999645 ) ) ;
#9672=CARTESIAN_POINT ( 'NONE',  ( -70.20000000218495018, 9.999999999999998224, 17.49999999999999645 ) ) ;
#9676=CARTESIAN_POINT ( 'NONE',  ( -70.95000000109247651, 11.46158073645647235, 13.53841926354352232 ) ) ;
#9684=CARTESIAN_POINT ( 'NONE',  ( 70.75000000109247367, 8.538419263543524096, 13.53841926354352054 ) ) ;
#9686=CARTESIAN_POINT ( 'NONE',  ( 70.00000000109247367, 7.933012699999995476, 15.85617417291294196 ) ) ;
#9692=CARTESIAN_POINT ( 'NONE',  ( 71.70000000218495018, 11.76776695296636888, 16.76776695296636532 ) ) ;
#9697=CARTESIAN_POINT ( 'NONE',  ( -65.85000000109246798, 9.999999999999998224, 17.06698730000000097 ) ) ;
#9714=CARTESIAN_POINT ( 'NONE',  ( 72.50000000000000000, 9.999999999999998224, 14.99999999999999645 ) ) ;
#9715=CARTESIAN_POINT ( 'NONE',  ( 70.55000000109245661, 11.46158073645647235, 16.46158073645647235 ) ) ;
#9716=ORIENTED_EDGE ( 'NONE', *, *, #906, .T. ) ;
#9722=CARTESIAN_POINT ( 'NONE',  ( 66.00000000109247367, 9.143825827087050939, 12.93301269999999370 ) ) ;
#9733=CARTESIAN_POINT ( 'NONE',  ( -66.05000000109247082, 9.999999999999998224, 12.93301269999999192 ) ) ;
#9736=CARTESIAN_POINT ( 'NONE',  ( -71.15000000109246514, 11.46158073645647235, 13.53841926354352232 ) ) ;
#9745=CARTESIAN_POINT ( 'NONE',  ( -66.35000000109248219, 11.46158073645647235, 16.46158073645647235 ) ) ;
#9746=CARTESIAN_POINT ( 'NONE',  ( 68.95000000109247651, 8.538419263543522320, 16.46158073645647235 ) ) ;
#9747=CARTESIAN_POINT ( 'NONE',  ( -66.55000000109247082, 11.46158073645647235, 16.46158073645647235 ) ) ;
#9748=CARTESIAN_POINT ( 'NONE',  ( -71.54999999999998295, 12.50000000000000000, 16.03553390593273775 ) ) ;
#9750=CARTESIAN_POINT ( 'NONE',  ( 72.15000000109247935, 9.999999999999998224, 17.06698730000000097 ) ) ;
#9763=AXIS2_PLACEMENT_3D ( 'NONE', #3550, #9316, #22085 ) ;
#9765=ADVANCED_FACE ( 'NONE', ( #18522 ), #14846, .F. ) ;
#9766=VECTOR ( 'NONE', #9340, 999.9999999999997726 ) ;
#9769=( BOUNDED_CURVE ( )  B_SPLINE_CURVE ( 2, ( #18243, #9403, #5795, #21836, #21941, #20268, #5550, #11085, #5437 ),
 .UNSPECIFIED., .F., .F. ) 
 B_SPLINE_CURVE_WITH_KNOTS ( ( 3, 2, 2, 2, 3 ),
 ( 0.2500000000000006661, 0.2656250000000005551, 0.2812500000000004441, 0.2968750000000003886, 0.3125000000000002776 ),
 .UNSPECIFIED. ) 
 CURVE ( )  GEOMETRIC_REPRESENTATION_ITEM ( )  RATIONAL_B_SPLINE_CURVE ( ( 0.9999999999999967804, 0.9238795325112899581, 1.000000000000000000, 0.9238795325112867385, 1.000000000000000000, 0.9238795325112867385, 1.000000000000000000, 0.9238795325112854062, 1.000000000000001332 ) ) 
 REPRESENTATION_ITEM ( '' )  );
#9770=CARTESIAN_POINT ( 'NONE',  ( -71.10000000218494165, 8.232233047033627571, 16.76776695296636532 ) ) ;
#9776=CARTESIAN_POINT ( 'NONE',  ( 70.80000000109248504, 9.143825827087050939, 12.93301269999999370 ) ) ;
#9778=CARTESIAN_POINT ( 'NONE',  ( -66.90000000000000568, 9.999999999999998224, 17.49999999999999645 ) ) ;
#9784=CARTESIAN_POINT ( 'NONE',  ( -70.25000000109245946, 9.999999999999998224, 12.93301269999999192 ) ) ;
#9787=DIRECTION ( 'NONE',  ( -1.000000000000000000, -0.000000000000000000, -0.000000000000000000 ) ) ;
#9789=CARTESIAN_POINT ( 'NONE',  ( -71.05000000109247082, 12.06698730000000097, 14.99999999999999645 ) ) ;
#9802=CARTESIAN_POINT ( 'NONE',  ( 69.30000000109247082, 10.85617417291294551, 12.93301269999999370 ) ) ;
#9803=CARTESIAN_POINT ( 'NONE',  ( 69.80000000109247082, 10.85617417291294551, 17.06698729999999742 ) ) ;
#9811=CARTESIAN_POINT ( 'NONE',  ( -66.55000000109247082, 11.46158073645647235, 16.46158073645647235 ) ) ;
#9813=DIRECTION ( 'NONE',  ( -1.000000000000000000, -0.000000000000000000, -0.000000000000000000 ) ) ;
#9817=CARTESIAN_POINT ( 'NONE',  ( -70.79999999999999716, 11.76776695296636888, 16.76776695296636532 ) ) ;
#9823=EDGE_CURVE ( 'NONE', #14025, #14210, #14780, .T. ) ;
#9824=CARTESIAN_POINT ( 'NONE',  ( 71.30000000218494449, 8.232233047033629347, 13.23223304703362402 ) ) ;
#9826=FACE_OUTER_BOUND ( 'NONE', #2038, .T. ) ;
#9827=ORIENTED_EDGE ( 'NONE', *, *, #20775, .T. ) ;
#9828=CARTESIAN_POINT ( 'NONE',  ( 71.90000000109247935, 12.06698729999999919, 15.85617417291294196 ) ) ;
#9831=CARTESIAN_POINT ( 'NONE',  ( 71.75000000218496155, 11.03553390593273598, 17.50000000000000355 ) ) ;
#9835=CARTESIAN_POINT ( 'NONE',  ( 70.70000000109247651, 9.143825827087049163, 17.06698730000000097 ) ) ;
#9839=CARTESIAN_POINT ( 'NONE',  ( 68.80000000109247082, 12.06698730000000275, 14.14382582708705094 ) ) ;
#9849=CARTESIAN_POINT ( 'NONE',  ( -66.55000000109247082, 8.538419263543522320, 16.46158073645647235 ) ) ;
#9851=VECTOR ( 'NONE', #16424, 1000.000000000000000 ) ;
#9853=CARTESIAN_POINT ( 'NONE',  ( -68.55000000109247082, 8.538419263543524096, 13.53841926354352054 ) ) ;
#9856=LINE ( 'NONE', #4212, #9419 ) ;
#9858=EDGE_CURVE ( 'NONE', #19131, #13175, #14200, .T. ) ;
#9866=CARTESIAN_POINT ( 'NONE',  ( -68.50000000109247367, 10.85617417291294551, 12.93301269999999370 ) ) ;
#9867=CARTESIAN_POINT ( 'NONE',  ( 68.30000000109247082, 7.933012699999995476, 14.14382582708705094 ) ) ;
#9868=CARTESIAN_POINT ( 'NONE',  ( -67.30000000109247082, 12.06698730000000275, 15.85617417291294196 ) ) ;
#9872=VECTOR ( 'NONE', #13958, 1000.000000000000000 ) ;
#9892=VERTEX_POINT ( 'NONE', #6998 ) ;
#9893=ADVANCED_FACE ( 'NONE', ( #21576 ), #18014, .T. ) ;
#9895=CARTESIAN_POINT ( 'NONE',  ( -71.55000000218494449, 12.50000000000000000, 13.96446609406725869 ) ) ;
#9903=CARTESIAN_POINT ( 'NONE',  ( 69.10000000109248219, 7.933012699999995476, 14.14382582708705094 ) ) ;
#9915=CARTESIAN_POINT ( 'NONE',  ( -69.55000000109247082, 11.46158073645647235, 16.46158073645647235 ) ) ;
#9925=CARTESIAN_POINT ( 'NONE',  ( 67.35000000109248219, 8.538419263543522320, 16.46158073645647235 ) ) ;
#9927=CARTESIAN_POINT ( 'NONE',  ( 69.35000000109246798, 8.538419263543524096, 13.53841926354352054 ) ) ;
#9941=CARTESIAN_POINT ( 'NONE',  ( -70.89999999999999147, 9.999999999999998224, 17.49999999999999645 ) ) ;
#9951=VERTEX_POINT ( 'NONE', #18592 ) ;
#9954=CARTESIAN_POINT ( 'NONE',  ( 71.30000000109249925, 9.143825827087049163, 17.06698730000000097 ) ) ;
#9956=CARTESIAN_POINT ( 'NONE',  ( 71.05000000218495870, 8.964466094067258695, 17.50000000000000355 ) ) ;
#9960=CARTESIAN_POINT ( 'NONE',  ( 67.05000000109247082, 9.999999999999998224, 12.93301269999999192 ) ) ;
#9967=CARTESIAN_POINT ( 'NONE',  ( 69.05000000109247082, 9.999999999999998224, 17.06698730000000097 ) ) ;
#9980=CARTESIAN_POINT ( 'NONE',  ( -66.30000000109247082, 12.06698729999999919, 15.85617417291294196 ) ) ;
#9982=CARTESIAN_POINT ( 'NONE',  ( -66.50000000109245946, 12.06698730000000275, 15.85617417291294196 ) ) ;
#9992=CARTESIAN_POINT ( 'NONE',  ( -66.90000000109246514, 10.85617417291294551, 12.93301269999999370 ) ) ;
#9995=CARTESIAN_POINT ( 'NONE',  ( 68.75000000109247367, 11.46158073645647235, 16.46158073645647235 ) ) ;
#9996=CARTESIAN_POINT ( 'NONE',  ( -67.90000000109245093, 10.85617417291294551, 12.93301269999999370 ) ) ;
#10008=ORIENTED_EDGE ( 'NONE', *, *, #5733, .T. ) ;
#10019=CARTESIAN_POINT ( 'NONE',  ( -72.50000000000000000, 9.999999999999998224, 14.99999999999999645 ) ) ;
#10022=CARTESIAN_POINT ( 'NONE',  ( -69.25000000218494733, 12.50000000000000000, 16.03553390593273420 ) ) ;
#10026=( BOUNDED_CURVE ( )  B_SPLINE_CURVE ( 2, ( #12021, #6727, #8649, #23231, #6499, #2995, #14037, #10586, #12135 ),
 .UNSPECIFIED., .F., .F. ) 
 B_SPLINE_CURVE_WITH_KNOTS ( ( 3, 2, 2, 2, 3 ),
 ( 0.7499999999999997780, 0.7656249999999996669, 0.7812499999999995559, 0.7968749999999994449, 0.8124999999999993339 ),
 .UNSPECIFIED. ) 
 CURVE ( )  GEOMETRIC_REPRESENTATION_ITEM ( )  RATIONAL_B_SPLINE_CURVE ( ( 1.000000000000001110, 0.9238795325112856283, 1.000000000000000000, 0.9238795325112867385, 1.000000000000000000, 0.9238795325112867385, 1.000000000000000000, 0.9238795325112899581, 0.9999999999999967804 ) ) 
 REPRESENTATION_ITEM ( '' )  );
#10029=CARTESIAN_POINT ( 'NONE',  ( 70.00000000109248788, 9.143825827087050939, 12.93301269999999370 ) ) ;
#10034=ADVANCED_FACE ( 'NONE', ( #20618 ), #258, .F. ) ;
#10036=CARTESIAN_POINT ( 'NONE',  ( -69.55000000109247082, 11.46158073645647235, 13.53841926354352232 ) ) ;
#10038=CARTESIAN_POINT ( 'NONE',  ( -69.80000000218494449, 9.999999999999998224, 12.49999999999999289 ) ) ;
#10041=DIRECTION ( 'NONE',  ( 0.000000000000000000, 0.000000000000000000, 1.000000000000000000 ) ) ;
#10042=CARTESIAN_POINT ( 'NONE',  ( 72.50000000000000000, 9.999999999999998224, 14.99999999999999645 ) ) ;
#10050=CARTESIAN_POINT ( 'NONE',  ( 67.80000000109247082, 12.06698730000000275, 14.14382582708705094 ) ) ;
#10051=CARTESIAN_POINT ( 'NONE',  ( 69.60000000109248219, 12.06698730000000275, 14.14382582708705094 ) ) ;
#10079=CARTESIAN_POINT ( 'NONE',  ( 68.95000000109247651, 11.46158073645647235, 16.46158073645647235 ) ) ;
#10083=CARTESIAN_POINT ( 'NONE',  ( 70.50000000109245946, 12.06698730000000275, 15.85617417291294196 ) ) ;
#10093=CARTESIAN_POINT ( 'NONE',  ( -67.05000000109247082, 12.06698730000000097, 14.99999999999999645 ) ) ;
#10095=CARTESIAN_POINT ( 'NONE',  ( -66.90000000109246514, 7.933012699999995476, 14.14382582708705094 ) ) ;
#10109=CARTESIAN_POINT ( 'NONE',  ( -70.29999999999999716, 7.499999999999996447, 14.99999999999999645 ) ) ;
#10126=CARTESIAN_POINT ( 'NONE',  ( 72.50000000000000000, 9.999999999999998224, 14.99999999999999645 ) ) ;
#10130=LINE ( 'NONE', #11938, #23655 ) ;
#10134=CARTESIAN_POINT ( 'NONE',  ( -68.85000000218495586, 7.499999999999995559, 13.96446609406725692 ) ) ;
#10135=EDGE_CURVE ( 'NONE', #1904, #15027, #21295, .T. ) ;
#10141=VECTOR ( 'NONE', #8084, 1000.000000000000000 ) ;
#10143=CARTESIAN_POINT ( 'NONE',  ( 69.00000000109247367, 7.933012699999995476, 15.85617417291294196 ) ) ;
#10144=CYLINDRICAL_SURFACE ( 'NONE', #11104, 2.500000000000002220 ) ;
#10149=CARTESIAN_POINT ( 'NONE',  ( -67.65000000109247935, 7.933012699999995476, 14.99999999999999645 ) ) ;
#10161=CARTESIAN_POINT ( 'NONE',  ( -66.84999999999999432, 11.03553390593268624, 17.50000000000005329 ) ) ;
#10166=CARTESIAN_POINT ( 'NONE',  ( 67.55000000109247082, 8.538419263543524096, 13.53841926354352054 ) ) ;
#10170=CARTESIAN_POINT ( 'NONE',  ( 68.35000000109246798, 8.538419263543522320, 16.46158073645647235 ) ) ;
#10177=CYLINDRICAL_SURFACE ( 'NONE', #19698, 2.500000000000002220 ) ;
#10188=CARTESIAN_POINT ( 'NONE',  ( -70.80000000218494449, 12.50000000000000000, 14.99999999999999645 ) ) ;
#10190=CARTESIAN_POINT ( 'NONE',  ( -69.70000000000000284, 9.999999999999998224, 12.49999999999999289 ) ) ;
#10193=CARTESIAN_POINT ( 'NONE',  ( 70.40000000218495302, 7.499999999999996447, 14.99999999999999645 ) ) ;
#10198=CARTESIAN_POINT ( 'NONE',  ( 67.50000000109245946, 9.143825827087049163, 17.06698730000000097 ) ) ;
#10201=CARTESIAN_POINT ( 'NONE',  ( -68.70000000218495018, 8.232233047033627571, 16.76776695296636532 ) ) ;
#10203=CARTESIAN_POINT ( 'NONE',  ( 68.40000000109246514, 7.933012699999995476, 15.85617417291294196 ) ) ;
#10205=CYLINDRICAL_SURFACE ( 'NONE', #1316, 2.500000000000002220 ) ;
#10216=CARTESIAN_POINT ( 'NONE',  ( -68.85000000109246798, 12.06698730000000097, 14.99999999999999645 ) ) ;
#10224=CARTESIAN_POINT ( 'NONE',  ( 67.30000000109247082, 9.143825827087049163, 17.06698730000000097 ) ) ;
#10225=CARTESIAN_POINT ( 'NONE',  ( -71.00000000000000000, 8.232233047033627571, 16.76776695296636532 ) ) ;
#10251=CARTESIAN_POINT ( 'NONE',  ( -66.55000000218494449, 8.964466094067258695, 12.49999999999999289 ) ) ;
#10259=CARTESIAN_POINT ( 'NONE',  ( 68.65000000109247935, 12.06698730000000097, 14.99999999999999645 ) ) ;
#10268=CARTESIAN_POINT ( 'NONE',  ( -69.70000000109247651, 12.06698729999999919, 15.85617417291294196 ) ) ;
#10269=ORIENTED_EDGE ( 'NONE', *, *, #7446, .F. ) ;
#10278=ORIENTED_EDGE ( 'NONE', *, *, #19457, .T. ) ;
#10286=CARTESIAN_POINT ( 'NONE',  ( 69.40000000109249356, 12.06698730000000275, 14.14382582708705094 ) ) ;
#10287=CARTESIAN_POINT ( 'NONE',  ( 69.45000000109247651, 9.999999999999998224, 12.93301269999999192 ) ) ;
#10308=CARTESIAN_POINT ( 'NONE',  ( 71.40000000109249356, 7.933012699999995476, 15.85617417291294196 ) ) ;
#10315=CARTESIAN_POINT ( 'NONE',  ( 70.85000000218494165, 12.50000000000000000, 16.03553390593273420 ) ) ;
#10319=CARTESIAN_POINT ( 'NONE',  ( 66.55000000109247082, 11.46158073645647235, 16.46158073645647235 ) ) ;
#10324=CARTESIAN_POINT ( 'NONE',  ( 69.80000000109247082, 10.85617417291294551, 17.06698729999999742 ) ) ;
#10339=CARTESIAN_POINT ( 'NONE',  ( -67.75000000109245946, 8.538419263543524096, 13.53841926354352054 ) ) ;
#10351=CARTESIAN_POINT ( 'NONE',  ( 67.50000000109247367, 7.933012699999995476, 14.14382582708705094 ) ) ;
#10352=CARTESIAN_POINT ( 'NONE',  ( -69.25000000000000000, 11.03553390593273598, 17.50000000000000355 ) ) ;
#10362=ORIENTED_EDGE ( 'NONE', *, *, #20233, .T. ) ;
#10366=CARTESIAN_POINT ( 'NONE',  ( -69.15000000109247935, 8.538419263543524096, 13.53841926354352054 ) ) ;
#10367=FACE_OUTER_BOUND ( 'NONE', #23324, .T. ) ;
#10373=DIRECTION ( 'NONE',  ( -1.000000000000000000, -0.000000000000000000, -0.000000000000000000 ) ) ;
#10377=CARTESIAN_POINT ( 'NONE',  ( -65.90000000218495302, 11.76776695296636888, 13.23223304703362579 ) ) ;
#10378=( BOUNDED_CURVE ( )  B_SPLINE_CURVE ( 2, ( #13882, #17810, #22831, #4753, #12089, #21377, #8716, #17347, #2829 ),
 .UNSPECIFIED., .F., .F. ) 
 B_SPLINE_CURVE_WITH_KNOTS ( ( 3, 2, 2, 2, 3 ),
 ( 0.5625000000000008882, 0.5781250000000007772, 0.5937500000000006661, 0.6093750000000006661, 0.6250000000000005551 ),
 .UNSPECIFIED. ) 
 CURVE ( )  GEOMETRIC_REPRESENTATION_ITEM ( )  RATIONAL_B_SPLINE_CURVE ( ( 0.9999999999999956701, 0.9238795325112910684, 1.000000000000000000, 0.9238795325112867385, 1.000000000000000000, 0.9238795325112867385, 1.000000000000000000, 0.9238795325112840739, 1.000000000000002665 ) ) 
 REPRESENTATION_ITEM ( '' )  );
#10388=COLOUR_RGB ( '', 0.40784314, 0.44705882, 0.49803922) ;
#10393=CARTESIAN_POINT ( 'NONE',  ( -67.70000000109247651, 7.933012699999995476, 14.14382582708705094 ) ) ;
#10401=ORIENTED_EDGE ( 'NONE', *, *, #4205, .T. ) ;
#10404=ORIENTED_EDGE ( 'NONE', *, *, #20775, .F. ) ;
#10408=CARTESIAN_POINT ( 'NONE',  ( -69.60000000218495586, 7.499999999999996447, 14.99999999999999645 ) ) ;
#10411=CARTESIAN_POINT ( 'NONE',  ( 69.65000000109246514, 12.06698730000000097, 14.99999999999999645 ) ) ;
#10435=CARTESIAN_POINT ( 'NONE',  ( 67.35000000218495586, 8.964466094067258695, 12.49999999999999289 ) ) ;
#10438=CARTESIAN_POINT ( 'NONE',  ( 68.90000000109246514, 12.06698729999999919, 15.85617417291294196 ) ) ;
#10444=CARTESIAN_POINT ( 'NONE',  ( 67.90000000109245093, 10.85617417291294551, 12.93301269999999370 ) ) ;
#10464=CARTESIAN_POINT ( 'NONE',  ( 66.20000000109247651, 12.06698729999999919, 14.14382582708705094 ) ) ;
#10467=EDGE_CURVE ( 'NONE', #13655, #7935, #18741, .T. ) ;
#10468=CARTESIAN_POINT ( 'NONE',  ( -70.05000000000002558, 11.03553390593273598, 17.50000000000000355 ) ) ;
#10480=CARTESIAN_POINT ( 'NONE',  ( -66.30000000109247082, 12.06698730000000275, 15.85617417291294196 ) ) ;
#10487=ORIENTED_EDGE ( 'NONE', *, *, #12762, .T. ) ;
#10491=CARTESIAN_POINT ( 'NONE',  ( -68.55000000218495870, 11.03553390593273598, 17.50000000000000355 ) ) ;
#10497=DIRECTION ( 'NONE',  ( -1.000000000000000000, -0.000000000000000000, -0.000000000000000000 ) ) ;
#10504=EDGE_CURVE ( 'NONE', #14810, #1264, #11047, .T. ) ;
#10505=ORIENTED_EDGE ( 'NONE', *, *, #1635, .T. ) ;
#10509=DIRECTION ( 'NONE',  ( 1.000000000000000000, 0.000000000000000000, 0.000000000000000000 ) ) ;
#10511=DIRECTION ( 'NONE',  ( 1.000000000000000000, 0.000000000000000000, 0.000000000000000000 ) ) ;
#10512=ORIENTED_EDGE ( 'NONE', *, *, #15530, .T. ) ;
#10516=( BOUNDED_CURVE ( )  B_SPLINE_CURVE ( 2, ( #13357, #14925, #7603, #5793, #11204, #5911, #7835, #15156, #18367 ),
 .UNSPECIFIED., .F., .F. ) 
 B_SPLINE_CURVE_WITH_KNOTS ( ( 3, 2, 2, 2, 3 ),
 ( 0.3749999999999998890, 0.3906249999999997780, 0.4062499999999996669, 0.4218749999999996114, 0.4374999999999995004 ),
 .UNSPECIFIED. ) 
 CURVE ( )  GEOMETRIC_REPRESENTATION_ITEM ( )  RATIONAL_B_SPLINE_CURVE ( ( 1.000000000000000444, 0.9238795325112861834, 1.000000000000000000, 0.9238795325112867385, 1.000000000000000000, 0.9238795325112867385, 1.000000000000000000, 0.9238795325112891810, 0.9999999999999975575 ) ) 
 REPRESENTATION_ITEM ( '' )  );
#10520=CARTESIAN_POINT ( 'NONE',  ( -69.65000000218496723, 7.499999999999996447, 13.96446609406725514 ) ) ;
#10525=CARTESIAN_POINT ( 'NONE',  ( 71.54999999999999716, 12.50000000000000000, 16.03553390593273420 ) ) ;
#10542=CARTESIAN_POINT ( 'NONE',  ( -67.70000000000000284, 9.999999999999998224, 17.49999999999999645 ) ) ;
#10545=ORIENTED_EDGE ( 'NONE', *, *, #4767, .F. ) ;
#10546=CARTESIAN_POINT ( 'NONE',  ( -68.45000000218495018, 12.50000000000000000, 16.03553390593273775 ) ) ;
#10552=CARTESIAN_POINT ( 'NONE',  ( 68.40000000218495302, 12.50000000000000000, 14.99999999999999645 ) ) ;
#10560=CARTESIAN_POINT ( 'NONE',  ( 67.55000000109247082, 8.538419263543522320, 16.46158073645647235 ) ) ;
#10582=ORIENTED_EDGE ( 'NONE', *, *, #7963, .F. ) ;
#10584=CARTESIAN_POINT ( 'NONE',  ( -66.15000000000000568, 8.964466094067260471, 17.50000000000000355 ) ) ;
#10585=VECTOR ( 'NONE', #11427, 1000.000000000000000 ) ;
#10586=CARTESIAN_POINT ( 'NONE',  ( -66.65000000218496723, 11.03553390593276973, 12.50000000000002665 ) ) ;
#10590=CARTESIAN_POINT ( 'NONE',  ( -70.34999999999999432, 7.499999999999995559, 13.96446609406725692 ) ) ;
#10603=CARTESIAN_POINT ( 'NONE',  ( -67.60000000109248219, 9.143825827087050939, 12.93301269999999370 ) ) ;
#10605=EDGE_CURVE ( 'NONE', #3718, #23046, #17179, .T. ) ;
#10608=CARTESIAN_POINT ( 'NONE',  ( -71.40000000218495302, 9.999999999999998224, 12.49999999999999289 ) ) ;
#10614=CARTESIAN_POINT ( 'NONE',  ( -68.20000000218495018, 9.999999999999998224, 12.49999999999999289 ) ) ;
#10639=DIRECTION ( 'NONE',  ( -1.000000000000000000, -0.000000000000000000, -0.000000000000000000 ) ) ;
#10640=ORIENTED_EDGE ( 'NONE', *, *, #18126, .T. ) ;
#10644=CARTESIAN_POINT ( 'NONE',  ( 71.05000000000001137, 7.499999999999995559, 16.03553390593273420 ) ) ;
#10645=CARTESIAN_POINT ( 'NONE',  ( -65.75000000218494733, 8.964466094067219615, 12.50000000000003553 ) ) ;
#10667=CARTESIAN_POINT ( 'NONE',  ( 68.10000000218495586, 8.232233047033629347, 13.23223304703362402 ) ) ;
#10678=CARTESIAN_POINT ( 'NONE',  ( 67.45000000109246230, 9.999999999999998224, 17.06698730000000097 ) ) ;
#10686=DIRECTION ( 'NONE',  ( 0.000000000000000000, 0.000000000000000000, 1.000000000000000000 ) ) ;
#10703=CARTESIAN_POINT ( 'NONE',  ( -67.39999999999999147, 11.76776695296636888, 13.23223304703362579 ) ) ;
#10705=CARTESIAN_POINT ( 'NONE',  ( 66.60000000218495586, 9.999999999999998224, 12.49999999999999289 ) ) ;
#10711=CARTESIAN_POINT ( 'NONE',  ( 67.15000000218495302, 7.499999999999996447, 16.03553390593273775 ) ) ;
#10712=CARTESIAN_POINT ( 'NONE',  ( 68.45000000218495018, 12.50000000000000000, 16.03553390593273775 ) ) ;
#10714=CARTESIAN_POINT ( 'NONE',  ( -66.40000000218495302, 7.499999999999996447, 14.99999999999999645 ) ) ;
#10716=CARTESIAN_POINT ( 'NONE',  ( -71.35000000109246798, 8.538419263543522320, 16.46158073645647235 ) ) ;
#10719=CARTESIAN_POINT ( 'NONE',  ( -68.70000000109246230, 12.06698730000000275, 15.85617417291294196 ) ) ;
#10722=DIRECTION ( 'NONE',  ( 0.000000000000000000, 0.000000000000000000, 1.000000000000000000 ) ) ;
#10728=CARTESIAN_POINT ( 'NONE',  ( 71.04999999999999716, 7.499999999999996447, 16.03553390593273775 ) ) ;
#10731=CARTESIAN_POINT ( 'NONE',  ( -71.55000000109247082, 8.538419263543524096, 13.53841926354352054 ) ) ;
#10747=CARTESIAN_POINT ( 'NONE',  ( 70.45000000218495018, 7.499999999999996447, 13.96446609406725514 ) ) ;
#10751=ORIENTED_EDGE ( 'NONE', *, *, #6266, .T. ) ;
#10758=CARTESIAN_POINT ( 'NONE',  ( 69.05000000000002558, 12.50000000000000000, 13.96446609406725692 ) ) ;
#10765=CARTESIAN_POINT ( 'NONE',  ( 70.64999999999999147, 12.50000000000000000, 13.96446609406725869 ) ) ;
#10769=CARTESIAN_POINT ( 'NONE',  ( 69.70000000218495018, 8.232233047033629347, 13.23223304703362402 ) ) ;
#10788=CARTESIAN_POINT ( 'NONE',  ( 66.80000000218494449, 12.50000000000000000, 14.99999999999999645 ) ) ;
#10795=( BOUNDED_CURVE ( )  B_SPLINE_CURVE ( 2, ( #8767, #3480, #18089, #21788, #16421, #6840, #12735, #10584, #19756 ),
 .UNSPECIFIED., .F., .F. ) 
 B_SPLINE_CURVE_WITH_KNOTS ( ( 3, 2, 2, 2, 3 ),
 ( 0.9375000000000007772, 0.9531250000000005551, 0.9687500000000004441, 0.9843750000000002220, 1.000000000000000000 ),
 .UNSPECIFIED. ) 
 CURVE ( )  GEOMETRIC_REPRESENTATION_ITEM ( )  RATIONAL_B_SPLINE_CURVE ( ( 0.9999999999999962252, 0.9238795325112905132, 1.000000000000000000, 0.9238795325112867385, 1.000000000000000000, 0.9238795325112867385, 1.000000000000000000, 0.9238795325112867385, 1.000000000000000000 ) ) 
 REPRESENTATION_ITEM ( '' )  );
#10799=CARTESIAN_POINT ( 'NONE',  ( -72.37500000054622262, 9.999999999999998224, 17.28349365000000049 ) ) ;
#10821=CARTESIAN_POINT ( 'NONE',  ( -66.40000000000000568, 8.232233047033629347, 13.23223304703362402 ) ) ;
#10832=CARTESIAN_POINT ( 'NONE',  ( -71.80000000109247082, 12.06698729999999919, 14.14382582708705094 ) ) ;
#10835=CARTESIAN_POINT ( 'NONE',  ( -68.15000000109247935, 8.538419263543522320, 16.46158073645647235 ) ) ;
#10837=EDGE_CURVE ( 'NONE', #3012, #9892, #1651, .T. ) ;
#10844=CARTESIAN_POINT ( 'NONE',  ( -69.95000000109247651, 8.538419263543524096, 13.53841926354352054 ) ) ;
#10845=CARTESIAN_POINT ( 'NONE',  ( -70.25000000109245946, 9.999999999999998224, 12.93301269999999192 ) ) ;
#10866=CARTESIAN_POINT ( 'NONE',  ( 72.50000000000000000, 9.999999999999998224, 14.99999999999999645 ) ) ;
#10872=ORIENTED_EDGE ( 'NONE', *, *, #6434, .T. ) ;
#10873=CARTESIAN_POINT ( 'NONE',  ( 65.75000000109247367, 8.538419263543522320, 16.46158073645647235 ) ) ;
#10874=CARTESIAN_POINT ( 'NONE',  ( 72.39999999999999147, 11.76776695296636888, 16.76776695296636532 ) ) ;
#10876=CARTESIAN_POINT ( 'NONE',  ( 69.29999999999999716, 9.999999999999998224, 17.49999999999999645 ) ) ;
#10893=LINE ( 'NONE', #11240, #17569 ) ;
#10897=CARTESIAN_POINT ( 'NONE',  ( 69.50000000218494733, 8.232233047033627571, 16.76776695296636532 ) ) ;
#10907=CARTESIAN_POINT ( 'NONE',  ( 66.05000000109247082, 7.933012699999995476, 14.99999999999999645 ) ) ;
#10908=CARTESIAN_POINT ( 'NONE',  ( 72.50000000000000000, 9.999999999999998224, 17.49999999999999645 ) ) ;
#10909=CARTESIAN_POINT ( 'NONE',  ( -68.89999999999999147, 9.999999999999998224, 12.49999999999999289 ) ) ;
#10914=( LENGTH_UNIT ( ) NAMED_UNIT ( * ) SI_UNIT ( .MILLI., .METRE. ) );
#10942=CARTESIAN_POINT ( 'NONE',  ( -69.75000000109247367, 8.538419263543522320, 16.46158073645647235 ) ) ;
#10945=CARTESIAN_POINT ( 'NONE',  ( -68.95000000109247651, 8.538419263543522320, 16.46158073645647235 ) ) ;
#10947=CARTESIAN_POINT ( 'NONE',  ( 72.50000000000000000, 9.999999999999998224, 17.49999999999999645 ) ) ;
#10954=CARTESIAN_POINT ( 'NONE',  ( -71.70000000109247651, 10.85617417291294551, 12.93301269999999370 ) ) ;
#10957=CARTESIAN_POINT ( 'NONE',  ( -68.85000000109246798, 12.06698730000000097, 14.99999999999999645 ) ) ;
#10977=CARTESIAN_POINT ( 'NONE',  ( 69.14999999999999147, 12.50000000000000000, 16.03553390593273775 ) ) ;
#10983=CARTESIAN_POINT ( 'NONE',  ( 69.99999999999998579, 11.76776695296636888, 16.76776695296636532 ) ) ;
#10986=CARTESIAN_POINT ( 'NONE',  ( 69.60000000218495586, 7.499999999999996447, 14.99999999999999645 ) ) ;
#11003=ORIENTED_EDGE ( 'NONE', *, *, #22832, .T. ) ;
#11008=CARTESIAN_POINT ( 'NONE',  ( 72.00000000109248788, 10.85617417291294551, 17.06698729999999742 ) ) ;
#11019=FACE_OUTER_BOUND ( 'NONE', #21135, .T. ) ;
#11020=VECTOR ( 'NONE', #16499, 1000.000000000000000 ) ;
#11021=CARTESIAN_POINT ( 'NONE',  ( -68.89999999999999147, 9.999999999999998224, 12.49999999999999289 ) ) ;
#11035=CARTESIAN_POINT ( 'NONE',  ( 69.89999999999999147, 12.50000000000000000, 14.99999999999999645 ) ) ;
#11045=CARTESIAN_POINT ( 'NONE',  ( -68.64999999999999147, 7.499999999999995559, 16.03553390593273420 ) ) ;
#11047=LINE ( 'NONE', #16903, #15297 ) ;
#11049=CARTESIAN_POINT ( 'NONE',  ( 67.85000000109248219, 12.06698730000000097, 14.99999999999999645 ) ) ;
#11054=CARTESIAN_POINT ( 'NONE',  ( 68.20000000218495018, 9.999999999999998224, 12.49999999999999289 ) ) ;
#11059=CARTESIAN_POINT ( 'NONE',  ( -69.50000000109247367, 12.06698729999999919, 15.85617417291294196 ) ) ;
#11062=CARTESIAN_POINT ( 'NONE',  ( -70.50000000109245946, 12.06698730000000275, 15.85617417291294196 ) ) ;
#11068=CARTESIAN_POINT ( 'NONE',  ( 70.89999999999999147, 9.999999999999998224, 17.49999999999999645 ) ) ;
#11072=CARTESIAN_POINT ( 'NONE',  ( -71.15000000109247935, 11.46158073645647235, 16.46158073645647235 ) ) ;
#11073=CARTESIAN_POINT ( 'NONE',  ( -71.00000000109245946, 9.143825827087050939, 12.93301269999999370 ) ) ;
#11085=CARTESIAN_POINT ( 'NONE',  ( 69.85000000218497007, 11.03553390593272177, 12.49999999999998046 ) ) ;
#11086=CARTESIAN_POINT ( 'NONE',  ( 72.50000000000000000, 9.999999999999998224, 17.49999999999999645 ) ) ;
#11102=EDGE_CURVE ( 'NONE', #14363, #20225, #3481, .T. ) ;
#11104=AXIS2_PLACEMENT_3D ( 'NONE', #6415, #6294, #17436 ) ;
#11105=CARTESIAN_POINT ( 'NONE',  ( 69.20000000000000284, 11.76776695296636888, 16.76776695296636532 ) ) ;
#11108=CARTESIAN_POINT ( 'NONE',  ( -66.94999999999998863, 8.964466094067207180, 17.49999999999995026 ) ) ;
#11114=DIRECTION ( 'NONE',  ( -1.000000000000000000, -0.000000000000000000, -0.000000000000000000 ) ) ;
#11121=AXIS2_PLACEMENT_3D ( 'NONE', #20259, #7366, #5905 ) ;
#11135=CARTESIAN_POINT ( 'NONE',  ( 71.85000000109246798, 12.06698730000000097, 14.99999999999999645 ) ) ;
#11136=CARTESIAN_POINT ( 'NONE',  ( 66.15000000000000568, 8.964466094067260471, 17.50000000000000355 ) ) ;
#11138=CARTESIAN_POINT ( 'NONE',  ( 72.15000000109246514, 11.46158073645647235, 16.46158073645647235 ) ) ;
#11146=CARTESIAN_POINT ( 'NONE',  ( -67.70000000000000284, 9.999999999999998224, 17.49999999999999645 ) ) ;
#11167=VECTOR ( 'NONE', #8281, 1000.000000000000000 ) ;
#11175=CARTESIAN_POINT ( 'NONE',  ( 72.25000000109247367, 9.999999999999998224, 17.06698730000000097 ) ) ;
#11182=CARTESIAN_POINT ( 'NONE',  ( -67.25000000218494733, 7.499999999999996447, 13.96446609406725514 ) ) ;
#11184=CARTESIAN_POINT ( 'NONE',  ( -70.35000000109248219, 11.46158073645647235, 16.46158073645647235 ) ) ;
#11187=CARTESIAN_POINT ( 'NONE',  ( -69.70000000109246230, 12.06698730000000275, 15.85617417291294196 ) ) ;
#11196=CARTESIAN_POINT ( 'NONE',  ( -71.75000000109248788, 11.46158073645647235, 13.53841926354352232 ) ) ;
#11197=CARTESIAN_POINT ( 'NONE',  ( -71.45000000109247651, 9.999999999999998224, 17.06698730000000097 ) ) ;
#11204=CARTESIAN_POINT ( 'NONE',  ( -69.20000000218495018, 12.50000000000000000, 14.99999999999999645 ) ) ;
#11206=CARTESIAN_POINT ( 'NONE',  ( 70.14999999999999147, 8.964466094067256918, 17.49999999999999289 ) ) ;
#11207=CARTESIAN_POINT ( 'NONE',  ( -71.55000000218494449, 12.50000000000000000, 13.96446609406725692 ) ) ;
#11220=CARTESIAN_POINT ( 'NONE',  ( 67.29999999999999716, 9.999999999999998224, 12.49999999999999289 ) ) ;
#11228=CARTESIAN_POINT ( 'NONE',  ( 68.90000000218495302, 8.232233047033629347, 13.23223304703362402 ) ) ;
#11229=CARTESIAN_POINT ( 'NONE',  ( -71.25000000109247367, 12.06698730000000097, 14.99999999999999645 ) ) ;
#11237=CARTESIAN_POINT ( 'NONE',  ( 72.50000000000000000, 9.999999999999998224, 17.49999999999999645 ) ) ;
#11240=CARTESIAN_POINT ( 'NONE',  ( 72.50000000000000000, 9.999999999999998224, 12.49999999999999289 ) ) ;
#11245=CARTESIAN_POINT ( 'NONE',  ( 66.00000000218494733, 12.50000000000000000, 14.99999999999999645 ) ) ;
#11247=CARTESIAN_POINT ( 'NONE',  ( 70.50000000109245946, 12.06698730000000275, 15.85617417291294196 ) ) ;
#11265=ORIENTED_EDGE ( 'NONE', *, *, #22086, .F. ) ;
#11270=ORIENTED_EDGE ( 'NONE', *, *, #1910, .T. ) ;
#11274=( BOUNDED_CURVE ( )  B_SPLINE_CURVE ( 2, ( #7550, #9010, #19982, #5747, #11035, #3585, #16302, #105, #14519 ),
 .UNSPECIFIED., .F., .F. ) 
 B_SPLINE_CURVE_WITH_KNOTS ( ( 3, 2, 2, 2, 3 ),
 ( 0.3749999999999998890, 0.3906249999999997780, 0.4062499999999996669, 0.4218749999999996114, 0.4374999999999995004 ),
 .UNSPECIFIED. ) 
 CURVE ( )  GEOMETRIC_REPRESENTATION_ITEM ( )  RATIONAL_B_SPLINE_CURVE ( ( 1.000000000000000444, 0.9238795325112861834, 1.000000000000000000, 0.9238795325112867385, 1.000000000000000000, 0.9238795325112867385, 1.000000000000000000, 0.9238795325112891810, 0.9999999999999975575 ) ) 
 REPRESENTATION_ITEM ( '' )  );
#11277=CYLINDRICAL_SURFACE ( 'NONE', #12641, 2.500000000000002220 ) ;
#11279=CARTESIAN_POINT ( 'NONE',  ( 71.80000000109245661, 9.143825827087052716, 12.93301269999999192 ) ) ;
#11282=EDGE_CURVE ( 'NONE', #9434, #23552, #21158, .T. ) ;
#11287=CARTESIAN_POINT ( 'NONE',  ( 67.10000000109248219, 12.06698730000000275, 15.85617417291294196 ) ) ;
#11299=CARTESIAN_POINT ( 'NONE',  ( -67.85000000109248219, 12.06698730000000097, 14.99999999999999645 ) ) ;
#11302=CARTESIAN_POINT ( 'NONE',  ( -69.35000000109246798, 8.538419263543524096, 13.53841926354352054 ) ) ;
#11312=CARTESIAN_POINT ( 'NONE',  ( -68.30000000109247082, 7.933012699999995476, 14.14382582708705094 ) ) ;
#11314=CARTESIAN_POINT ( 'NONE',  ( 68.45000000109247651, 9.999999999999998224, 12.93301269999999192 ) ) ;
#11315=CARTESIAN_POINT ( 'NONE',  ( -68.60000000109246798, 9.143825827087050939, 12.93301269999999370 ) ) ;
#11320=CARTESIAN_POINT ( 'NONE',  ( 71.84999999999999432, 7.499999999999996447, 16.03553390593273775 ) ) ;
#11328=ORIENTED_EDGE ( 'NONE', *, *, #13379, .F. ) ;
#11344=DIRECTION ( 'NONE',  ( -1.000000000000000000, -0.000000000000000000, -0.000000000000000000 ) ) ;
#11346=CARTESIAN_POINT ( 'NONE',  ( 68.64999999999999147, 7.499999999999995559, 16.03553390593273420 ) ) ;
#11347=CYLINDRICAL_SURFACE ( 'NONE', #16974, 2.500000000000002220 ) ;
#11358=CARTESIAN_POINT ( 'NONE',  ( -71.25000000109248788, 9.999999999999998224, 17.06698730000000097 ) ) ;
#11359=EDGE_LOOP ( 'NONE', ( #12694, #5707, #4385, #7868 ) ) ;
#11367=CARTESIAN_POINT ( 'NONE',  ( 65.65000000218493881, 7.499999999999995559, 13.96446609406725692 ) ) ;
#11369=CARTESIAN_POINT ( 'NONE',  ( 70.15000000109246514, 8.538419263543524096, 13.53841926354352054 ) ) ;
#11382=FILL_AREA_STYLE_COLOUR ( '', #10388 ) ;
#11401=CARTESIAN_POINT ( 'NONE',  ( 71.90000000109246514, 10.85617417291294551, 12.93301269999999192 ) ) ;
#11407=DIRECTION ( 'NONE',  ( 1.000000000000000000, 0.000000000000000000, 0.000000000000000000 ) ) ;
#11408=CARTESIAN_POINT ( 'NONE',  ( 67.95000000109247651, 11.46158073645647235, 16.46158073645647235 ) ) ;
#11423=CARTESIAN_POINT ( 'NONE',  ( -70.85000000109246798, 7.933012699999995476, 14.99999999999999645 ) ) ;
#11425=( BOUNDED_CURVE ( )  B_SPLINE_CURVE ( 2, ( #19141, #8025, #22728, #5977, #10188, #22845, #11635, #6095, #2605 ),
 .UNSPECIFIED., .F., .F. ) 
 B_SPLINE_CURVE_WITH_KNOTS ( ( 3, 2, 2, 2, 3 ),
 ( 0.1249999999999992367, 0.1406249999999996947, 0.1562500000000001388, 0.1718750000000005829, 0.1875000000000010270 ),
 .UNSPECIFIED. ) 
 CURVE ( )  GEOMETRIC_REPRESENTATION_ITEM ( )  RATIONAL_B_SPLINE_CURVE ( ( 1.000000000000003775, 0.9238795325112830747, 1.000000000000000000, 0.9238795325112867385, 1.000000000000000000, 0.9238795325112867385, 1.000000000000000000, 0.9238795325112817425, 1.000000000000005107 ) ) 
 REPRESENTATION_ITEM ( '' )  );
#11426=EDGE_LOOP ( 'NONE', ( #3320, #4204, #4394, #10545 ) ) ;
#11427=DIRECTION ( 'NONE',  ( -1.000000000000000000, -0.000000000000000000, -0.000000000000000000 ) ) ;
#11435=CARTESIAN_POINT ( 'NONE',  ( -66.85000000109248219, 9.999999999999998224, 12.93301269999999192 ) ) ;
#11436=CARTESIAN_POINT ( 'NONE',  ( 68.15000000109247935, 8.538419263543522320, 16.46158073645647235 ) ) ;
#11439=CARTESIAN_POINT ( 'NONE',  ( -67.15000000109247935, 11.46158073645647235, 13.53841926354352232 ) ) ;
#11461=LINE ( 'NONE', #18610, #21314 ) ;
#11463=CARTESIAN_POINT ( 'NONE',  ( -71.40000000218495302, 9.999999999999998224, 12.49999999999999289 ) ) ;
#11469=CARTESIAN_POINT ( 'NONE',  ( 69.09999999999999432, 12.50000000000000000, 14.99999999999999645 ) ) ;
#11473=CARTESIAN_POINT ( 'NONE',  ( -67.29999999999999716, 9.999999999999998224, 12.49999999999999289 ) ) ;
#11478=CARTESIAN_POINT ( 'NONE',  ( -70.45000000109247651, 12.06698730000000097, 14.99999999999999645 ) ) ;
#11485=CARTESIAN_POINT ( 'NONE',  ( -71.80000000109247082, 12.06698730000000275, 14.14382582708705094 ) ) ;
#11499=CARTESIAN_POINT ( 'NONE',  ( 70.15000000109247935, 11.46158073645647235, 13.53841926354352232 ) ) ;
#11503=CARTESIAN_POINT ( 'NONE',  ( 70.30000000109248504, 10.85617417291294551, 12.93301269999999370 ) ) ;
#11512=CARTESIAN_POINT ( 'NONE',  ( -67.30000000109247082, 12.06698729999999919, 15.85617417291294196 ) ) ;
#11525=DIRECTION ( 'NONE',  ( -1.000000000000000000, -0.000000000000000000, -0.000000000000000000 ) ) ;
#11532=CARTESIAN_POINT ( 'NONE',  ( 71.35000000109246798, 11.46158073645647235, 16.46158073645647235 ) ) ;
#11534=VECTOR ( 'NONE', #17678, 1000.000000000000000 ) ;
#11537=CARTESIAN_POINT ( 'NONE',  ( 67.60000000109248219, 9.143825827087050939, 12.93301269999999370 ) ) ;
#11543=LINE ( 'NONE', #18812, #14785 ) ;
#11545=FACE_OUTER_BOUND ( 'NONE', #8823, .T. ) ;
#11547=CARTESIAN_POINT ( 'NONE',  ( -66.90000000109247935, 10.85617417291294551, 12.93301269999999192 ) ) ;
#11550=CARTESIAN_POINT ( 'NONE',  ( -70.45000000109247651, 12.06698730000000097, 14.99999999999999645 ) ) ;
#11552=CARTESIAN_POINT ( 'NONE',  ( -69.29999999999999716, 9.999999999999998224, 17.49999999999999645 ) ) ;
#11558=CARTESIAN_POINT ( 'NONE',  ( -67.15000000109247935, 11.46158073645647235, 16.46158073645647235 ) ) ;
#11559=CARTESIAN_POINT ( 'NONE',  ( 67.70000000109247651, 10.85617417291294551, 12.93301269999999192 ) ) ;
#11560=CARTESIAN_POINT ( 'NONE',  ( -72.25000000000000000, 12.50000000000000000, 13.96446609406725869 ) ) ;
#11563=FACE_OUTER_BOUND ( 'NONE', #11359, .T. ) ;
#11567=EDGE_CURVE ( 'NONE', #6908, #7519, #945, .T. ) ;
#11578=ORIENTED_EDGE ( 'NONE', *, *, #17427, .T. ) ;
#11580=DIRECTION ( 'NONE',  ( -1.000000000000000000, -0.000000000000000000, -0.000000000000000000 ) ) ;
#11581=DIRECTION ( 'NONE',  ( 0.5000000000000013323, 0.000000000000000000, 0.8660254037844380415 ) ) ;
#11583=CARTESIAN_POINT ( 'NONE',  ( -69.30000000218494449, 11.76776695296636888, 16.76776695296636532 ) ) ;
#11597=CARTESIAN_POINT ( 'NONE',  ( -71.15000000109246514, 11.46158073645647235, 13.53841926354352232 ) ) ;
#11602=CARTESIAN_POINT ( 'NONE',  ( -71.90000000109247935, 12.06698730000000275, 15.85617417291294196 ) ) ;
#11610=CARTESIAN_POINT ( 'NONE',  ( 68.50000000109247367, 10.85617417291294551, 12.93301269999999370 ) ) ;
#11613=CARTESIAN_POINT ( 'NONE',  ( 71.05000000109245661, 9.999999999999998224, 12.93301269999999192 ) ) ;
#11619=DIRECTION ( 'NONE',  ( 0.000000000000000000, 0.000000000000000000, 1.000000000000000000 ) ) ;
#11621=CARTESIAN_POINT ( 'NONE',  ( -67.15000000109247935, 11.46158073645647235, 13.53841926354352232 ) ) ;
#11622=VERTEX_POINT ( 'NONE', #5137 ) ;
#11631=LINE ( 'NONE', #13182, #16639 ) ;
#11635=CARTESIAN_POINT ( 'NONE',  ( -70.70000000218495018, 11.76776695296636888, 13.23223304703362579 ) ) ;
#11639=CARTESIAN_POINT ( 'NONE',  ( 71.10000000109246798, 12.06698729999999919, 15.85617417291294196 ) ) ;
#11646=CARTESIAN_POINT ( 'NONE',  ( 69.20000000109246230, 7.933012699999995476, 15.85617417291294196 ) ) ;
#11650=CARTESIAN_POINT ( 'NONE',  ( 68.55000000109247082, 8.538419263543524096, 13.53841926354352054 ) ) ;
#11662=CARTESIAN_POINT ( 'NONE',  ( -66.50000000109247367, 9.143825827087049163, 17.06698730000000097 ) ) ;
#11665=CARTESIAN_POINT ( 'NONE',  ( -66.85000000109246798, 7.933012699999995476, 14.99999999999999645 ) ) ;
#11672=CARTESIAN_POINT ( 'NONE',  ( -66.10000000109248219, 10.85617417291294551, 12.93301269999999370 ) ) ;
#11673=CARTESIAN_POINT ( 'NONE',  ( 68.65000000109247935, 12.06698730000000097, 14.99999999999999645 ) ) ;
#11675=CARTESIAN_POINT ( 'NONE',  ( -72.14999999999999147, 11.03553390593273598, 12.49999999999999289 ) ) ;
#11682=FACE_OUTER_BOUND ( 'NONE', #2831, .T. ) ;
#11685=ORIENTED_EDGE ( 'NONE', *, *, #8978, .F. ) ;
#11697=CARTESIAN_POINT ( 'NONE',  ( -70.30000000218494449, 8.232233047033627571, 16.76776695296636532 ) ) ;
#11703=CARTESIAN_POINT ( 'NONE',  ( 68.30000000109247082, 7.933012699999995476, 14.14382582708705094 ) ) ;
#11710=CARTESIAN_POINT ( 'NONE',  ( 68.95000000218495018, 8.964466094067285340, 12.49999999999996980 ) ) ;
#11717=CARTESIAN_POINT ( 'NONE',  ( -71.20000000109246230, 10.85617417291294551, 17.06698729999999742 ) ) ;
#11719=ORIENTED_EDGE ( 'NONE', *, *, #17427, .F. ) ;
#11722=ORIENTED_EDGE ( 'NONE', *, *, #19125, .T. ) ;
#11729=CARTESIAN_POINT ( 'NONE',  ( 67.45000000109246230, 7.933012699999995476, 14.99999999999999645 ) ) ;
#11730=CARTESIAN_POINT ( 'NONE',  ( 67.25000000109245946, 12.06698730000000097, 14.99999999999999645 ) ) ;
#11732=ORIENTED_EDGE ( 'NONE', *, *, #11567, .T. ) ;
#11736=CARTESIAN_POINT ( 'NONE',  ( 71.65000000218496723, 12.50000000000000000, 16.03553390593273775 ) ) ;
#11744=VERTEX_POINT ( 'NONE', #10909 ) ;
#11745=CARTESIAN_POINT ( 'NONE',  ( 69.35000000218497007, 11.03553390593273420, 17.50000000000000711 ) ) ;
#11747=DIRECTION ( 'NONE',  ( -1.000000000000000000, -0.000000000000000000, -0.000000000000000000 ) ) ;
#11753=CARTESIAN_POINT ( 'NONE',  ( 70.80000000109245661, 9.143825827087052716, 12.93301269999999192 ) ) ;
#11759=CARTESIAN_POINT ( 'NONE',  ( 69.85000000109246798, 9.999999999999998224, 17.06698730000000097 ) ) ;
#11765=CARTESIAN_POINT ( 'NONE',  ( 71.20000000109246230, 12.06698730000000275, 14.14382582708705094 ) ) ;
#11773=CARTESIAN_POINT ( 'NONE',  ( 71.40000000218495302, 9.999999999999998224, 12.49999999999999289 ) ) ;
#11778=CARTESIAN_POINT ( 'NONE',  ( -68.70000000109246230, 10.85617417291294551, 12.93301269999999370 ) ) ;
#11788=CARTESIAN_POINT ( 'NONE',  ( -66.20000000109247651, 12.06698730000000275, 14.14382582708705094 ) ) ;
#11789=CARTESIAN_POINT ( 'NONE',  ( 67.75000000109247367, 11.46158073645647235, 13.53841926354352232 ) ) ;
#11792=CARTESIAN_POINT ( 'NONE',  ( -67.25000000109245946, 12.06698730000000097, 14.99999999999999645 ) ) ;
#11815=CARTESIAN_POINT ( 'NONE',  ( -69.55000000218495870, 7.499999999999995559, 16.03553390593273420 ) ) ;
#11821=CARTESIAN_POINT ( 'NONE',  ( 70.95000000109247651, 11.46158073645647235, 13.53841926354352232 ) ) ;
#11822=CARTESIAN_POINT ( 'NONE',  ( 70.95000000218495018, 11.03553390593269867, 17.50000000000003908 ) ) ;
#11827=CARTESIAN_POINT ( 'NONE',  ( 67.64999999999999147, 11.03553390593272887, 17.50000000000001066 ) ) ;
#11828=CARTESIAN_POINT ( 'NONE',  ( -68.60000000109246798, 9.143825827087052716, 12.93301269999999192 ) ) ;
#11843=CARTESIAN_POINT ( 'NONE',  ( 67.95000000109247651, 11.46158073645647235, 16.46158073645647235 ) ) ;
#11845=CARTESIAN_POINT ( 'NONE',  ( 68.40000000109246514, 7.933012699999995476, 15.85617417291294196 ) ) ;
#11848=PRODUCT_DEFINITION_FORMATION_WITH_SPECIFIED_SOURCE ( 'ANY', '', #127, .NOT_KNOWN. ) ;
#11854=CYLINDRICAL_SURFACE ( 'NONE', #4785, 2.500000000000002220 ) ;
#11877=CARTESIAN_POINT ( 'NONE',  ( 69.60000000218495586, 7.499999999999996447, 14.99999999999999645 ) ) ;
#11880=CARTESIAN_POINT ( 'NONE',  ( 66.40000000109247935, 12.06698729999999919, 14.14382582708705094 ) ) ;
#11885=CARTESIAN_POINT ( 'NONE',  ( 69.20000000109246230, 7.933012699999995476, 15.85617417291294196 ) ) ;
#11893=EDGE_CURVE ( 'NONE', #16036, #21124, #94, .T. ) ;
#11898=CARTESIAN_POINT ( 'NONE',  ( -66.25000000109247367, 12.06698730000000097, 14.99999999999999645 ) ) ;
#11900=CARTESIAN_POINT ( 'NONE',  ( -66.95000000109246230, 8.538419263543524096, 13.53841926354352054 ) ) ;
#11914=CARTESIAN_POINT ( 'NONE',  ( -67.85000000109246798, 9.999999999999998224, 12.93301269999999192 ) ) ;
#11915=( BOUNDED_CURVE ( )  B_SPLINE_CURVE ( 2, ( #8741, #6700, #4547, #8622, #14015, #13666, #10201, #4662, #21274 ),
 .UNSPECIFIED., .F., .F. ) 
 B_SPLINE_CURVE_WITH_KNOTS ( ( 3, 2, 2, 2, 3 ),
 ( 0.4374999999999995004, 0.4531249999999993894, 0.4687499999999993339, 0.4843749999999992228, 0.4999999999999991118 ),
 .UNSPECIFIED. ) 
 CURVE ( )  GEOMETRIC_REPRESENTATION_ITEM ( )  RATIONAL_B_SPLINE_CURVE ( ( 1.000000000000002442, 0.9238795325112842960, 1.000000000000000000, 0.9238795325112867385, 1.000000000000000000, 0.9238795325112867385, 1.000000000000000000, 0.9238795325112910684, 0.9999999999999956701 ) ) 
 REPRESENTATION_ITEM ( '' )  );
#11938=CARTESIAN_POINT ( 'NONE',  ( 72.50000000000000000, 9.999999999999998224, 12.49999999999999289 ) ) ;
#11941=CARTESIAN_POINT ( 'NONE',  ( -69.65000000218496723, 7.499999999999995559, 13.96446609406725692 ) ) ;
#11944=CARTESIAN_POINT ( 'NONE',  ( 66.69999999999998863, 12.50000000000000000, 14.99999999999999645 ) ) ;
#11947=CARTESIAN_POINT ( 'NONE',  ( 69.30000000109247082, 10.85617417291294551, 12.93301269999999370 ) ) ;
#11952=CARTESIAN_POINT ( 'NONE',  ( -70.10000000109246798, 7.933012699999995476, 14.14382582708705094 ) ) ;
#11966=CARTESIAN_POINT ( 'NONE',  ( 68.60000000109248219, 12.06698730000000275, 14.14382582708705094 ) ) ;
#11968=CARTESIAN_POINT ( 'NONE',  ( 66.95000000109246230, 8.538419263543524096, 13.53841926354352054 ) ) ;
#11972=CARTESIAN_POINT ( 'NONE',  ( 71.45000000218495018, 11.03553390593275374, 12.50000000000001243 ) ) ;
#11973=CARTESIAN_POINT ( 'NONE',  ( 72.50000000000000000, 9.999999999999998224, 14.99999999999999645 ) ) ;
#11984=CARTESIAN_POINT ( 'NONE',  ( 71.40000000218495302, 9.999999999999998224, 12.49999999999999289 ) ) ;
#11987=VERTEX_POINT ( 'NONE', #17471 ) ;
#11989=CARTESIAN_POINT ( 'NONE',  ( 71.35000000218494165, 8.964466094067258695, 12.49999999999999289 ) ) ;
#11994=CARTESIAN_POINT ( 'NONE',  ( 66.10000000109246798, 7.933012699999995476, 14.14382582708705094 ) ) ;
#11999=CARTESIAN_POINT ( 'NONE',  ( 71.25000000109247367, 12.06698730000000097, 14.99999999999999645 ) ) ;
#12011=ORIENTED_EDGE ( 'NONE', *, *, #22673, .T. ) ;
#12012=CARTESIAN_POINT ( 'NONE',  ( -66.35000000109246798, 11.46158073645647235, 13.53841926354352232 ) ) ;
#12021=CARTESIAN_POINT ( 'NONE',  ( -67.00000000218494733, 9.999999999999998224, 17.49999999999999645 ) ) ;
#12023=ADVANCED_FACE ( 'NONE', ( #13419 ), #20685, .T. ) ;
#12025=CARTESIAN_POINT ( 'NONE',  ( -71.74999999999998579, 8.964466094067258695, 17.50000000000000355 ) ) ;
#12033=CARTESIAN_POINT ( 'NONE',  ( 71.70000000000000284, 9.999999999999998224, 17.49999999999999645 ) ) ;
#12035=CARTESIAN_POINT ( 'NONE',  ( -68.09999999999999432, 9.999999999999998224, 12.49999999999999289 ) ) ;
#12048=CARTESIAN_POINT ( 'NONE',  ( -67.40000000218495302, 9.999999999999998224, 12.49999999999999289 ) ) ;
#12056=CARTESIAN_POINT ( 'NONE',  ( 70.50000000109247367, 9.143825827087049163, 17.06698729999999742 ) ) ;
#12058=CARTESIAN_POINT ( 'NONE',  ( 70.65000000218495302, 11.03553390593268269, 12.49999999999994138 ) ) ;
#12063=CARTESIAN_POINT ( 'NONE',  ( -67.90000000109246514, 10.85617417291294551, 12.93301269999999192 ) ) ;
#12066=CARTESIAN_POINT ( 'NONE',  ( 65.70000000218495018, 8.232233047033629347, 13.23223304703362402 ) ) ;
#12078=CARTESIAN_POINT ( 'NONE',  ( 69.25000000109247367, 9.999999999999998224, 12.93301269999999192 ) ) ;
#12080=CARTESIAN_POINT ( 'NONE',  ( 66.85000000109246798, 7.933012699999995476, 14.99999999999999645 ) ) ;
#12084=( BOUNDED_CURVE ( )  B_SPLINE_CURVE ( 2, ( #7594, #14916, #13117, #20019, #1821, #11320, #5544, #2177, #9514 ),
 .UNSPECIFIED., .F., .F. ) 
 B_SPLINE_CURVE_WITH_KNOTS ( ( 3, 2, 2, 2, 3 ),
 ( 0.06249999999999961836, 0.07812499999999952816, 0.09374999999999943101, 0.1093749999999993339, 0.1249999999999992367 ),
 .UNSPECIFIED. ) 
 CURVE ( )  GEOMETRIC_REPRESENTATION_ITEM ( )  RATIONAL_B_SPLINE_CURVE ( ( 1.000000000000001776, 0.9238795325112848511, 1.000000000000000000, 0.9238795325112867385, 1.000000000000000000, 0.9238795325112867385, 1.000000000000000000, 0.9238795325112904022, 0.9999999999999963363 ) ) 
 REPRESENTATION_ITEM ( '' )  );
#12089=CARTESIAN_POINT ( 'NONE',  ( 68.00000000218494733, 7.499999999999996447, 14.99999999999999645 ) ) ;
#12091=EDGE_LOOP ( 'NONE', ( #14057, #13546, #16856, #8887 ) ) ;
#12102=CARTESIAN_POINT ( 'NONE',  ( -69.49999999999998579, 7.499999999999996447, 14.99999999999999645 ) ) ;
#12105=FACE_OUTER_BOUND ( 'NONE', #516, .T. ) ;
#12110=CARTESIAN_POINT ( 'NONE',  ( 67.30000000109247082, 12.06698729999999919, 15.85617417291294196 ) ) ;
#12114=CARTESIAN_POINT ( 'NONE',  ( 70.05000000109247082, 7.933012699999995476, 14.99999999999999645 ) ) ;
#12127=CARTESIAN_POINT ( 'NONE',  ( -67.60000000109246798, 7.933012699999995476, 15.85617417291294196 ) ) ;
#12135=CARTESIAN_POINT ( 'NONE',  ( -66.60000000218495586, 9.999999999999998224, 12.49999999999999289 ) ) ;
#12136=CARTESIAN_POINT ( 'NONE',  ( 66.60000000109248219, 7.933012699999995476, 15.85617417291294196 ) ) ;
#12137=CARTESIAN_POINT ( 'NONE',  ( -69.45000000000000284, 7.499999999999995559, 16.03553390593273420 ) ) ;
#12148=CARTESIAN_POINT ( 'NONE',  ( -70.80000000109245661, 9.143825827087052716, 12.93301269999999192 ) ) ;
#12151=CARTESIAN_POINT ( 'NONE',  ( -69.20000000109246230, 9.143825827087050939, 12.93301269999999370 ) ) ;
#12161=CARTESIAN_POINT ( 'NONE',  ( -67.75000000218496155, 11.03553390593273598, 17.50000000000000355 ) ) ;
#12164=CARTESIAN_POINT ( 'NONE',  ( -71.65000000109246514, 7.933012699999995476, 14.99999999999999645 ) ) ;
#12175=CARTESIAN_POINT ( 'NONE',  ( 67.50000000218494733, 11.76776695296636888, 13.23223304703362579 ) ) ;
#12176=CARTESIAN_POINT ( 'NONE',  ( 67.39999999999999147, 11.76776695296636888, 13.23223304703362579 ) ) ;
#12177=CARTESIAN_POINT ( 'NONE',  ( -69.65000000109246514, 12.06698730000000097, 14.99999999999999645 ) ) ;
#12181=ORIENTED_EDGE ( 'NONE', *, *, #21624, .T. ) ;
#12187=ORIENTED_EDGE ( 'NONE', *, *, #1635, .F. ) ;
#12193=ADVANCED_FACE ( 'NONE', ( #21620 ), #8495, .T. ) ;
#12198=CARTESIAN_POINT ( 'NONE',  ( 66.25000000109247367, 12.06698730000000097, 14.99999999999999645 ) ) ;
#12200=CARTESIAN_POINT ( 'NONE',  ( 67.55000000109247082, 8.538419263543522320, 16.46158073645647235 ) ) ;
#12217=AXIS2_PLACEMENT_3D ( 'NONE', #5428, #3514, #7121 ) ;
#12221=CARTESIAN_POINT ( 'NONE',  ( 65.90000000218495302, 11.76776695296636888, 13.23223304703362579 ) ) ;
#12226=CARTESIAN_POINT ( 'NONE',  ( 70.20000000218495018, 9.999999999999998224, 17.49999999999999645 ) ) ;
#12227=( BOUNDED_CURVE ( )  B_SPLINE_CURVE ( 2, ( #3070, #10645, #7031, #6787, #1373, #15791, #17919, #23423, #14464 ),
 .UNSPECIFIED., .F., .F. ) 
 B_SPLINE_CURVE_WITH_KNOTS ( ( 3, 2, 2, 2, 3 ),
 ( 0.9375000000000007772, 0.9531250000000005551, 0.9687500000000004441, 0.9843750000000002220, 1.000000000000000000 ),
 .UNSPECIFIED. ) 
 CURVE ( )  GEOMETRIC_REPRESENTATION_ITEM ( )  RATIONAL_B_SPLINE_CURVE ( ( 0.9999999999999962252, 0.9238795325112905132, 1.000000000000000000, 0.9238795325112867385, 1.000000000000000000, 0.9238795325112867385, 1.000000000000000000, 0.9238795325112867385, 1.000000000000000000 ) ) 
 REPRESENTATION_ITEM ( '' )  );
#12228=CARTESIAN_POINT ( 'NONE',  ( 71.80000000218494449, 9.999999999999998224, 17.49999999999999645 ) ) ;
#12229=VECTOR ( 'NONE', #16892, 1000.000000000000000 ) ;
#12231=CARTESIAN_POINT ( 'NONE',  ( 66.30000000109247082, 10.85617417291294551, 12.93301269999999192 ) ) ;
#12237=CARTESIAN_POINT ( 'NONE',  ( 66.95000000109246230, 8.538419263543524096, 13.53841926354352054 ) ) ;
#12242=ORIENTED_EDGE ( 'NONE', *, *, #8635, .T. ) ;
#12256=AXIS2_PLACEMENT_3D ( 'NONE', #3563, #16042, #8735 ) ;
#12260=CARTESIAN_POINT ( 'NONE',  ( 66.40000000109247935, 10.85617417291294551, 17.06698730000000097 ) ) ;
#12263=CARTESIAN_POINT ( 'NONE',  ( -70.39999999999999147, 8.232233047033629347, 13.23223304703362402 ) ) ;
#12277=CARTESIAN_POINT ( 'NONE',  ( -66.25000000109247367, 12.06698730000000097, 14.99999999999999645 ) ) ;
#12288=CARTESIAN_POINT ( 'NONE',  ( -66.50000000218494733, 8.232233047033629347, 13.23223304703362402 ) ) ;
#12313=CARTESIAN_POINT ( 'NONE',  ( 68.60000000218495586, 9.999999999999998224, 17.49999999999999645 ) ) ;
#12320=CARTESIAN_POINT ( 'NONE',  ( 71.74999999999998579, 8.964466094067258695, 17.50000000000000355 ) ) ;
#12332=DIRECTION ( 'NONE',  ( -1.000000000000000000, -0.000000000000000000, -0.000000000000000000 ) ) ;
#12338=CARTESIAN_POINT ( 'NONE',  ( 71.35000000109246798, 8.538419263543522320, 16.46158073645647235 ) ) ;
#12340=ORIENTED_EDGE ( 'NONE', *, *, #18553, .T. ) ;
#12344=CARTESIAN_POINT ( 'NONE',  ( 69.25000000218494733, 12.50000000000000000, 16.03553390593273420 ) ) ;
#12346=CARTESIAN_POINT ( 'NONE',  ( -68.49999999999998579, 9.999999999999998224, 17.49999999999999645 ) ) ;
#12353=CARTESIAN_POINT ( 'NONE',  ( 67.50000000109245946, 9.143825827087049163, 17.06698729999999742 ) ) ;
#12374=CARTESIAN_POINT ( 'NONE',  ( -65.75000000109247367, 8.538419263543522320, 16.46158073645647235 ) ) ;
#12377=CARTESIAN_POINT ( 'NONE',  ( -69.79999999999999716, 11.76776695296636888, 13.23223304703362579 ) ) ;
#12390=CARTESIAN_POINT ( 'NONE',  ( -68.35000000109248219, 8.538419263543524096, 13.53841926354352054 ) ) ;
#12401=CARTESIAN_POINT ( 'NONE',  ( -68.15000000218495302, 8.964466094067258695, 12.49999999999999289 ) ) ;
#12411=CARTESIAN_POINT ( 'NONE',  ( 70.35000000218495586, 7.499999999999996447, 16.03553390593273775 ) ) ;
#12416=DIRECTION ( 'NONE',  ( 0.000000000000000000, 0.000000000000000000, -1.000000000000000000 ) ) ;
#12432=CARTESIAN_POINT ( 'NONE',  ( 66.35000000109248219, 11.46158073645647235, 16.46158073645647235 ) ) ;
#12433=CARTESIAN_POINT ( 'NONE',  ( 71.20000000000000284, 8.232233047033629347, 13.23223304703362402 ) ) ;
#12435=CARTESIAN_POINT ( 'NONE',  ( 69.45000000000000284, 7.499999999999996447, 16.03553390593273775 ) ) ;
#12453=VERTEX_POINT ( 'NONE', #19108 ) ;
#12460=ADVANCED_FACE ( 'NONE', ( #7754 ), #18757, .T. ) ;
#12461=CARTESIAN_POINT ( 'NONE',  ( 67.45000000218493597, 11.03553390593273598, 12.49999999999999289 ) ) ;
#12471=CARTESIAN_POINT ( 'NONE',  ( 67.15000000109247935, 11.46158073645647235, 13.53841926354352232 ) ) ;
#12474=AXIS2_PLACEMENT_3D ( 'NONE', #1691, #14302, #19778 ) ;
#12495=EDGE_CURVE ( 'NONE', #6076, #18376, #23285, .T. ) ;
#12503=CARTESIAN_POINT ( 'NONE',  ( -71.20000000000000284, 8.232233047033629347, 13.23223304703362402 ) ) ;
#12511=ORIENTED_EDGE ( 'NONE', *, *, #10837, .F. ) ;
#12512=CARTESIAN_POINT ( 'NONE',  ( -71.90000000109247935, 12.06698729999999919, 15.85617417291294196 ) ) ;
#12515=CARTESIAN_POINT ( 'NONE',  ( -68.85000000109248219, 9.999999999999998224, 17.06698730000000097 ) ) ;
#12525=ADVANCED_FACE ( 'NONE', ( #3407 ), #13864, .T. ) ;
#12526=CARTESIAN_POINT ( 'NONE',  ( -68.70000000218495018, 8.232233047033627571, 16.76776695296636532 ) ) ;
#12528=CARTESIAN_POINT ( 'NONE',  ( -72.10000000109246798, 12.06698730000000275, 15.85617417291294196 ) ) ;
#12559=CARTESIAN_POINT ( 'NONE',  ( 72.50000000000000000, 9.999999999999998224, 17.49999999999999645 ) ) ;
#12562=CARTESIAN_POINT ( 'NONE',  ( 69.70000000000000284, 9.999999999999998224, 12.49999999999999289 ) ) ;
#12571=DIRECTION ( 'NONE',  ( 0.000000000000000000, 0.000000000000000000, 1.000000000000000000 ) ) ;
#12583=CARTESIAN_POINT ( 'NONE',  ( 67.20000000218495018, 7.499999999999996447, 14.99999999999999645 ) ) ;
#12597=CARTESIAN_POINT ( 'NONE',  ( 66.30000000109247082, 10.85617417291294551, 12.93301269999999370 ) ) ;
#12622=CARTESIAN_POINT ( 'NONE',  ( -66.59999999999999432, 11.76776695296636888, 13.23223304703362579 ) ) ;
#12630=CARTESIAN_POINT ( 'NONE',  ( -66.10000000109246798, 7.933012699999995476, 14.14382582708705094 ) ) ;
#12631=CARTESIAN_POINT ( 'NONE',  ( 68.50000000218494733, 11.76776695296636888, 16.76776695296636532 ) ) ;
#12634=EDGE_CURVE ( 'NONE', #8256, #5464, #23112, .T. ) ;
#12639=CARTESIAN_POINT ( 'NONE',  ( -68.45000000109247651, 9.999999999999998224, 12.93301269999999192 ) ) ;
#12641=AXIS2_PLACEMENT_3D ( 'NONE', #9714, #6106, #7686 ) ;
#12648=CARTESIAN_POINT ( 'NONE',  ( -72.05000000109247082, 9.999999999999998224, 17.06698730000000097 ) ) ;
#12649=CARTESIAN_POINT ( 'NONE',  ( -68.80000000109247082, 12.06698730000000275, 14.14382582708705094 ) ) ;
#12681=CARTESIAN_POINT ( 'NONE',  ( 66.45000000109247651, 9.999999999999998224, 17.06698730000000097 ) ) ;
#12684=CARTESIAN_POINT ( 'NONE',  ( 70.39999999999999147, 8.232233047033629347, 13.23223304703362402 ) ) ;
#12686=CARTESIAN_POINT ( 'NONE',  ( 69.50000000218494733, 8.232233047033627571, 16.76776695296636532 ) ) ;
#12694=ORIENTED_EDGE ( 'NONE', *, *, #19940, .T. ) ;
#12708=CARTESIAN_POINT ( 'NONE',  ( 66.60000000218495586, 9.999999999999998224, 12.49999999999999289 ) ) ;
#12709=CYLINDRICAL_SURFACE ( 'NONE', #12256, 2.500000000000002220 ) ;
#12717=CARTESIAN_POINT ( 'NONE',  ( 66.10000000109246798, 7.933012699999995476, 14.14382582708705094 ) ) ;
#12718=CARTESIAN_POINT ( 'NONE',  ( -67.79999999999999716, 8.232233047033627571, 16.76776695296636532 ) ) ;
#12724=CARTESIAN_POINT ( 'NONE',  ( -72.20000000000000284, 11.76776695296636888, 13.23223304703362579 ) ) ;
#12735=CARTESIAN_POINT ( 'NONE',  ( -66.19999999999998863, 8.232233047033627571, 16.76776695296636532 ) ) ;
#12740=CARTESIAN_POINT ( 'NONE',  ( -66.09999999999999432, 9.999999999999998224, 17.49999999999999645 ) ) ;
#12749=CARTESIAN_POINT ( 'NONE',  ( -69.25000000109247367, 9.999999999999998224, 12.93301269999999192 ) ) ;
#12752=CARTESIAN_POINT ( 'NONE',  ( -67.75000000109247367, 11.46158073645647235, 13.53841926354352232 ) ) ;
#12754=LINE ( 'NONE', #10947, #10585 ) ;
#12760=CARTESIAN_POINT ( 'NONE',  ( -69.60000000109249640, 10.85617417291294551, 17.06698729999999742 ) ) ;
#12762=EDGE_CURVE ( 'NONE', #6076, #4468, #10795, .T. ) ;
#12763=CARTESIAN_POINT ( 'NONE',  ( -69.75000000109245946, 11.46158073645647235, 16.46158073645647235 ) ) ;
#12780=ORIENTED_EDGE ( 'NONE', *, *, #21355, .F. ) ;
#12791=CARTESIAN_POINT ( 'NONE',  ( 72.29999999999998295, 12.50000000000000000, 14.99999999999999645 ) ) ;
#12794=CARTESIAN_POINT ( 'NONE',  ( 69.54999999999999716, 7.499999999999996447, 13.96446609406725514 ) ) ;
#12813=CARTESIAN_POINT ( 'NONE',  ( 68.50000000218494733, 11.76776695296636888, 16.76776695296636532 ) ) ;
#12815=( BOUNDED_CURVE ( )  B_SPLINE_CURVE ( 2, ( #6536, #11822, #17986, #13611, #1119, #13964, #776, #12058, #8463 ),
 .UNSPECIFIED., .F., .F. ) 
 B_SPLINE_CURVE_WITH_KNOTS ( ( 3, 2, 2, 2, 3 ),
 ( 0.1249999999999992367, 0.1406249999999996947, 0.1562500000000001388, 0.1718750000000005829, 0.1875000000000010270 ),
 .UNSPECIFIED. ) 
 CURVE ( )  GEOMETRIC_REPRESENTATION_ITEM ( )  RATIONAL_B_SPLINE_CURVE ( ( 1.000000000000003775, 0.9238795325112830747, 1.000000000000000000, 0.9238795325112867385, 1.000000000000000000, 0.9238795325112867385, 1.000000000000000000, 0.9238795325112817425, 1.000000000000005107 ) ) 
 REPRESENTATION_ITEM ( '' )  );
#12845=CARTESIAN_POINT ( 'NONE',  ( -68.09999999999999432, 9.999999999999998224, 12.49999999999999289 ) ) ;
#12848=CARTESIAN_POINT ( 'NONE',  ( 71.95000000109247651, 11.46158073645647235, 13.53841926354352232 ) ) ;
#12858=CARTESIAN_POINT ( 'NONE',  ( -68.50000000109247367, 10.85617417291294551, 12.93301269999999192 ) ) ;
#12861=CARTESIAN_POINT ( 'NONE',  ( -70.00000000109247367, 7.933012699999995476, 15.85617417291294196 ) ) ;
#12871=CARTESIAN_POINT ( 'NONE',  ( -71.65000000109247935, 9.999999999999998224, 12.93301269999999192 ) ) ;
#12872=CARTESIAN_POINT ( 'NONE',  ( -70.75000000109247367, 8.538419263543522320, 16.46158073645647235 ) ) ;
#12884=CARTESIAN_POINT ( 'NONE',  ( -70.50000000000000000, 9.999999999999998224, 12.49999999999999289 ) ) ;
#12898=CARTESIAN_POINT ( 'NONE',  ( 67.54999999999999716, 12.50000000000000000, 16.03553390593273420 ) ) ;
#12925=CARTESIAN_POINT ( 'NONE',  ( 70.95000000109247651, 11.46158073645647235, 13.53841926354352232 ) ) ;
#12927=CARTESIAN_POINT ( 'NONE',  ( 72.10000000109246798, 12.06698730000000275, 15.85617417291294196 ) ) ;
#12931=VECTOR ( 'NONE', #5870, 1000.000000000000000 ) ;
#12941=FACE_OUTER_BOUND ( 'NONE', #15803, .T. ) ;
#12944=SURFACE_STYLE_USAGE ( .BOTH. , #2125 ) ;
#12956=( BOUNDED_CURVE ( )  B_SPLINE_CURVE ( 2, ( #15130, #5641, #22391, #11182, #18456, #9375, #16665, #14893, #20474 ),
 .UNSPECIFIED., .F., .F. ) 
 B_SPLINE_CURVE_WITH_KNOTS ( ( 3, 2, 2, 2, 3 ),
 ( 0.6875000000000001110, 0.7031250000000000000, 0.7187500000000000000, 0.7343749999999998890, 0.7499999999999997780 ),
 .UNSPECIFIED. ) 
 CURVE ( )  GEOMETRIC_REPRESENTATION_ITEM ( )  RATIONAL_B_SPLINE_CURVE ( ( 0.9999999999999994449, 0.9238795325112872936, 1.000000000000000000, 0.9238795325112867385, 1.000000000000000000, 0.9238795325112867385, 1.000000000000000000, 0.9238795325112878487, 0.9999999999999988898 ) ) 
 REPRESENTATION_ITEM ( '' )  );
#12966=CARTESIAN_POINT ( 'NONE',  ( -67.20000000000000284, 8.232233047033629347, 13.23223304703362402 ) ) ;
#12968=CARTESIAN_POINT ( 'NONE',  ( 67.90000000109246514, 12.06698730000000275, 15.85617417291294196 ) ) ;
#12978=CARTESIAN_POINT ( 'NONE',  ( -70.10000000109248219, 10.85617417291294551, 12.93301269999999192 ) ) ;
#12981=CARTESIAN_POINT ( 'NONE',  ( -69.80000000109247082, 10.85617417291294551, 17.06698729999999742 ) ) ;
#12991=CARTESIAN_POINT ( 'NONE',  ( -71.95000000109247651, 11.46158073645647235, 16.46158073645647235 ) ) ;
#12992=CARTESIAN_POINT ( 'NONE',  ( -70.10000000109245377, 7.933012699999995476, 14.14382582708705094 ) ) ;
#13000=CARTESIAN_POINT ( 'NONE',  ( 68.84999999999998010, 8.964466094067214286, 12.50000000000004086 ) ) ;
#13003=CARTESIAN_POINT ( 'NONE',  ( 70.25000000000000000, 7.499999999999996447, 16.03553390593273775 ) ) ;
#13004=CARTESIAN_POINT ( 'NONE',  ( -71.65000000218496723, 12.50000000000000000, 16.03553390593273775 ) ) ;
#13005=ORIENTED_EDGE ( 'NONE', *, *, #13379, .T. ) ;
#13010=ORIENTED_EDGE ( 'NONE', *, *, #21331, .F. ) ;
#13024=CARTESIAN_POINT ( 'NONE',  ( 67.39999999999999147, 11.76776695296636888, 13.23223304703362579 ) ) ;
#13032=CARTESIAN_POINT ( 'NONE',  ( -71.50000000109247367, 9.143825827087049163, 17.06698730000000097 ) ) ;
#13049=STYLED_ITEM ( 'NONE', ( #13180 ), #19874 ) ;
#13051=CARTESIAN_POINT ( 'NONE',  ( 71.05000000109247082, 12.06698730000000097, 14.99999999999999645 ) ) ;
#13052=CARTESIAN_POINT ( 'NONE',  ( 66.44999999999998863, 8.964466094067219615, 12.50000000000003553 ) ) ;
#13053=CARTESIAN_POINT ( 'NONE',  ( 70.55000000109245661, 11.46158073645647235, 16.46158073645647235 ) ) ;
#13061=CARTESIAN_POINT ( 'NONE',  ( 70.20000000218495018, 9.999999999999998224, 17.49999999999999645 ) ) ;
#13063=CARTESIAN_POINT ( 'NONE',  ( -65.95000000109246230, 8.538419263543522320, 16.46158073645647235 ) ) ;
#13068=CYLINDRICAL_SURFACE ( 'NONE', #5443, 2.500000000000002220 ) ;
#13084=SURFACE_STYLE_FILL_AREA ( #22257 ) ;
#13085=CARTESIAN_POINT ( 'NONE',  ( 69.60000000109246798, 12.06698729999999919, 14.14382582708705094 ) ) ;
#13090=CARTESIAN_POINT ( 'NONE',  ( 65.90000000109246514, 7.933012699999995476, 14.14382582708705094 ) ) ;
#13099=CARTESIAN_POINT ( 'NONE',  ( -68.55000000109247082, 11.46158073645647235, 13.53841926354352232 ) ) ;
#13102=CARTESIAN_POINT ( 'NONE',  ( -69.45000000109247651, 9.999999999999998224, 12.93301269999999192 ) ) ;
#13105=ORIENTED_EDGE ( 'NONE', *, *, #4392, .T. ) ;
#13110=CARTESIAN_POINT ( 'NONE',  ( -70.20000000109246230, 12.06698730000000275, 14.14382582708705094 ) ) ;
#13111=CARTESIAN_POINT ( 'NONE',  ( 70.10000000109248219, 10.85617417291294551, 12.93301269999999192 ) ) ;
#13113=CARTESIAN_POINT ( 'NONE',  ( -69.60000000109248219, 12.06698730000000275, 14.14382582708705094 ) ) ;
#13117=CARTESIAN_POINT ( 'NONE',  ( 72.00000000000000000, 8.232233047033629347, 13.23223304703362402 ) ) ;
#13123=CARTESIAN_POINT ( 'NONE',  ( 70.09999999999999432, 9.999999999999998224, 17.49999999999999645 ) ) ;
#13124=CARTESIAN_POINT ( 'NONE',  ( -70.25000000000000000, 7.499999999999996447, 16.03553390593273775 ) ) ;
#13137=CARTESIAN_POINT ( 'NONE',  ( 69.59999999999999432, 8.232233047033629347, 13.23223304703362402 ) ) ;
#13143=CARTESIAN_POINT ( 'NONE',  ( -71.95000000000001705, 7.499999999999996447, 13.96446609406725514 ) ) ;
#13144=CARTESIAN_POINT ( 'NONE',  ( -72.10000000109246798, 12.06698729999999919, 15.85617417291294196 ) ) ;
#13161=CARTESIAN_POINT ( 'NONE',  ( 65.90000000218495302, 11.76776695296636888, 13.23223304703362579 ) ) ;
#13172=ADVANCED_FACE ( 'NONE', ( #12105 ), #8973, .T. ) ;
#13173=CARTESIAN_POINT ( 'NONE',  ( -66.90000000109247935, 7.933012699999995476, 14.14382582708705094 ) ) ;
#13175=VERTEX_POINT ( 'NONE', #19819 ) ;
#13180=PRESENTATION_STYLE_ASSIGNMENT (( #12944 ) ) ;
#13182=CARTESIAN_POINT ( 'NONE',  ( -65.97500000054623115, 9.999999999999998224, 17.28349365000000049 ) ) ;
#13183=CARTESIAN_POINT ( 'NONE',  ( 70.84999999999998010, 11.03553390593276973, 17.49999999999997158 ) ) ;
#13195=CARTESIAN_POINT ( 'NONE',  ( 71.40000000109246514, 10.85617417291294551, 17.06698730000000097 ) ) ;
#13200=CARTESIAN_POINT ( 'NONE',  ( 66.20000000218495018, 9.999999999999998224, 17.49999999999999645 ) ) ;
#13201=CARTESIAN_POINT ( 'NONE',  ( 66.55000000109247082, 8.538419263543522320, 16.46158073645647235 ) ) ;
#13211=CARTESIAN_POINT ( 'NONE',  ( -69.80000000109247082, 7.933012699999995476, 15.85617417291294196 ) ) ;
#13214=CARTESIAN_POINT ( 'NONE',  ( -71.00000000109245946, 9.143825827087050939, 12.93301269999999370 ) ) ;
#13226=CARTESIAN_POINT ( 'NONE',  ( -68.15000000109247935, 8.538419263543522320, 16.46158073645647235 ) ) ;
#13228=CARTESIAN_POINT ( 'NONE',  ( 68.40000000109249356, 9.143825827087052716, 12.93301269999999192 ) ) ;
#13229=CARTESIAN_POINT ( 'NONE',  ( -66.90000000109246514, 7.933012699999995476, 14.14382582708705094 ) ) ;
#13256=CARTESIAN_POINT ( 'NONE',  ( -70.25000000218494733, 8.964466094067258695, 17.50000000000000355 ) ) ;
#13259=CARTESIAN_POINT ( 'NONE',  ( 67.20000000000000284, 8.232233047033629347, 13.23223304703362402 ) ) ;
#13260=CARTESIAN_POINT ( 'NONE',  ( -71.14999999999999147, 7.499999999999996447, 13.96446609406725514 ) ) ;
#13264=CARTESIAN_POINT ( 'NONE',  ( 68.70000000218495018, 8.232233047033627571, 16.76776695296636532 ) ) ;
#13266=CARTESIAN_POINT ( 'NONE',  ( -69.89999999999999147, 12.50000000000000000, 14.99999999999999645 ) ) ;
#13271=ORIENTED_EDGE ( 'NONE', *, *, #4767, .T. ) ;
#13279=CARTESIAN_POINT ( 'NONE',  ( 70.85000000109246798, 9.999999999999998224, 12.93301269999999192 ) ) ;
#13312=CARTESIAN_POINT ( 'NONE',  ( 72.50000000000000000, 9.999999999999998224, 17.49999999999999645 ) ) ;
#13313=CARTESIAN_POINT ( 'NONE',  ( 70.05000000109247082, 7.933012699999995476, 14.99999999999999645 ) ) ;
#13320=CARTESIAN_POINT ( 'NONE',  ( 67.20000000109247651, 10.85617417291294551, 17.06698729999999742 ) ) ;
#13330=CARTESIAN_POINT ( 'NONE',  ( -66.95000000109246230, 11.46158073645647235, 13.53841926354352232 ) ) ;
#13331=ORIENTED_EDGE ( 'NONE', *, *, #16314, .F. ) ;
#13333=CARTESIAN_POINT ( 'NONE',  ( -70.65000000109246514, 9.999999999999998224, 17.06698730000000097 ) ) ;
#13335=ORIENTED_EDGE ( 'NONE', *, *, #22427, .F. ) ;
#13343=CARTESIAN_POINT ( 'NONE',  ( -67.40000000109247935, 7.933012699999995476, 15.85617417291294196 ) ) ;
#13345=CARTESIAN_POINT ( 'NONE',  ( 67.65000000109247935, 9.999999999999998224, 12.93301269999999192 ) ) ;
#13347=CARTESIAN_POINT ( 'NONE',  ( -65.95000000109246230, 8.538419263543522320, 16.46158073645647235 ) ) ;
#13357=CARTESIAN_POINT ( 'NONE',  ( -69.40000000218495302, 9.999999999999998224, 17.49999999999999645 ) ) ;
#13372=CARTESIAN_POINT ( 'NONE',  ( -69.70000000218495018, 8.232233047033629347, 13.23223304703362402 ) ) ;
#13377=CARTESIAN_POINT ( 'NONE',  ( 67.95000000000000284, 7.499999999999995559, 13.96446609406725692 ) ) ;
#13379=EDGE_CURVE ( 'NONE', #17245, #7757, #7974, .T. ) ;
#13383=CARTESIAN_POINT ( 'NONE',  ( -67.09999999999999432, 7.499999999999996447, 14.99999999999999645 ) ) ;
#13388=CARTESIAN_POINT ( 'NONE',  ( -70.30000000109247082, 10.85617417291294551, 12.93301269999999192 ) ) ;
#13392=VERTEX_POINT ( 'NONE', #13494 ) ;
#13395=CARTESIAN_POINT ( 'NONE',  ( -70.00000000109248788, 9.143825827087050939, 12.93301269999999370 ) ) ;
#13404=CARTESIAN_POINT ( 'NONE',  ( 69.55000000109247082, 11.46158073645647235, 16.46158073645647235 ) ) ;
#13407=CARTESIAN_POINT ( 'NONE',  ( 70.95000000109247651, 8.538419263543524096, 13.53841926354352054 ) ) ;
#13413=CARTESIAN_POINT ( 'NONE',  ( 66.60000000218495586, 9.999999999999998224, 12.49999999999999289 ) ) ;
#13419=FACE_OUTER_BOUND ( 'NONE', #23357, .T. ) ;
#13424=VERTEX_POINT ( 'NONE', #4606 ) ;
#13425=CARTESIAN_POINT ( 'NONE',  ( 69.40000000218495302, 9.999999999999998224, 17.49999999999999645 ) ) ;
#13431=LINE ( 'NONE', #2256, #12229 ) ;
#13432=ORIENTED_EDGE ( 'NONE', *, *, #2865, .F. ) ;
#13433=CARTESIAN_POINT ( 'NONE',  ( 71.45000000109247651, 7.933012699999995476, 14.99999999999999645 ) ) ;
#13440=CARTESIAN_POINT ( 'NONE',  ( 69.35000000109246798, 8.538419263543524096, 13.53841926354352054 ) ) ;
#13442=AXIS2_PLACEMENT_3D ( 'NONE', #15779, #10509, #12416 ) ;
#13445=CARTESIAN_POINT ( 'NONE',  ( 71.05000000109245661, 9.999999999999998224, 12.93301269999999192 ) ) ;
#13453=ORIENTED_EDGE ( 'NONE', *, *, #1294, .F. ) ;
#13455=CARTESIAN_POINT ( 'NONE',  ( -66.85000000109248219, 9.999999999999998224, 12.93301269999999192 ) ) ;
#13458=CARTESIAN_POINT ( 'NONE',  ( -67.30000000109247082, 12.06698730000000275, 15.85617417291294196 ) ) ;
#13464=ORIENTED_EDGE ( 'NONE', *, *, #13604, .F. ) ;
#13468=CARTESIAN_POINT ( 'NONE',  ( -66.30000000109247082, 12.06698730000000275, 15.85617417291294196 ) ) ;
#13469=CARTESIAN_POINT ( 'NONE',  ( 69.55000000109247082, 11.46158073645647235, 16.46158073645647235 ) ) ;
#13470=CARTESIAN_POINT ( 'NONE',  ( -72.35000000000000853, 12.50000000000000000, 16.03553390593273420 ) ) ;
#13493=CARTESIAN_POINT ( 'NONE',  ( -71.05000000218495870, 8.964466094067258695, 17.50000000000000355 ) ) ;
#13494=CARTESIAN_POINT ( 'NONE',  ( -69.00000000218494733, 9.999999999999998224, 12.49999999999999289 ) ) ;
#13498=CARTESIAN_POINT ( 'NONE',  ( 71.25000000109248788, 9.999999999999998224, 17.06698730000000097 ) ) ;
#13504=CARTESIAN_POINT ( 'NONE',  ( -70.70000000109247651, 9.143825827087049163, 17.06698730000000097 ) ) ;
#13510=CARTESIAN_POINT ( 'NONE',  ( -70.05000000109247082, 9.999999999999998224, 12.93301269999999192 ) ) ;
#13518=CARTESIAN_POINT ( 'NONE',  ( 69.00000000109247367, 7.933012699999995476, 15.85617417291294196 ) ) ;
#13519=CARTESIAN_POINT ( 'NONE',  ( 67.65000000109247935, 7.933012699999995476, 14.99999999999999645 ) ) ;
#13524=DIRECTION ( 'NONE',  ( -1.000000000000000000, -0.000000000000000000, -0.000000000000000000 ) ) ;
#13542=CARTESIAN_POINT ( 'NONE',  ( 70.95000000109247651, 11.46158073645647235, 13.53841926354352232 ) ) ;
#13546=ORIENTED_EDGE ( 'NONE', *, *, #8298, .T. ) ;
#13548=CARTESIAN_POINT ( 'NONE',  ( 71.00000000109247367, 9.143825827087052716, 12.93301269999999192 ) ) ;
#13551=CARTESIAN_POINT ( 'NONE',  ( 72.50000000000000000, 9.999999999999998224, 12.49999999999999289 ) ) ;
#13553=CARTESIAN_POINT ( 'NONE',  ( 68.85000000109246798, 12.06698730000000097, 14.99999999999999645 ) ) ;
#13564=CARTESIAN_POINT ( 'NONE',  ( -66.35000000109248219, 11.46158073645647235, 16.46158073645647235 ) ) ;
#13566=CARTESIAN_POINT ( 'NONE',  ( -68.20000000109246230, 10.85617417291294551, 17.06698729999999742 ) ) ;
#13573=CARTESIAN_POINT ( 'NONE',  ( -69.25000000109247367, 9.999999999999998224, 12.93301269999999192 ) ) ;
#13575=CARTESIAN_POINT ( 'NONE',  ( 68.25000000109247367, 7.933012699999995476, 14.99999999999999645 ) ) ;
#13578=CARTESIAN_POINT ( 'NONE',  ( -67.40000000109247935, 10.85617417291294551, 17.06698729999999742 ) ) ;
#13595=EDGE_LOOP ( 'NONE', ( #11719, #10640, #2164, #15598, #17967, #8151, #15232, #3295, #9124, #20570, #7838, #6344, #15159, #1529, #13432, #8068, #3534, #16329, #1412 ) ) ;
#13604=EDGE_CURVE ( 'NONE', #17274, #7791, #22014, .T. ) ;
#13606=CARTESIAN_POINT ( 'NONE',  ( 66.29999999999999716, 7.499999999999996447, 14.99999999999999645 ) ) ;
#13609=CARTESIAN_POINT ( 'NONE',  ( 68.10000000109246798, 9.143825827087049163, 17.06698729999999742 ) ) ;
#13611=CARTESIAN_POINT ( 'NONE',  ( 70.85000000218494165, 12.50000000000000000, 16.03553390593273775 ) ) ;
#13618=CARTESIAN_POINT ( 'NONE',  ( -68.10000000109246798, 12.06698729999999919, 15.85617417291294196 ) ) ;
#13621=ORIENTED_EDGE ( 'NONE', *, *, #6464, .T. ) ;
#13633=CARTESIAN_POINT ( 'NONE',  ( 67.90000000109246514, 12.06698730000000275, 15.85617417291294196 ) ) ;
#13634=CARTESIAN_POINT ( 'NONE',  ( 67.95000000109247651, 11.46158073645647235, 13.53841926354352232 ) ) ;
#13655=VERTEX_POINT ( 'NONE', #16650 ) ;
#13660=CARTESIAN_POINT ( 'NONE',  ( 69.80000000218494449, 9.999999999999998224, 12.49999999999999289 ) ) ;
#13661=MANIFOLD_SOLID_BREP ( 'Mirror2', #14697 ) ;
#13664=CARTESIAN_POINT ( 'NONE',  ( 66.75000000109245946, 8.538419263543522320, 16.46158073645647235 ) ) ;
#13666=CARTESIAN_POINT ( 'NONE',  ( -68.75000000218494733, 7.499999999999996447, 16.03553390593273775 ) ) ;
#13670=CARTESIAN_POINT ( 'NONE',  ( 71.35000000109246798, 11.46158073645647235, 16.46158073645647235 ) ) ;
#13673=EDGE_CURVE ( 'NONE', #3210, #9951, #9607, .T. ) ;
#13680=ORIENTED_EDGE ( 'NONE', *, *, #14033, .F. ) ;
#13681=CARTESIAN_POINT ( 'NONE',  ( -65.70000000109247651, 9.143825827087049163, 17.06698730000000097 ) ) ;
#13684=CARTESIAN_POINT ( 'NONE',  ( -69.25000000109245946, 7.933012699999995476, 14.99999999999999645 ) ) ;
#13687=ORIENTED_EDGE ( 'NONE', *, *, #17482, .F. ) ;
#13692=VECTOR ( 'NONE', #19228, 1000.000000000000000 ) ;
#13693=VECTOR ( 'NONE', #22735, 1000.000000000000000 ) ;
#13695=CARTESIAN_POINT ( 'NONE',  ( 66.95000000109246230, 11.46158073645647235, 13.53841926354352232 ) ) ;
#13696=CARTESIAN_POINT ( 'NONE',  ( -68.10000000109245377, 12.06698730000000275, 15.85617417291294196 ) ) ;
#13699=LINE ( 'NONE', #9750, #14288 ) ;
#13702=CARTESIAN_POINT ( 'NONE',  ( 71.34999999999999432, 11.03553390593268269, 12.49999999999994138 ) ) ;
#13721=CARTESIAN_POINT ( 'NONE',  ( -71.25000000218494733, 7.499999999999995559, 13.96446609406725692 ) ) ;
#13729=CARTESIAN_POINT ( 'NONE',  ( 70.15000000109247935, 11.46158073645647235, 13.53841926354352232 ) ) ;
#13734=CARTESIAN_POINT ( 'NONE',  ( -67.85000000109246798, 9.999999999999998224, 12.93301269999999192 ) ) ;
#13751=VECTOR ( 'NONE', #19375, 1000.000000000000000 ) ;
#13753=CARTESIAN_POINT ( 'NONE',  ( 66.95000000109246230, 11.46158073645647235, 13.53841926354352232 ) ) ;
#13755=CARTESIAN_POINT ( 'NONE',  ( 68.65000000109246514, 9.999999999999998224, 12.93301269999999192 ) ) ;
#13759=( BOUNDED_CURVE ( )  B_SPLINE_CURVE ( 2, ( #18022, #1598, #400, #43, #16694, #13003, #16464, #11206, #13123 ),
 .UNSPECIFIED., .F., .F. ) 
 B_SPLINE_CURVE_WITH_KNOTS ( ( 3, 2, 2, 2, 3 ),
 ( 0.3125000000000002776, 0.3281250000000001665, 0.3437500000000001110, 0.3593750000000000000, 0.3749999999999998890 ),
 .UNSPECIFIED. ) 
 CURVE ( )  GEOMETRIC_REPRESENTATION_ITEM ( )  RATIONAL_B_SPLINE_CURVE ( ( 0.9999999999999986677, 0.9238795325112880708, 1.000000000000000000, 0.9238795325112867385, 1.000000000000000000, 0.9238795325112867385, 1.000000000000000000, 0.9238795325112872936, 0.9999999999999994449 ) ) 
 REPRESENTATION_ITEM ( '' )  );
#13784=CARTESIAN_POINT ( 'NONE',  ( 71.35000000109246798, 8.538419263543522320, 16.46158073645647235 ) ) ;
#13787=CARTESIAN_POINT ( 'NONE',  ( 70.90000000218495302, 11.76776695296636888, 16.76776695296636532 ) ) ;
#13791=CARTESIAN_POINT ( 'NONE',  ( 68.05000000109247082, 12.06698730000000097, 14.99999999999999645 ) ) ;
#13796=CARTESIAN_POINT ( 'NONE',  ( 68.70000000109246230, 10.85617417291294551, 12.93301269999999370 ) ) ;
#13810=CARTESIAN_POINT ( 'NONE',  ( -69.05000000109247082, 9.999999999999998224, 17.06698730000000097 ) ) ;
#13823=CARTESIAN_POINT ( 'NONE',  ( 66.90000000109247935, 10.85617417291294551, 12.93301269999999192 ) ) ;
#13824=CARTESIAN_POINT ( 'NONE',  ( -70.25000000000000000, 7.499999999999995559, 16.03553390593273420 ) ) ;
#13847=CARTESIAN_POINT ( 'NONE',  ( -66.60000000218495586, 9.999999999999998224, 12.49999999999999289 ) ) ;
#13849=CARTESIAN_POINT ( 'NONE',  ( -71.85000000109246798, 9.999999999999998224, 12.93301269999999192 ) ) ;
#13850=CARTESIAN_POINT ( 'NONE',  ( 66.34999999999999432, 7.499999999999995559, 13.96446609406725692 ) ) ;
#13853=CARTESIAN_POINT ( 'NONE',  ( 69.40000000109249356, 12.06698730000000275, 14.14382582708705094 ) ) ;
#13857=CARTESIAN_POINT ( 'NONE',  ( 67.80000000218494449, 9.999999999999998224, 17.49999999999999645 ) ) ;
#13859=CARTESIAN_POINT ( 'NONE',  ( -69.00000000109245946, 10.85617417291294551, 17.06698730000000097 ) ) ;
#13862=CARTESIAN_POINT ( 'NONE',  ( 65.40000000218495302, 9.999999999999998224, 17.49999999999999645 ) ) ;
#13864=PLANE ( 'NONE',  #13442 ) ;
#13874=CARTESIAN_POINT ( 'NONE',  ( 67.65000000109247935, 9.999999999999998224, 12.93301269999999192 ) ) ;
#13875=CARTESIAN_POINT ( 'NONE',  ( 69.00000000109245946, 10.85617417291294551, 17.06698729999999742 ) ) ;
#13882=CARTESIAN_POINT ( 'NONE',  ( 68.20000000218495018, 9.999999999999998224, 12.49999999999999289 ) ) ;
#13896=CARTESIAN_POINT ( 'NONE',  ( 71.15000000109247935, 11.46158073645647235, 16.46158073645647235 ) ) ;
#13897=CARTESIAN_POINT ( 'NONE',  ( 70.00000000218494733, 12.50000000000000000, 14.99999999999999645 ) ) ;
#13901=CARTESIAN_POINT ( 'NONE',  ( 65.95000000109246230, 8.538419263543522320, 16.46158073645647235 ) ) ;
#13904=DIRECTION ( 'NONE',  ( -1.000000000000000000, -0.000000000000000000, -0.000000000000000000 ) ) ;
#13907=CARTESIAN_POINT ( 'NONE',  ( 70.40000000109247935, 12.06698730000000275, 14.14382582708705094 ) ) ;
#13921=ORIENTED_EDGE ( 'NONE', *, *, #12495, .F. ) ;
#13922=CARTESIAN_POINT ( 'NONE',  ( -66.10000000109246798, 7.933012699999995476, 14.14382582708705094 ) ) ;
#13924=EDGE_LOOP ( 'NONE', ( #19801, #4910, #21835, #22377 ) ) ;
#13933=CARTESIAN_POINT ( 'NONE',  ( 65.80000000109247082, 7.933012699999995476, 15.85617417291294196 ) ) ;
#13934=CARTESIAN_POINT ( 'NONE',  ( -70.20000000000000284, 8.232233047033627571, 16.76776695296636532 ) ) ;
#13940=CARTESIAN_POINT ( 'NONE',  ( 71.45000000000000284, 12.50000000000000000, 13.96446609406725692 ) ) ;
#13949=CARTESIAN_POINT ( 'NONE',  ( -71.55000000109247082, 8.538419263543524096, 13.53841926354352054 ) ) ;
#13957=CARTESIAN_POINT ( 'NONE',  ( -66.25000000218494733, 8.964466094067258695, 17.50000000000000355 ) ) ;
#13958=DIRECTION ( 'NONE',  ( -1.000000000000000000, -0.000000000000000000, -0.000000000000000000 ) ) ;
#13959=CARTESIAN_POINT ( 'NONE',  ( -71.80000000109245661, 9.143825827087050939, 12.93301269999999370 ) ) ;
#13963=CARTESIAN_POINT ( 'NONE',  ( 69.15000000109247935, 8.538419263543524096, 13.53841926354352054 ) ) ;
#13964=CARTESIAN_POINT ( 'NONE',  ( 70.75000000218496155, 12.50000000000000000, 13.96446609406725692 ) ) ;
#13967=CARTESIAN_POINT ( 'NONE',  ( 67.65000000218496723, 12.50000000000000000, 16.03553390593273775 ) ) ;
#13969=CARTESIAN_POINT ( 'NONE',  ( -68.85000000109246798, 12.06698730000000097, 14.99999999999999645 ) ) ;
#13973=CARTESIAN_POINT ( 'NONE',  ( 65.45000000218495018, 8.964466094067260471, 17.50000000000000355 ) ) ;
#13981=CARTESIAN_POINT ( 'NONE',  ( -66.90000000000000568, 9.999999999999998224, 17.49999999999999645 ) ) ;
#13985=CARTESIAN_POINT ( 'NONE',  ( 67.85000000109246798, 9.999999999999998224, 12.93301269999999192 ) ) ;
#14013=CARTESIAN_POINT ( 'NONE',  ( 66.00000000109245946, 7.933012699999995476, 15.85617417291294196 ) ) ;
#14015=CARTESIAN_POINT ( 'NONE',  ( -68.80000000218494449, 7.499999999999996447, 14.99999999999999645 ) ) ;
#14017=CARTESIAN_POINT ( 'NONE',  ( 66.80000000109247082, 7.933012699999995476, 15.85617417291294196 ) ) ;
#14025=VERTEX_POINT ( 'NONE', #18065 ) ;
#14027=EDGE_LOOP ( 'NONE', ( #8672, #14753, #14512, #928, #3010, #16181, #2779, #12187 ) ) ;
#14031=ORIENTED_EDGE ( 'NONE', *, *, #22166, .F. ) ;
#14033=EDGE_CURVE ( 'NONE', #13655, #14025, #3325, .T. ) ;
#14037=CARTESIAN_POINT ( 'NONE',  ( -66.70000000218495018, 11.76776695296636888, 13.23223304703362579 ) ) ;
#14038=CARTESIAN_POINT ( 'NONE',  ( 66.55000000109247082, 8.538419263543522320, 16.46158073645647235 ) ) ;
#14039=EDGE_CURVE ( 'NONE', #11744, #18480, #6508, .T. ) ;
#14040=CARTESIAN_POINT ( 'NONE',  ( -68.84999999999999432, 8.964466094067258695, 12.49999999999999289 ) ) ;
#14053=CARTESIAN_POINT ( 'NONE',  ( -68.10000000109246798, 9.143825827087049163, 17.06698729999999742 ) ) ;
#14057=ORIENTED_EDGE ( 'NONE', *, *, #11282, .T. ) ;
#14059=AXIS2_PLACEMENT_3D ( 'NONE', #3297, #10639, #18382 ) ;
#14068=CARTESIAN_POINT ( 'NONE',  ( -67.45000000218493597, 11.03553390593273598, 12.49999999999999289 ) ) ;
#14083=CARTESIAN_POINT ( 'NONE',  ( 67.59999999999999432, 11.76776695296636888, 16.76776695296636532 ) ) ;
#14084=EDGE_LOOP ( 'NONE', ( #230, #17933, #22462, #23314 ) ) ;
#14091=VERTEX_POINT ( 'NONE', #18179 ) ;
#14107=CARTESIAN_POINT ( 'NONE',  ( 72.09999999999999432, 9.999999999999998224, 12.49999999999999289 ) ) ;
#14114=CARTESIAN_POINT ( 'NONE',  ( 72.50000000000000000, 9.999999999999998224, 14.99999999999999645 ) ) ;
#14120=CARTESIAN_POINT ( 'NONE',  ( 68.20000000000000284, 11.76776695296636888, 13.23223304703362579 ) ) ;
#14124=CARTESIAN_POINT ( 'NONE',  ( 71.95000000109247651, 11.46158073645647235, 16.46158073645647235 ) ) ;
#14127=CARTESIAN_POINT ( 'NONE',  ( 66.20000000218495018, 9.999999999999998224, 17.49999999999999645 ) ) ;
#14131=ADVANCED_FACE ( 'NONE', ( #18646 ), #7422, .T. ) ;
#14132=CARTESIAN_POINT ( 'NONE',  ( 67.25000000218494733, 7.499999999999995559, 13.96446609406725692 ) ) ;
#14135=CARTESIAN_POINT ( 'NONE',  ( 67.20000000109246230, 12.06698729999999919, 14.14382582708705094 ) ) ;
#14140=CARTESIAN_POINT ( 'NONE',  ( 66.00000000109245946, 7.933012699999995476, 15.85617417291294196 ) ) ;
#14169=CARTESIAN_POINT ( 'NONE',  ( -70.14999999999999147, 8.964466094067258695, 17.50000000000000355 ) ) ;
#14181=CARTESIAN_POINT ( 'NONE',  ( -71.45000000109247651, 7.933012699999995476, 14.99999999999999645 ) ) ;
#14184=CARTESIAN_POINT ( 'NONE',  ( -66.80000000109247082, 9.143825827087050939, 12.93301269999999370 ) ) ;
#14193=CYLINDRICAL_SURFACE ( 'NONE', #14498, 2.500000000000002220 ) ;
#14196=CARTESIAN_POINT ( 'NONE',  ( -67.00000000218494733, 9.999999999999998224, 17.49999999999999645 ) ) ;
#14198=CARTESIAN_POINT ( 'NONE',  ( -71.75000000109247367, 8.538419263543524096, 13.53841926354352054 ) ) ;
#14200=LINE ( 'NONE', #7245, #6135 ) ;
#14208=CARTESIAN_POINT ( 'NONE',  ( 67.40000000218495302, 9.999999999999998224, 12.49999999999999289 ) ) ;
#14210=VERTEX_POINT ( 'NONE', #20373 ) ;
#14223=CYLINDRICAL_SURFACE ( 'NONE', #15645, 2.500000000000002220 ) ;
#14229=CARTESIAN_POINT ( 'NONE',  ( 66.65000000109247935, 7.933012699999995476, 14.99999999999999645 ) ) ;
#14230=CARTESIAN_POINT ( 'NONE',  ( 71.29999999999998295, 9.999999999999998224, 12.49999999999999289 ) ) ;
#14251=CARTESIAN_POINT ( 'NONE',  ( -69.39999999999999147, 8.232233047033627571, 16.76776695296636532 ) ) ;
#14255=CARTESIAN_POINT ( 'NONE',  ( 66.70000000218495018, 11.76776695296636888, 13.23223304703362579 ) ) ;
#14258=CARTESIAN_POINT ( 'NONE',  ( 65.85000000109246798, 9.999999999999998224, 17.06698730000000097 ) ) ;
#14263=CARTESIAN_POINT ( 'NONE',  ( 67.75000000109245946, 8.538419263543524096, 13.53841926354352054 ) ) ;
#14287=CARTESIAN_POINT ( 'NONE',  ( -70.54999999999999716, 11.03553390593273598, 12.49999999999999289 ) ) ;
#14288=VECTOR ( 'NONE', #17048, 1000.000000000000000 ) ;
#14292=CARTESIAN_POINT ( 'NONE',  ( 67.35000000218495586, 8.964466094067256918, 12.49999999999999822 ) ) ;
#14293=CARTESIAN_POINT ( 'NONE',  ( 68.09999999999999432, 9.999999999999998224, 12.49999999999999289 ) ) ;
#14300=CARTESIAN_POINT ( 'NONE',  ( -68.80000000109247082, 10.85617417291294551, 17.06698729999999742 ) ) ;
#14302=DIRECTION ( 'NONE',  ( -1.000000000000000000, -0.000000000000000000, -0.000000000000000000 ) ) ;
#14305=AXIS2_PLACEMENT_3D ( 'NONE', #5257, #96, #16292 ) ;
#14308=CARTESIAN_POINT ( 'NONE',  ( -71.92500000163870766, 9.999999999999998224, 17.28349365000000049 ) ) ;
#14312=CARTESIAN_POINT ( 'NONE',  ( -67.20000000218495018, 7.499999999999996447, 14.99999999999999645 ) ) ;
#14319=CARTESIAN_POINT ( 'NONE',  ( 66.94999999999998863, 8.964466094067207180, 17.49999999999995026 ) ) ;
#14323=CARTESIAN_POINT ( 'NONE',  ( -68.45000000000000284, 11.03553390593276617, 17.49999999999997513 ) ) ;
#14344=CARTESIAN_POINT ( 'NONE',  ( 66.10000000109246798, 7.933012699999995476, 14.14382582708705094 ) ) ;
#14355=CARTESIAN_POINT ( 'NONE',  ( -70.45000000218495018, 7.499999999999996447, 13.96446609406725514 ) ) ;
#14358=CARTESIAN_POINT ( 'NONE',  ( 68.45000000000000284, 11.03553390593276617, 17.49999999999997513 ) ) ;
#14363=VERTEX_POINT ( 'NONE', #9128 ) ;
#14364=CARTESIAN_POINT ( 'NONE',  ( 71.10000000218494165, 8.232233047033627571, 16.76776695296636532 ) ) ;
#14366=CARTESIAN_POINT ( 'NONE',  ( 65.85000000218495586, 11.03553390593269867, 12.49999999999995559 ) ) ;
#14373=CARTESIAN_POINT ( 'NONE',  ( 67.75000000218496155, 11.03553390593273598, 17.50000000000000355 ) ) ;
#14378=ORIENTED_EDGE ( 'NONE', *, *, #17482, .T. ) ;
#14409=CARTESIAN_POINT ( 'NONE',  ( -67.74999999999998579, 8.964466094067258695, 17.50000000000000355 ) ) ;
#14414=CARTESIAN_POINT ( 'NONE',  ( -66.15000000109247935, 8.538419263543524096, 13.53841926354352054 ) ) ;
#14419=CARTESIAN_POINT ( 'NONE',  ( -71.30000000109249925, 9.143825827087049163, 17.06698730000000097 ) ) ;
#14422=CARTESIAN_POINT ( 'NONE',  ( -66.70000000109246230, 7.933012699999995476, 14.14382582708705094 ) ) ;
#14428=CARTESIAN_POINT ( 'NONE',  ( 71.00000000000000000, 8.232233047033627571, 16.76776695296636532 ) ) ;
#14431=CARTESIAN_POINT ( 'NONE',  ( -71.85000000109246798, 12.06698730000000097, 14.99999999999999645 ) ) ;
#14432=CARTESIAN_POINT ( 'NONE',  ( -70.45000000109247651, 12.06698730000000097, 14.99999999999999645 ) ) ;
#14452=VERTEX_POINT ( 'NONE', #107 ) ;
#14454=CARTESIAN_POINT ( 'NONE',  ( 66.20000000218495018, 9.999999999999998224, 17.49999999999999645 ) ) ;
#14463=CARTESIAN_POINT ( 'NONE',  ( 65.90000000109246514, 9.143825827087049163, 17.06698729999999742 ) ) ;
#14464=CARTESIAN_POINT ( 'NONE',  ( -65.40000000218495302, 9.999999999999998224, 17.49999999999999645 ) ) ;
#14479=CIRCLE ( 'NONE', #22472, 2.500000000000002220 ) ;
#14486=ORIENTED_EDGE ( 'NONE', *, *, #22569, .T. ) ;
#14490=CARTESIAN_POINT ( 'NONE',  ( 67.15000000218495302, 7.499999999999995559, 16.03553390593273420 ) ) ;
#14493=( BOUNDED_CURVE ( )  B_SPLINE_CURVE ( 2, ( #18502, #11710, #11228, #4135, #6056, #5938, #13264, #20528, #181 ),
 .UNSPECIFIED., .F., .F. ) 
 B_SPLINE_CURVE_WITH_KNOTS ( ( 3, 2, 2, 2, 3 ),
 ( 0.4374999999999995004, 0.4531249999999993894, 0.4687499999999993339, 0.4843749999999992228, 0.4999999999999991118 ),
 .UNSPECIFIED. ) 
 CURVE ( )  GEOMETRIC_REPRESENTATION_ITEM ( )  RATIONAL_B_SPLINE_CURVE ( ( 1.000000000000002442, 0.9238795325112842960, 1.000000000000000000, 0.9238795325112867385, 1.000000000000000000, 0.9238795325112867385, 1.000000000000000000, 0.9238795325112910684, 0.9999999999999956701 ) ) 
 REPRESENTATION_ITEM ( '' )  );
#14498=AXIS2_PLACEMENT_3D ( 'NONE', #6752, #19203, #8452 ) ;
#14502=CARTESIAN_POINT ( 'NONE',  ( 66.50000000109245946, 12.06698730000000275, 15.85617417291294196 ) ) ;
#14511=CARTESIAN_POINT ( 'NONE',  ( -72.45000000000001705, 11.03553390593273953, 17.50000000000000355 ) ) ;
#14512=ORIENTED_EDGE ( 'NONE', *, *, #20893, .F. ) ;
#14519=CARTESIAN_POINT ( 'NONE',  ( 69.70000000000000284, 9.999999999999998224, 12.49999999999999289 ) ) ;
#14531=CARTESIAN_POINT ( 'NONE',  ( -67.59999999999999432, 11.76776695296636888, 16.76776695296636532 ) ) ;
#14538=CARTESIAN_POINT ( 'NONE',  ( -67.40000000109247935, 10.85617417291294551, 17.06698730000000097 ) ) ;
#14544=CARTESIAN_POINT ( 'NONE',  ( -69.55000000109247082, 11.46158073645647235, 16.46158073645647235 ) ) ;
#14547=CARTESIAN_POINT ( 'NONE',  ( -67.20000000109247651, 10.85617417291294551, 17.06698729999999742 ) ) ;
#14549=VECTOR ( 'NONE', #3093, 1000.000000000000000 ) ;
#14557=CARTESIAN_POINT ( 'NONE',  ( -69.70000000109246230, 9.143825827087049163, 17.06698729999999742 ) ) ;
#14559=CARTESIAN_POINT ( 'NONE',  ( -71.55000000109245661, 8.538419263543522320, 16.46158073645647235 ) ) ;
#14589=( GEOMETRIC_REPRESENTATION_CONTEXT ( 3 ) GLOBAL_UNCERTAINTY_ASSIGNED_CONTEXT ( ( #18878 ) ) GLOBAL_UNIT_ASSIGNED_CONTEXT ( ( #10914, #17209, #16757 ) ) REPRESENTATION_CONTEXT ( 'NONE', 'WORKASPACE' ) );
#14590=CARTESIAN_POINT ( 'NONE',  ( 72.20000000000000284, 11.76776695296636888, 13.23223304703362579 ) ) ;
#14602=EDGE_LOOP ( 'NONE', ( #6164, #18400, #9716, #11685 ) ) ;
#14610=CARTESIAN_POINT ( 'NONE',  ( 68.30000000218494449, 11.76776695296636888, 13.23223304703362579 ) ) ;
#14621=CARTESIAN_POINT ( 'NONE',  ( 72.50000000000000000, 9.999999999999998224, 14.99999999999999645 ) ) ;
#14622=CARTESIAN_POINT ( 'NONE',  ( 72.15000000000001990, 11.03553390593275374, 12.50000000000001243 ) ) ;
#14637=( BOUNDED_CURVE ( )  B_SPLINE_CURVE ( 2, ( #9289, #7486, #14804, #13004, #3873, #11207, #18481, #2064, #980 ),
 .UNSPECIFIED., .F., .F. ) 
 B_SPLINE_CURVE_WITH_KNOTS ( ( 3, 2, 2, 2, 3 ),
 ( 0.000000000000000000, 0.01562499999999990459, 0.03124999999999980918, 0.04687499999999971551, 0.06249999999999961836 ),
 .UNSPECIFIED. ) 
 CURVE ( )  GEOMETRIC_REPRESENTATION_ITEM ( )  RATIONAL_B_SPLINE_CURVE ( ( 1.000000000000000000, 0.9238795325112867385, 1.000000000000000000, 0.9238795325112867385, 1.000000000000000000, 0.9238795325112867385, 1.000000000000000000, 0.9238795325112886259, 0.9999999999999981126 ) ) 
 REPRESENTATION_ITEM ( '' )  );
#14642=EDGE_CURVE ( 'NONE', #23001, #4247, #57, .T. ) ;
#14645=CARTESIAN_POINT ( 'NONE',  ( -67.84999999999999432, 7.499999999999995559, 16.03553390593273420 ) ) ;
#14649=CARTESIAN_POINT ( 'NONE',  ( 66.75000000109247367, 8.538419263543524096, 13.53841926354352054 ) ) ;
#14653=CARTESIAN_POINT ( 'NONE',  ( 68.55000000218494449, 11.03553390593269157, 17.50000000000004619 ) ) ;
#14655=DIRECTION ( 'NONE',  ( 0.000000000000000000, 0.000000000000000000, 1.000000000000000000 ) ) ;
#14657=CARTESIAN_POINT ( 'NONE',  ( -68.60000000109248219, 12.06698729999999919, 14.14382582708705094 ) ) ;
#14660=CARTESIAN_POINT ( 'NONE',  ( -65.65000000109247935, 9.999999999999998224, 17.06698730000000097 ) ) ;
#14668=CARTESIAN_POINT ( 'NONE',  ( -71.80000000109247082, 12.06698730000000275, 14.14382582708705094 ) ) ;
#14670=( BOUNDED_CURVE ( )  B_SPLINE_CURVE ( 2, ( #773, #17072, #22799, #13260, #4479, #22436, #4129, #2552, #19211 ),
 .UNSPECIFIED., .F., .F. ) 
 B_SPLINE_CURVE_WITH_KNOTS ( ( 3, 2, 2, 2, 3 ),
 ( 0.1875000000000010270, 0.2031250000000009437, 0.2187500000000008327, 0.2343750000000007494, 0.2500000000000006661 ),
 .UNSPECIFIED. ) 
 CURVE ( )  GEOMETRIC_REPRESENTATION_ITEM ( )  RATIONAL_B_SPLINE_CURVE ( ( 0.9999999999999950040, 0.9238795325112917345, 1.000000000000000000, 0.9238795325112867385, 1.000000000000000000, 0.9238795325112867385, 1.000000000000000000, 0.9238795325112835188, 1.000000000000003331 ) ) 
 REPRESENTATION_ITEM ( '' )  );
#14671=CARTESIAN_POINT ( 'NONE',  ( -71.15000000109246514, 11.46158073645647235, 13.53841926354352232 ) ) ;
#14683=VERTEX_POINT ( 'NONE', #6842 ) ;
#14685=LINE ( 'NONE', #11086, #18151 ) ;
#14694=CARTESIAN_POINT ( 'NONE',  ( 68.99999999999998579, 11.76776695296636888, 13.23223304703362579 ) ) ;
#14697=CLOSED_SHELL ( 'NONE', ( #17278, #20477, #283, #6938, #9645, #21223, #19584, #16645, #20462, #9893, #687, #17871, #23000, #5567, #7901, #8655, #2769, #3237, #17857, #17736, #8360, #8650, #8324, #4500, #17313, #12193, #4234, #12460, #12023, #6839, #22287, #9328, #23381, #3999, #12525, #9765, #18032, #10034, #14131, #3951, #13172, #3235, #2035, #15267, #3359, #8841 ) ) ;
#14701=CARTESIAN_POINT ( 'NONE',  ( 67.74999999999998579, 8.964466094067258695, 17.50000000000000355 ) ) ;
#14724=CARTESIAN_POINT ( 'NONE',  ( 65.80000000218494449, 9.999999999999998224, 12.49999999999999289 ) ) ;
#14735=CARTESIAN_POINT ( 'NONE',  ( 66.90000000218495302, 11.76776695296636888, 16.76776695296636532 ) ) ;
#14753=ORIENTED_EDGE ( 'NONE', *, *, #6906, .T. ) ;
#14765=CARTESIAN_POINT ( 'NONE',  ( 66.90000000109246514, 10.85617417291294551, 12.93301269999999370 ) ) ;
#14775=CARTESIAN_POINT ( 'NONE',  ( -67.55000000109247082, 8.538419263543524096, 13.53841926354352054 ) ) ;
#14778=CARTESIAN_POINT ( 'NONE',  ( -70.75000000109247367, 8.538419263543522320, 16.46158073645647235 ) ) ;
#14780=( BOUNDED_CURVE ( )  B_SPLINE_CURVE ( 2, ( #319, #13052, #2233, #7879, #5836, #15087, #22342, #11136, #14974 ),
 .UNSPECIFIED., .F., .F. ) 
 B_SPLINE_CURVE_WITH_KNOTS ( ( 3, 2, 2, 2, 3 ),
 ( 0.9375000000000007772, 0.9531250000000005551, 0.9687500000000004441, 0.9843750000000002220, 1.000000000000000000 ),
 .UNSPECIFIED. ) 
 CURVE ( )  GEOMETRIC_REPRESENTATION_ITEM ( )  RATIONAL_B_SPLINE_CURVE ( ( 0.9999999999999962252, 0.9238795325112905132, 1.000000000000000000, 0.9238795325112867385, 1.000000000000000000, 0.9238795325112867385, 1.000000000000000000, 0.9238795325112867385, 1.000000000000000000 ) ) 
 REPRESENTATION_ITEM ( '' )  );
#14785=VECTOR ( 'NONE', #20939, 1000.000000000000000 ) ;
#14786=ORIENTED_EDGE ( 'NONE', *, *, #4661, .T. ) ;
#14791=CARTESIAN_POINT ( 'NONE',  ( -71.45000000109247651, 7.933012699999995476, 14.99999999999999645 ) ) ;
#14792=CARTESIAN_POINT ( 'NONE',  ( -70.55000000109245661, 11.46158073645647235, 16.46158073645647235 ) ) ;
#14803=EDGE_CURVE ( 'NONE', #2788, #9234, #2497, .T. ) ;
#14804=CARTESIAN_POINT ( 'NONE',  ( -71.70000000218495018, 11.76776695296636888, 16.76776695296636532 ) ) ;
#14810=VERTEX_POINT ( 'NONE', #21517 ) ;
#14813=CARTESIAN_POINT ( 'NONE',  ( 69.29999999999999716, 9.999999999999998224, 17.49999999999999645 ) ) ;
#14819=CARTESIAN_POINT ( 'NONE',  ( 67.45000000000000284, 12.50000000000000000, 13.96446609406725869 ) ) ;
#14825=CARTESIAN_POINT ( 'NONE',  ( -71.79999999999998295, 8.232233047033627571, 16.76776695296636532 ) ) ;
#14844=CARTESIAN_POINT ( 'NONE',  ( 70.40000000109250777, 10.85617417291294551, 17.06698729999999742 ) ) ;
#14846=PLANE ( 'NONE',  #5355 ) ;
#14847=CARTESIAN_POINT ( 'NONE',  ( 70.65000000109246514, 9.999999999999998224, 17.06698730000000097 ) ) ;
#14856=CARTESIAN_POINT ( 'NONE',  ( 72.39999999999999147, 11.76776695296636888, 16.76776695296636532 ) ) ;
#14859=EDGE_LOOP ( 'NONE', ( #14378, #21126 ) ) ;
#14866=CARTESIAN_POINT ( 'NONE',  ( 70.50000000000000000, 9.999999999999998224, 12.49999999999999289 ) ) ;
#14882=CARTESIAN_POINT ( 'NONE',  ( 70.10000000109246798, 7.933012699999995476, 14.14382582708705094 ) ) ;
#14886=CARTESIAN_POINT ( 'NONE',  ( 68.05000000109247082, 9.999999999999998224, 17.06698730000000097 ) ) ;
#14893=CARTESIAN_POINT ( 'NONE',  ( -67.05000000218494449, 8.964466094067246260, 17.49999999999999289 ) ) ;
#14896=CARTESIAN_POINT ( 'NONE',  ( -70.00000000109247367, 9.143825827087052716, 12.93301269999999192 ) ) ;
#14899=CARTESIAN_POINT ( 'NONE',  ( -71.45000000109247651, 9.999999999999998224, 17.06698730000000097 ) ) ;
#14908=CARTESIAN_POINT ( 'NONE',  ( -69.85000000109248219, 7.933012699999995476, 14.99999999999999645 ) ) ;
#14911=CARTESIAN_POINT ( 'NONE',  ( -69.05000000109247082, 9.999999999999998224, 17.06698730000000097 ) ) ;
#14916=CARTESIAN_POINT ( 'NONE',  ( 72.04999999999998295, 8.964466094067278235, 12.49999999999997691 ) ) ;
#14925=CARTESIAN_POINT ( 'NONE',  ( -69.35000000218497007, 11.03553390593273420, 17.50000000000000711 ) ) ;
#14944=CARTESIAN_POINT ( 'NONE',  ( 68.29999999999999716, 12.50000000000000000, 14.99999999999999645 ) ) ;
#14949=AXIS2_PLACEMENT_3D ( 'NONE', #7812, #489, #14655 ) ;
#14955=CARTESIAN_POINT ( 'NONE',  ( -71.65000000109246514, 7.933012699999995476, 14.99999999999999645 ) ) ;
#14971=MECHANICAL_DESIGN_GEOMETRIC_PRESENTATION_REPRESENTATION('',(#13049),#9612);
#14973=CARTESIAN_POINT ( 'NONE',  ( 65.40000000218495302, 9.999999999999998224, 17.49999999999999645 ) ) ;
#14974=CARTESIAN_POINT ( 'NONE',  ( 66.09999999999999432, 9.999999999999998224, 17.49999999999999645 ) ) ;
#14975=CARTESIAN_POINT ( 'NONE',  ( 71.80000000109245661, 9.143825827087050939, 12.93301269999999370 ) ) ;
#14990=CARTESIAN_POINT ( 'NONE',  ( -69.90000000218495302, 11.76776695296636888, 13.23223304703362579 ) ) ;
#14995=CARTESIAN_POINT ( 'NONE',  ( 70.79999999999999716, 11.76776695296636888, 16.76776695296636532 ) ) ;
#15006=CARTESIAN_POINT ( 'NONE',  ( 69.30000000109247082, 7.933012699999995476, 14.14382582708705094 ) ) ;
#15010=CARTESIAN_POINT ( 'NONE',  ( 65.65000000109247935, 9.999999999999998224, 17.06698730000000097 ) ) ;
#15016=CARTESIAN_POINT ( 'NONE',  ( -71.25000000218494733, 7.499999999999996447, 13.96446609406725514 ) ) ;
#15020=CARTESIAN_POINT ( 'NONE',  ( -69.35000000109248219, 11.46158073645647235, 13.53841926354352232 ) ) ;
#15023=CARTESIAN_POINT ( 'NONE',  ( -71.40000000109246514, 10.85617417291294551, 17.06698729999999742 ) ) ;
#15027=VERTEX_POINT ( 'NONE', #17430 ) ;
#15030=CARTESIAN_POINT ( 'NONE',  ( -68.05000000109247082, 9.999999999999998224, 17.06698730000000097 ) ) ;
#15031=CARTESIAN_POINT ( 'NONE',  ( 69.00000000109247367, 7.933012699999995476, 15.85617417291294196 ) ) ;
#15032=CARTESIAN_POINT ( 'NONE',  ( -67.00000000109247367, 9.143825827087050939, 12.93301269999999370 ) ) ;
#15038=LINE ( 'NONE', #748, #10141 ) ;
#15056=ORIENTED_EDGE ( 'NONE', *, *, #15403, .T. ) ;
#15057=CARTESIAN_POINT ( 'NONE',  ( -69.35000000218495586, 11.03553390593273598, 17.50000000000000355 ) ) ;
#15059=CARTESIAN_POINT ( 'NONE',  ( 68.09999999999999432, 9.999999999999998224, 12.49999999999999289 ) ) ;
#15068=CARTESIAN_POINT ( 'NONE',  ( -72.00000000109248788, 12.06698729999999919, 14.14382582708705094 ) ) ;
#15069=CARTESIAN_POINT ( 'NONE',  ( -70.04999999999999716, 11.03553390593273420, 17.50000000000000711 ) ) ;
#15071=CARTESIAN_POINT ( 'NONE',  ( 72.50000000000000000, 9.999999999999998224, 14.99999999999999645 ) ) ;
#15072=FACE_OUTER_BOUND ( 'NONE', #9086, .T. ) ;
#15073=CARTESIAN_POINT ( 'NONE',  ( -70.20000000109246230, 12.06698730000000275, 14.14382582708705094 ) ) ;
#15086=CARTESIAN_POINT ( 'NONE',  ( 71.00000000109247367, 12.06698730000000275, 14.14382582708705094 ) ) ;
#15087=CARTESIAN_POINT ( 'NONE',  ( 66.24999999999998579, 7.499999999999996447, 16.03553390593273775 ) ) ;
#15088=CARTESIAN_POINT ( 'NONE',  ( 72.00000000109245946, 12.06698730000000275, 14.14382582708705094 ) ) ;
#15097=CARTESIAN_POINT ( 'NONE',  ( -65.90000000109247935, 9.143825827087049163, 17.06698730000000097 ) ) ;
#15104=CARTESIAN_POINT ( 'NONE',  ( 70.59999999999999432, 11.76776695296636888, 13.23223304703362579 ) ) ;
#15117=CARTESIAN_POINT ( 'NONE',  ( 70.25000000109245946, 9.999999999999998224, 12.93301269999999192 ) ) ;
#15121=CARTESIAN_POINT ( 'NONE',  ( 67.00000000109247367, 12.06698730000000275, 14.14382582708705094 ) ) ;
#15130=CARTESIAN_POINT ( 'NONE',  ( -67.40000000218495302, 9.999999999999998224, 12.49999999999999289 ) ) ;
#15135=CARTESIAN_POINT ( 'NONE',  ( -71.50000000109247367, 9.143825827087049163, 17.06698729999999742 ) ) ;
#15146=CARTESIAN_POINT ( 'NONE',  ( -66.40000000109247935, 10.85617417291294551, 17.06698729999999742 ) ) ;
#15148=CARTESIAN_POINT ( 'NONE',  ( 69.95000000109247651, 8.538419263543524096, 13.53841926354352054 ) ) ;
#15149=CARTESIAN_POINT ( 'NONE',  ( -66.10000000109246798, 7.933012699999995476, 14.14382582708705094 ) ) ;
#15156=CARTESIAN_POINT ( 'NONE',  ( -69.05000000218494449, 11.03553390593276262, 12.50000000000001776 ) ) ;
#15157=ORIENTED_EDGE ( 'NONE', *, *, #18126, .F. ) ;
#15159=ORIENTED_EDGE ( 'NONE', *, *, #18738, .F. ) ;
#15166=EDGE_LOOP ( 'NONE', ( #3641, #1926, #6248, #807 ) ) ;
#15177=CARTESIAN_POINT ( 'NONE',  ( 68.54999999999999716, 8.964466094067258695, 17.50000000000000355 ) ) ;
#15179=CARTESIAN_POINT ( 'NONE',  ( -67.24999999999998579, 8.964466094067294222, 12.49999999999996092 ) ) ;
#15184=CARTESIAN_POINT ( 'NONE',  ( -70.65000000109246514, 9.999999999999998224, 17.06698730000000097 ) ) ;
#15189=CARTESIAN_POINT ( 'NONE',  ( -70.60000000109246798, 7.933012699999995476, 15.85617417291294196 ) ) ;
#15192=LINE ( 'NONE', #18511, #11020 ) ;
#15196=CARTESIAN_POINT ( 'NONE',  ( 65.50000000218494733, 8.232233047033627571, 16.76776695296636532 ) ) ;
#15198=CARTESIAN_POINT ( 'NONE',  ( 69.90000000109246514, 9.143825827087049163, 17.06698729999999742 ) ) ;
#15208=CARTESIAN_POINT ( 'NONE',  ( -66.20000000109246230, 9.143825827087052716, 12.93301269999999192 ) ) ;
#15231=CARTESIAN_POINT ( 'NONE',  ( 72.00000000109248788, 12.06698729999999919, 14.14382582708705094 ) ) ;
#15232=ORIENTED_EDGE ( 'NONE', *, *, #3903, .F. ) ;
#15238=CARTESIAN_POINT ( 'NONE',  ( 68.75000000109245946, 11.46158073645647235, 13.53841926354352232 ) ) ;
#15252=CARTESIAN_POINT ( 'NONE',  ( -68.05000000109247082, 12.06698730000000097, 14.99999999999999645 ) ) ;
#15263=CARTESIAN_POINT ( 'NONE',  ( -69.20000000109246230, 9.143825827087050939, 12.93301269999999370 ) ) ;
#15264=CARTESIAN_POINT ( 'NONE',  ( 68.80000000109247082, 10.85617417291294551, 17.06698730000000097 ) ) ;
#15265=CARTESIAN_POINT ( 'NONE',  ( -68.35000000109246798, 8.538419263543522320, 16.46158073645647235 ) ) ;
#15267=ADVANCED_FACE ( 'NONE', ( #5187 ), #2074, .F. ) ;
#15278=CARTESIAN_POINT ( 'NONE',  ( 65.40000000218495302, 9.999999999999998224, 17.49999999999999645 ) ) ;
#15287=CARTESIAN_POINT ( 'NONE',  ( 67.40000000218495302, 9.999999999999998224, 12.49999999999999289 ) ) ;
#15291=CARTESIAN_POINT ( 'NONE',  ( -69.95000000218493597, 12.50000000000000000, 13.96446609406725869 ) ) ;
#15296=CARTESIAN_POINT ( 'NONE',  ( 66.15000000000000568, 8.964466094067258695, 17.50000000000000355 ) ) ;
#15297=VECTOR ( 'NONE', #18446, 1000.000000000000000 ) ;
#15299=CARTESIAN_POINT ( 'NONE',  ( 69.45000000109247651, 12.06698730000000097, 14.99999999999999645 ) ) ;
#15307=CARTESIAN_POINT ( 'NONE',  ( -72.20000000109246230, 10.85617417291294551, 17.06698730000000097 ) ) ;
#15309=CARTESIAN_POINT ( 'NONE',  ( 65.60000000218495586, 7.499999999999996447, 14.99999999999999645 ) ) ;
#15314=CARTESIAN_POINT ( 'NONE',  ( -70.75000000109247367, 8.538419263543524096, 13.53841926354352054 ) ) ;
#15318=CARTESIAN_POINT ( 'NONE',  ( 72.50000000000000000, 9.999999999999998224, 17.49999999999999645 ) ) ;
#15325=CARTESIAN_POINT ( 'NONE',  ( 68.85000000109248219, 9.999999999999998224, 17.06698730000000097 ) ) ;
#15327=CARTESIAN_POINT ( 'NONE',  ( 67.40000000109247935, 10.85617417291294551, 17.06698729999999742 ) ) ;
#15341=ORIENTED_EDGE ( 'NONE', *, *, #8978, .T. ) ;
#15353=CARTESIAN_POINT ( 'NONE',  ( 70.80000000218494449, 12.50000000000000000, 14.99999999999999645 ) ) ;
#15355=( NAMED_UNIT ( * ) SI_UNIT ( $, .STERADIAN. ) SOLID_ANGLE_UNIT ( ) );
#15356=CARTESIAN_POINT ( 'NONE',  ( 71.10000000109246798, 10.85617417291294551, 12.93301269999999192 ) ) ;
#15362=CARTESIAN_POINT ( 'NONE',  ( 70.00000000109247367, 7.933012699999995476, 15.85617417291294196 ) ) ;
#15372=CARTESIAN_POINT ( 'NONE',  ( -67.35000000109248219, 8.538419263543522320, 16.46158073645647235 ) ) ;
#15375=CARTESIAN_POINT ( 'NONE',  ( -67.35000000109246798, 11.46158073645647235, 16.46158073645647235 ) ) ;
#15386=CARTESIAN_POINT ( 'NONE',  ( -66.45000000109247651, 9.999999999999998224, 17.06698730000000097 ) ) ;
#15387=CARTESIAN_POINT ( 'NONE',  ( 69.70000000109247651, 9.143825827087049163, 17.06698730000000097 ) ) ;
#15389=CARTESIAN_POINT ( 'NONE',  ( -72.44999999999998863, 11.03553390593273598, 17.50000000000000355 ) ) ;
#15403=EDGE_CURVE ( 'NONE', #23070, #4760, #18913, .T. ) ;
#15410=CARTESIAN_POINT ( 'NONE',  ( -70.70000000218495018, 11.76776695296636888, 13.23223304703362579 ) ) ;
#15411=( BOUNDED_CURVE ( )  B_SPLINE_CURVE ( 2, ( #8342, #22690, #12066, #4736, #15309, #6185, #22809, #13973, #13862 ),
 .UNSPECIFIED., .F., .F. ) 
 B_SPLINE_CURVE_WITH_KNOTS ( ( 3, 2, 2, 2, 3 ),
 ( 0.9375000000000007772, 0.9531250000000005551, 0.9687500000000004441, 0.9843750000000002220, 1.000000000000000000 ),
 .UNSPECIFIED. ) 
 CURVE ( )  GEOMETRIC_REPRESENTATION_ITEM ( )  RATIONAL_B_SPLINE_CURVE ( ( 0.9999999999999962252, 0.9238795325112905132, 1.000000000000000000, 0.9238795325112867385, 1.000000000000000000, 0.9238795325112867385, 1.000000000000000000, 0.9238795325112867385, 1.000000000000000000 ) ) 
 REPRESENTATION_ITEM ( '' )  );
#15418=CARTESIAN_POINT ( 'NONE',  ( 69.55000000109247082, 11.46158073645647235, 16.46158073645647235 ) ) ;
#15425=CARTESIAN_POINT ( 'NONE',  ( -68.25000000109245946, 9.999999999999998224, 17.06698730000000097 ) ) ;
#15431=CARTESIAN_POINT ( 'NONE',  ( -69.40000000109249356, 12.06698730000000275, 14.14382582708705094 ) ) ;
#15439=CARTESIAN_POINT ( 'NONE',  ( 67.20000000109247651, 10.85617417291294551, 17.06698729999999742 ) ) ;
#15441=CARTESIAN_POINT ( 'NONE',  ( 69.20000000109246230, 7.933012699999995476, 15.85617417291294196 ) ) ;
#15443=( BOUNDED_CURVE ( )  B_SPLINE_CURVE ( 2, ( #13857, #21112, #15771, #13967, #21229, #4841, #12175, #19445, #14208 ),
 .UNSPECIFIED., .F., .F. ) 
 B_SPLINE_CURVE_WITH_KNOTS ( ( 3, 2, 2, 2, 3 ),
 ( 0.6250000000000005551, 0.6406250000000004441, 0.6562500000000003331, 0.6718750000000002220, 0.6875000000000001110 ),
 .UNSPECIFIED. ) 
 CURVE ( )  GEOMETRIC_REPRESENTATION_ITEM ( )  RATIONAL_B_SPLINE_CURVE ( ( 0.9999999999999973355, 0.9238795325112894030, 1.000000000000000000, 0.9238795325112867385, 1.000000000000000000, 0.9238795325112867385, 1.000000000000000000, 0.9238795325112861834, 1.000000000000000444 ) ) 
 REPRESENTATION_ITEM ( '' )  );
#15464=CARTESIAN_POINT ( 'NONE',  ( -65.75000000109245946, 9.999999999999998224, 17.49999999999999645 ) ) ;
#15465=CARTESIAN_POINT ( 'NONE',  ( 70.95000000218495018, 11.03553390593273598, 17.50000000000000355 ) ) ;
#15468=CARTESIAN_POINT ( 'NONE',  ( 66.85000000109246798, 7.933012699999995476, 14.99999999999999645 ) ) ;
#15473=CARTESIAN_POINT ( 'NONE',  ( 69.75000000109245946, 11.46158073645647235, 16.46158073645647235 ) ) ;
#15484=EDGE_LOOP ( 'NONE', ( #21325, #6360, #13271, #20562, #12340, #22756, #12242, #8534, #5681, #4329, #15341, #337, #2565, #7017, #19460, #16236, #21809, #20772, #1870 ) ) ;
#15485=CARTESIAN_POINT ( 'NONE',  ( -66.15000000109247935, 11.46158073645647235, 13.53841926354352232 ) ) ;
#15487=CARTESIAN_POINT ( 'NONE',  ( -68.15000000109246514, 11.46158073645647235, 16.46158073645647235 ) ) ;
#15496=CARTESIAN_POINT ( 'NONE',  ( -67.75000000109247367, 11.46158073645647235, 13.53841926354352232 ) ) ;
#15499=CARTESIAN_POINT ( 'NONE',  ( -72.09999999999999432, 9.999999999999998224, 12.49999999999999289 ) ) ;
#15508=DIRECTION ( 'NONE',  ( 0.000000000000000000, 0.000000000000000000, 1.000000000000000000 ) ) ;
#15520=DIRECTION ( 'NONE',  ( -1.000000000000000000, -0.000000000000000000, -0.000000000000000000 ) ) ;
#15530=EDGE_CURVE ( 'NONE', #4037, #11622, #5990, .T. ) ;
#15532=CARTESIAN_POINT ( 'NONE',  ( 70.90000000109246514, 10.85617417291294551, 12.93301269999999370 ) ) ;
#15541=CARTESIAN_POINT ( 'NONE',  ( 67.29999999999999716, 9.999999999999998224, 12.49999999999999289 ) ) ;
#15542=CARTESIAN_POINT ( 'NONE',  ( -68.65000000109246514, 9.999999999999998224, 12.93301269999999192 ) ) ;
#15544=CARTESIAN_POINT ( 'NONE',  ( -69.70000000000000284, 9.999999999999998224, 12.49999999999999289 ) ) ;
#15551=EDGE_CURVE ( 'NONE', #19246, #14452, #1057, .T. ) ;
#15561=CARTESIAN_POINT ( 'NONE',  ( 68.65000000109247935, 12.06698730000000097, 14.99999999999999645 ) ) ;
#15562=CARTESIAN_POINT ( 'NONE',  ( 68.20000000109246230, 10.85617417291294551, 17.06698729999999742 ) ) ;
#15589=CARTESIAN_POINT ( 'NONE',  ( 67.70000000109247651, 7.933012699999995476, 14.14382582708705094 ) ) ;
#15593=CARTESIAN_POINT ( 'NONE',  ( 70.25000000109245946, 9.999999999999998224, 12.93301269999999192 ) ) ;
#15598=ORIENTED_EDGE ( 'NONE', *, *, #12762, .F. ) ;
#15605=CARTESIAN_POINT ( 'NONE',  ( -67.20000000109246230, 10.85617417291294551, 17.06698730000000097 ) ) ;
#15608=CARTESIAN_POINT ( 'NONE',  ( -66.45000000109246230, 12.06698730000000097, 14.99999999999999645 ) ) ;
#15613=ORIENTED_EDGE ( 'NONE', *, *, #48, .F. ) ;
#15620=CARTESIAN_POINT ( 'NONE',  ( -70.50000000000000000, 9.999999999999998224, 12.49999999999999289 ) ) ;
#15642=EDGE_CURVE ( 'NONE', #13392, #22910, #11915, .T. ) ;
#15643=CARTESIAN_POINT ( 'NONE',  ( -67.25000000218494733, 7.499999999999995559, 13.96446609406725692 ) ) ;
#15645=AXIS2_PLACEMENT_3D ( 'NONE', #10866, #8952, #18253 ) ;
#15652=CARTESIAN_POINT ( 'NONE',  ( 70.05000000109247082, 9.999999999999998224, 12.93301269999999192 ) ) ;
#15658=CARTESIAN_POINT ( 'NONE',  ( -70.00000000109247367, 7.933012699999995476, 15.85617417291294196 ) ) ;
#15674=CARTESIAN_POINT ( 'NONE',  ( 68.20000000109246230, 7.933012699999995476, 15.85617417291294196 ) ) ;
#15676=CARTESIAN_POINT ( 'NONE',  ( 66.80000000109247082, 7.933012699999995476, 15.85617417291294196 ) ) ;
#15689=( BOUNDED_SURFACE ( )  B_SPLINE_SURFACE ( 1, 2, ( 
 ( #4121, #4359, #876, #641, #2549, #9895, #16834, #4605, #11463, #22674, #16950, #13721, #20518, #17067, #9770, #13493, #18850, #7741, #22562, #7973, #413, #2326, #15410, #20641, #6404, #20985, #8212, #22432, #2437, #22313, #11697, #13256, #18967, #6285, #9659, #4250, #6044, #15291, #19088, #4474, #17190, #6170, #13372, #11941, #2683, #11815, #528, #22793, #19206, #15057, #11583, #10022, #768, #7849, #8100, #5927, #20867, #19553, #3147, #10134, #4717, #21454, #12526, #1342, #17428, #10491, #5183, #17772, #4954, #17885, #23264, #8678, #10614, #12401, #8804, #22915, #1461, #6528, #8455, #15978, #19666, #12161, #6755, #21102, #6874, #5068, #19787, #14068, #12048, #994, #8321, #15643, #14312, #21571, #19314, #15762, #14196, #3269, #16105, #2905, #23144, #23389, #6991, #8562, #13847, #10251, #12288, #6643, #17541, #1109, #23033, #13957, #15870, #21215, #4829, #21334, #19430, #3027, #10377, #17663, #1224, #2048, #7472, #3615, #18008, #5655, #16332, #19907, #3388 ),
 ( #12648, #23626, #12991, #7241, #14431, #14668, #11196, #10954, #12871, #20124, #10731, #21697, #14791, #5782, #18356, #1584, #3731, #22167, #11072, #21927, #18470, #16563, #1938, #3860, #20254, #9389, #16216, #16682, #23503, #1697, #9278, #254, #5424, #32, #5307, #141, #22038, #13110, #7362, #3509, #8923, #7116, #10844, #7589, #14908, #18120, #9041, #14557, #21822, #12760, #20014, #16452, #18232, #1815, #9164, #5538, #13573, #15263, #16926, #6255, #22650, #2168, #2526, #18827, #17283, #18586, #17041, #17160, #22532, #849, #5902, #9866, #19060, #740, #20611, #11312, #20843, #9635, #13226, #20369, #15030, #22765, #9507, #20728, #8183, #6377, #15496, #22284, #8073, #20492, #3976, #384, #4221, #13343, #618, #22408, #16804, #2413, #11558, #7716, #4094, #18942, #503, #9992, #11435, #4451, #18710, #6017, #2299, #6143, #7825, #7944, #15386, #15146, #9745, #13468, #4332, #11788, #2651, #11672, #19401, #19286, #17856, #15948, #1311, #17396, #12374, #1428, #8768 ) ),
 .UNSPECIFIED., .F., .F., .F. ) 
 B_SPLINE_SURFACE_WITH_KNOTS ( ( 2, 2 ),
 ( 3, 2, 2, 2, 2, 2, 2, 2, 2, 2, 2, 2, 2, 2, 2, 2, 2, 2, 2, 2, 2, 2, 2, 2, 2, 2, 2, 2, 2, 2, 2, 2, 2, 2, 2, 2, 2, 2, 2, 2, 2, 2, 2, 2, 2, 2, 2, 2, 2, 2, 2, 2, 2, 2, 2, 2, 2, 2, 2, 2, 2, 2, 2, 2, 3 ),
 ( 0.000000000000000000, 1.000000000000000000 ),
 ( 0.000000000000000000, 0.01562500000000000000, 0.03125000000000000000, 0.04687500000000000000, 0.06250000000000000000, 0.07812500000000000000, 0.09375000000000000000, 0.1093750000000000000, 0.1250000000000000000, 0.1406250000000000000, 0.1562500000000000000, 0.1718750000000000000, 0.1875000000000000000, 0.2031250000000000000, 0.2187500000000000000, 0.2343750000000000000, 0.2500000000000000000, 0.2656250000000000000, 0.2812500000000000000, 0.2968750000000000000, 0.3125000000000000000, 0.3281250000000000000, 0.3437500000000000000, 0.3593750000000000000, 0.3750000000000000000, 0.3906250000000000000, 0.4062500000000000000, 0.4218750000000000000, 0.4375000000000000000, 0.4531250000000000000, 0.4687500000000000000, 0.4843750000000000000, 0.5000000000000000000, 0.5156250000000000000, 0.5312500000000000000, 0.5468750000000000000, 0.5625000000000000000, 0.5781250000000000000, 0.5937500000000000000, 0.6093750000000000000, 0.6250000000000000000, 0.6406250000000000000, 0.6562500000000000000, 0.6718750000000000000, 0.6875000000000000000, 0.7031250000000000000, 0.7187500000000000000, 0.7343750000000000000, 0.7500000000000000000, 0.7656250000000000000, 0.7812500000000000000, 0.7968750000000000000, 0.8125000000000000000, 0.8281250000000000000, 0.8437500000000000000, 0.8593750000000000000, 0.8750000000000000000, 0.8906250000000000000, 0.9062500000000000000, 0.9218750000000000000, 0.9375000000000000000, 0.9531250000000000000, 0.9687500000000000000, 0.9843750000000000000, 1.000000000000000000 ),
 .UNSPECIFIED. ) 
 GEOMETRIC_REPRESENTATION_ITEM ( )  RATIONAL_B_SPLINE_SURFACE ( (
 ( 1.000000000000000000, 0.9238795325112867385, 1.000000000000000000, 0.9238795325112867385, 1.000000000000000000, 0.9238795325112867385, 1.000000000000000000, 0.9238795325112867385, 1.000000000000000000, 0.9238795325112867385, 1.000000000000000000, 0.9238795325112867385, 1.000000000000000000, 0.9238795325112867385, 1.000000000000000000, 0.9238795325112867385, 1.000000000000000000, 0.9238795325112867385, 1.000000000000000000, 0.9238795325112867385, 1.000000000000000000, 0.9238795325112867385, 1.000000000000000000, 0.9238795325112867385, 1.000000000000000000, 0.9238795325112867385, 1.000000000000000000, 0.9238795325112867385, 1.000000000000000000, 0.9238795325112867385, 1.000000000000000000, 0.9238795325112867385, 1.000000000000000000, 0.9238795325112867385, 1.000000000000000000, 0.9238795325112867385, 1.000000000000000000, 0.9238795325112867385, 1.000000000000000000, 0.9238795325112867385, 1.000000000000000000, 0.9238795325112867385, 1.000000000000000000, 0.9238795325112867385, 1.000000000000000000, 0.9238795325112867385, 1.000000000000000000, 0.9238795325112867385, 1.000000000000000000, 0.9238795325112867385, 1.000000000000000000, 0.9238795325112867385, 1.000000000000000000, 0.9238795325112867385, 1.000000000000000000, 0.9238795325112867385, 1.000000000000000000, 0.9238795325112867385, 1.000000000000000000, 0.9238795325112867385, 1.000000000000000000, 0.9238795325112867385, 1.000000000000000000, 0.9238795325112867385, 1.000000000000000000, 0.9238795325112867385, 1.000000000000000000, 0.9238795325112867385, 1.000000000000000000, 0.9238795325112867385, 1.000000000000000000, 0.9238795325112867385, 1.000000000000000000, 0.9238795325112867385, 1.000000000000000000, 0.9238795325112867385, 1.000000000000000000, 0.9238795325112867385, 1.000000000000000000, 0.9238795325112867385, 1.000000000000000000, 0.9238795325112867385, 1.000000000000000000, 0.9238795325112867385, 1.000000000000000000, 0.9238795325112867385, 1.000000000000000000, 0.9238795325112867385, 1.000000000000000000, 0.9238795325112867385, 1.000000000000000000, 0.9238795325112867385, 1.000000000000000000, 0.9238795325112867385, 1.000000000000000000, 0.9238795325112867385, 1.000000000000000000, 0.9238795325112867385, 1.000000000000000000, 0.9238795325112867385, 1.000000000000000000, 0.9238795325112867385, 1.000000000000000000, 0.9238795325112867385, 1.000000000000000000, 0.9238795325112867385, 1.000000000000000000, 0.9238795325112867385, 1.000000000000000000, 0.9238795325112867385, 1.000000000000000000, 0.9238795325112867385, 1.000000000000000000, 0.9238795325112867385, 1.000000000000000000, 0.9238795325112867385, 1.000000000000000000, 0.9238795325112867385, 1.000000000000000000, 0.9238795325112867385, 1.000000000000000000, 0.9238795325112867385, 1.000000000000000000, 0.9238795325112867385, 1.000000000000000000, 0.9238795325112867385, 1.000000000000000000, 0.9238795325112867385, 1.000000000000000000),
 ( 1.000000000000000000, 0.9238795325112867385, 1.000000000000000000, 0.9238795325112867385, 1.000000000000000000, 0.9238795325112867385, 1.000000000000000000, 0.9238795325112867385, 1.000000000000000000, 0.9238795325112867385, 1.000000000000000000, 0.9238795325112867385, 1.000000000000000000, 0.9238795325112867385, 1.000000000000000000, 0.9238795325112867385, 1.000000000000000000, 0.9238795325112867385, 1.000000000000000000, 0.9238795325112867385, 1.000000000000000000, 0.9238795325112867385, 1.000000000000000000, 0.9238795325112867385, 1.000000000000000000, 0.9238795325112867385, 1.000000000000000000, 0.9238795325112867385, 1.000000000000000000, 0.9238795325112867385, 1.000000000000000000, 0.9238795325112867385, 1.000000000000000000, 0.9238795325112867385, 1.000000000000000000, 0.9238795325112867385, 1.000000000000000000, 0.9238795325112867385, 1.000000000000000000, 0.9238795325112867385, 1.000000000000000000, 0.9238795325112867385, 1.000000000000000000, 0.9238795325112867385, 1.000000000000000000, 0.9238795325112867385, 1.000000000000000000, 0.9238795325112867385, 1.000000000000000000, 0.9238795325112867385, 1.000000000000000000, 0.9238795325112867385, 1.000000000000000000, 0.9238795325112867385, 1.000000000000000000, 0.9238795325112867385, 1.000000000000000000, 0.9238795325112867385, 1.000000000000000000, 0.9238795325112867385, 1.000000000000000000, 0.9238795325112867385, 1.000000000000000000, 0.9238795325112867385, 1.000000000000000000, 0.9238795325112867385, 1.000000000000000000, 0.9238795325112867385, 1.000000000000000000, 0.9238795325112867385, 1.000000000000000000, 0.9238795325112867385, 1.000000000000000000, 0.9238795325112867385, 1.000000000000000000, 0.9238795325112867385, 1.000000000000000000, 0.9238795325112867385, 1.000000000000000000, 0.9238795325112867385, 1.000000000000000000, 0.9238795325112867385, 1.000000000000000000, 0.9238795325112867385, 1.000000000000000000, 0.9238795325112867385, 1.000000000000000000, 0.9238795325112867385, 1.000000000000000000, 0.9238795325112867385, 1.000000000000000000, 0.9238795325112867385, 1.000000000000000000, 0.9238795325112867385, 1.000000000000000000, 0.9238795325112867385, 1.000000000000000000, 0.9238795325112867385, 1.000000000000000000, 0.9238795325112867385, 1.000000000000000000, 0.9238795325112867385, 1.000000000000000000, 0.9238795325112867385, 1.000000000000000000, 0.9238795325112867385, 1.000000000000000000, 0.9238795325112867385, 1.000000000000000000, 0.9238795325112867385, 1.000000000000000000, 0.9238795325112867385, 1.000000000000000000, 0.9238795325112867385, 1.000000000000000000, 0.9238795325112867385, 1.000000000000000000, 0.9238795325112867385, 1.000000000000000000, 0.9238795325112867385, 1.000000000000000000, 0.9238795325112867385, 1.000000000000000000, 0.9238795325112867385, 1.000000000000000000, 0.9238795325112867385, 1.000000000000000000, 0.9238795325112867385, 1.000000000000000000) ) ) 
 REPRESENTATION_ITEM ( '' )  SURFACE ( )  );
#15701=CARTESIAN_POINT ( 'NONE',  ( 71.40000000109249356, 7.933012699999995476, 15.85617417291294196 ) ) ;
#15706=CARTESIAN_POINT ( 'NONE',  ( 68.60000000109246798, 9.143825827087052716, 12.93301269999999192 ) ) ;
#15714=CARTESIAN_POINT ( 'NONE',  ( 69.85000000109246798, 9.999999999999998224, 17.06698730000000097 ) ) ;
#15728=CARTESIAN_POINT ( 'NONE',  ( -66.25000000109245946, 9.999999999999998224, 12.93301269999999192 ) ) ;
#15739=CARTESIAN_POINT ( 'NONE',  ( 67.25000000109247367, 9.999999999999998224, 17.06698730000000097 ) ) ;
#15742=CARTESIAN_POINT ( 'NONE',  ( -69.74999999999998579, 11.03553390593273598, 12.49999999999999289 ) ) ;
#15746=CARTESIAN_POINT ( 'NONE',  ( 67.00000000218494733, 9.999999999999998224, 17.49999999999999645 ) ) ;
#15748=LINE ( 'NONE', #17295, #6523 ) ;
#15759=FACE_OUTER_BOUND ( 'NONE', #14084, .T. ) ;
#15762=CARTESIAN_POINT ( 'NONE',  ( -67.05000000218494449, 8.964466094067258695, 17.50000000000000355 ) ) ;
#15764=CARTESIAN_POINT ( 'NONE',  ( -72.15000000109246514, 11.46158073645647235, 16.46158073645647235 ) ) ;
#15768=CARTESIAN_POINT ( 'NONE',  ( 71.10000000109246798, 12.06698730000000275, 15.85617417291294196 ) ) ;
#15771=CARTESIAN_POINT ( 'NONE',  ( 67.70000000218493597, 11.76776695296636888, 16.76776695296636532 ) ) ;
#15773=CARTESIAN_POINT ( 'NONE',  ( -68.45000000109247651, 7.933012699999995476, 14.99999999999999645 ) ) ;
#15779=CARTESIAN_POINT ( 'NONE',  ( 72.50000000000000000, 9.999999999999998224, 14.99999999999999645 ) ) ;
#15788=CARTESIAN_POINT ( 'NONE',  ( 66.70000000109246230, 7.933012699999995476, 14.14382582708705094 ) ) ;
#15789=CARTESIAN_POINT ( 'NONE',  ( 69.15000000109246514, 8.538419263543522320, 16.46158073645647235 ) ) ;
#15791=CARTESIAN_POINT ( 'NONE',  ( -65.55000000218494449, 7.499999999999996447, 16.03553390593273775 ) ) ;
#15799=ORIENTED_EDGE ( 'NONE', *, *, #16575, .T. ) ;
#15802=CARTESIAN_POINT ( 'NONE',  ( 72.37500000054622262, 9.999999999999998224, 17.28349365000000049 ) ) ;
#15803=EDGE_LOOP ( 'NONE', ( #1756, #19142, #11265, #7781 ) ) ;
#15805=CARTESIAN_POINT ( 'NONE',  ( 71.60000000109246798, 9.143825827087050939, 12.93301269999999370 ) ) ;
#15812=CARTESIAN_POINT ( 'NONE',  ( 71.00000000218494733, 9.999999999999998224, 17.49999999999999645 ) ) ;
#15815=CARTESIAN_POINT ( 'NONE',  ( 65.90000000109247935, 9.143825827087049163, 17.06698730000000097 ) ) ;
#15827=LINE ( 'NONE', #8407, #17066 ) ;
#15829=CARTESIAN_POINT ( 'NONE',  ( -72.09999999999999432, 9.999999999999998224, 12.49999999999999289 ) ) ;
#15831=CARTESIAN_POINT ( 'NONE',  ( 72.50000000000000000, 9.999999999999998224, 14.99999999999999645 ) ) ;
#15847=CARTESIAN_POINT ( 'NONE',  ( -68.99999999999998579, 11.76776695296636888, 13.23223304703362579 ) ) ;
#15852=DIRECTION ( 'NONE',  ( 0.000000000000000000, 0.000000000000000000, 1.000000000000000000 ) ) ;
#15854=DIRECTION ( 'NONE',  ( -1.000000000000000000, -0.000000000000000000, -0.000000000000000000 ) ) ;
#15856=CARTESIAN_POINT ( 'NONE',  ( -71.50000000109248788, 7.933012699999995476, 14.14382582708705094 ) ) ;
#15859=CARTESIAN_POINT ( 'NONE',  ( -71.50000000109248788, 7.933012699999995476, 14.14382582708705094 ) ) ;
#15870=CARTESIAN_POINT ( 'NONE',  ( -66.20000000218495018, 9.999999999999998224, 17.49999999999999645 ) ) ;
#15896=CARTESIAN_POINT ( 'NONE',  ( 66.50000000109247367, 9.143825827087049163, 17.06698729999999742 ) ) ;
#15898=CARTESIAN_POINT ( 'NONE',  ( 66.45000000109246230, 12.06698730000000097, 14.99999999999999645 ) ) ;
#15905=DIRECTION ( 'NONE',  ( -1.000000000000000000, -0.000000000000000000, -0.000000000000000000 ) ) ;
#15910=LINE ( 'NONE', #15802, #5063 ) ;
#15919=CARTESIAN_POINT ( 'NONE',  ( 67.55000000218494449, 12.50000000000000000, 13.96446609406725869 ) ) ;
#15924=CARTESIAN_POINT ( 'NONE',  ( 68.80000000109247082, 12.06698729999999919, 14.14382582708705094 ) ) ;
#15929=CARTESIAN_POINT ( 'NONE',  ( 68.05000000109247082, 12.06698730000000097, 14.99999999999999645 ) ) ;
#15931=FACE_OUTER_BOUND ( 'NONE', #17851, .T. ) ;
#15939=CARTESIAN_POINT ( 'NONE',  ( -66.05000000109247082, 7.933012699999995476, 14.99999999999999645 ) ) ;
#15948=CARTESIAN_POINT ( 'NONE',  ( -65.90000000109246514, 7.933012699999995476, 14.14382582708705094 ) ) ;
#15950=CARTESIAN_POINT ( 'NONE',  ( 65.70000000109247651, 9.143825827087049163, 17.06698730000000097 ) ) ;
#15952=CARTESIAN_POINT ( 'NONE',  ( -68.70000000000000284, 7.499999999999996447, 14.99999999999999645 ) ) ;
#15967=CARTESIAN_POINT ( 'NONE',  ( -67.65000000109247935, 9.999999999999998224, 12.93301269999999192 ) ) ;
#15978=CARTESIAN_POINT ( 'NONE',  ( -67.85000000218495586, 8.964466094067258695, 17.50000000000000355 ) ) ;
#15994=CARTESIAN_POINT ( 'NONE',  ( 70.30000000218494449, 8.232233047033627571, 16.76776695296636532 ) ) ;
#15995=EDGE_LOOP ( 'NONE', ( #16100, #11722, #10872, #20507 ) ) ;
#16013=CARTESIAN_POINT ( 'NONE',  ( 66.60000000109248219, 7.933012699999995476, 15.85617417291294196 ) ) ;
#16014=CARTESIAN_POINT ( 'NONE',  ( 66.40000000109247935, 12.06698730000000275, 14.14382582708705094 ) ) ;
#16018=CARTESIAN_POINT ( 'NONE',  ( 69.59999999999999432, 8.232233047033629347, 13.23223304703362402 ) ) ;
#16036=VERTEX_POINT ( 'NONE', #448 ) ;
#16037=CARTESIAN_POINT ( 'NONE',  ( -68.30000000218494449, 11.76776695296636888, 13.23223304703362579 ) ) ;
#16041=CARTESIAN_POINT ( 'NONE',  ( 68.90000000218495302, 8.232233047033629347, 13.23223304703362402 ) ) ;
#16042=DIRECTION ( 'NONE',  ( -1.000000000000000000, -0.000000000000000000, -0.000000000000000000 ) ) ;
#16059=ORIENTED_EDGE ( 'NONE', *, *, #11893, .F. ) ;
#16067=VERTEX_POINT ( 'NONE', #7774 ) ;
#16078=CARTESIAN_POINT ( 'NONE',  ( -71.14999999999999147, 7.499999999999995559, 13.96446609406725692 ) ) ;
#16089=CARTESIAN_POINT ( 'NONE',  ( -70.95000000109247651, 11.46158073645647235, 13.53841926354352232 ) ) ;
#16090=ORIENTED_EDGE ( 'NONE', *, *, #17460, .T. ) ;
#16092=CARTESIAN_POINT ( 'NONE',  ( -67.90000000109246514, 12.06698730000000275, 15.85617417291294196 ) ) ;
#16100=ORIENTED_EDGE ( 'NONE', *, *, #9858, .F. ) ;
#16101=LINE ( 'NONE', #14308, #647 ) ;
#16105=CARTESIAN_POINT ( 'NONE',  ( -66.90000000218495302, 11.76776695296636888, 16.76776695296636532 ) ) ;
#16129=CARTESIAN_POINT ( 'NONE',  ( -72.25000000109247367, 9.999999999999998224, 17.06698730000000097 ) ) ;
#16137=CARTESIAN_POINT ( 'NONE',  ( 66.05000000109247082, 9.999999999999998224, 12.93301269999999192 ) ) ;
#16138=CARTESIAN_POINT ( 'NONE',  ( 70.89999999999999147, 9.999999999999998224, 17.49999999999999645 ) ) ;
#16144=DIRECTION ( 'NONE',  ( 0.000000000000000000, 0.000000000000000000, 1.000000000000000000 ) ) ;
#16145=CARTESIAN_POINT ( 'NONE',  ( -70.55000000218494449, 8.964466094067205404, 12.50000000000004263 ) ) ;
#16154=CARTESIAN_POINT ( 'NONE',  ( 71.00000000218494733, 9.999999999999998224, 17.49999999999999645 ) ) ;
#16156=CARTESIAN_POINT ( 'NONE',  ( 66.00000000218494733, 12.50000000000000000, 14.99999999999999645 ) ) ;
#16160=CARTESIAN_POINT ( 'NONE',  ( 67.90000000218495302, 8.232233047033627571, 16.76776695296636532 ) ) ;
#16169=CARTESIAN_POINT ( 'NONE',  ( 66.85000000109246798, 7.933012699999995476, 14.99999999999999645 ) ) ;
#16170=CARTESIAN_POINT ( 'NONE',  ( -68.99999999999998579, 11.76776695296636888, 13.23223304703362579 ) ) ;
#16178=DIRECTION ( 'NONE',  ( -1.000000000000000000, -0.000000000000000000, -0.000000000000000000 ) ) ;
#16181=ORIENTED_EDGE ( 'NONE', *, *, #15551, .F. ) ;
#16191=CARTESIAN_POINT ( 'NONE',  ( -68.49999999999998579, 9.999999999999998224, 17.49999999999999645 ) ) ;
#16198=CARTESIAN_POINT ( 'NONE',  ( -67.65000000218496723, 12.50000000000000000, 16.03553390593273775 ) ) ;
#16203=CARTESIAN_POINT ( 'NONE',  ( -71.10000000109246798, 12.06698729999999919, 15.85617417291294196 ) ) ;
#16206=CARTESIAN_POINT ( 'NONE',  ( -67.70000000109246230, 10.85617417291294551, 12.93301269999999370 ) ) ;
#16216=CARTESIAN_POINT ( 'NONE',  ( -70.75000000109247367, 8.538419263543524096, 13.53841926354352054 ) ) ;
#16218=CARTESIAN_POINT ( 'NONE',  ( -70.05000000109247082, 7.933012699999995476, 14.99999999999999645 ) ) ;
#16236=ORIENTED_EDGE ( 'NONE', *, *, #20893, .T. ) ;
#16248=CARTESIAN_POINT ( 'NONE',  ( 66.05000000109247082, 7.933012699999995476, 14.99999999999999645 ) ) ;
#16254=AXIS2_PLACEMENT_3D ( 'NONE', #1405, #17726, #23342 ) ;
#16261=CARTESIAN_POINT ( 'NONE',  ( -70.25000000218493312, 8.964466094067294222, 17.50000000000003908 ) ) ;
#16265=LINE ( 'NONE', #2095, #21583 ) ;
#16276=CARTESIAN_POINT ( 'NONE',  ( 69.20000000218495018, 12.50000000000000000, 14.99999999999999645 ) ) ;
#16278=CARTESIAN_POINT ( 'NONE',  ( -68.64999999999999147, 7.499999999999996447, 16.03553390593273775 ) ) ;
#16286=CARTESIAN_POINT ( 'NONE',  ( 68.25000000109245946, 9.999999999999998224, 17.06698730000000097 ) ) ;
#16291=ORIENTED_EDGE ( 'NONE', *, *, #2055, .T. ) ;
#16292=DIRECTION ( 'NONE',  ( 0.000000000000000000, 0.000000000000000000, 1.000000000000000000 ) ) ;
#16296=CARTESIAN_POINT ( 'NONE',  ( -72.34999999999999432, 12.50000000000000000, 16.03553390593273775 ) ) ;
#16301=ORIENTED_EDGE ( 'NONE', *, *, #6277, .T. ) ;
#16302=CARTESIAN_POINT ( 'NONE',  ( 69.79999999999999716, 11.76776695296636888, 13.23223304703362579 ) ) ;
#16312=CARTESIAN_POINT ( 'NONE',  ( -66.19999999999998863, 8.232233047033627571, 16.76776695296636532 ) ) ;
#16314=EDGE_CURVE ( 'NONE', #4004, #4847, #2216, .T. ) ;
#16319=CARTESIAN_POINT ( 'NONE',  ( 68.35000000218495586, 12.50000000000000000, 13.96446609406725692 ) ) ;
#16323=CARTESIAN_POINT ( 'NONE',  ( -68.20000000109246230, 7.933012699999995476, 15.85617417291294196 ) ) ;
#16326=CARTESIAN_POINT ( 'NONE',  ( -67.85000000109248219, 12.06698730000000097, 14.99999999999999645 ) ) ;
#16328=ORIENTED_EDGE ( 'NONE', *, *, #4855, .F. ) ;
#16329=ORIENTED_EDGE ( 'NONE', *, *, #22423, .F. ) ;
#16332=CARTESIAN_POINT ( 'NONE',  ( -65.50000000218494733, 8.232233047033627571, 16.76776695296636532 ) ) ;
#16334=CARTESIAN_POINT ( 'NONE',  ( -69.35000000109246798, 8.538419263543524096, 13.53841926354352054 ) ) ;
#16360=EDGE_CURVE ( 'NONE', #7647, #5505, #6223, .T. ) ;
#16364=CARTESIAN_POINT ( 'NONE',  ( 72.05000000000001137, 8.964466094067258695, 12.49999999999999289 ) ) ;
#16376=FACE_OUTER_BOUND ( 'NONE', #19124, .T. ) ;
#16389=CARTESIAN_POINT ( 'NONE',  ( 69.00000000218494733, 9.999999999999998224, 12.49999999999999289 ) ) ;
#16400=CARTESIAN_POINT ( 'NONE',  ( -69.29999999999999716, 9.999999999999998224, 17.49999999999999645 ) ) ;
#16421=CARTESIAN_POINT ( 'NONE',  ( -66.29999999999999716, 7.499999999999996447, 14.99999999999999645 ) ) ;
#16424=DIRECTION ( 'NONE',  ( -1.000000000000000000, 0.000000000000000000, 0.000000000000000000 ) ) ;
#16425=VECTOR ( 'NONE', #20818, 1000.000000000000000 ) ;
#16426=CARTESIAN_POINT ( 'NONE',  ( -66.99999999999998579, 8.232233047033627571, 16.76776695296636532 ) ) ;
#16437=CARTESIAN_POINT ( 'NONE',  ( -68.95000000109247651, 8.538419263543522320, 16.46158073645647235 ) ) ;
#16440=CARTESIAN_POINT ( 'NONE',  ( -66.05000000109247082, 9.999999999999998224, 12.93301269999999192 ) ) ;
#16442=( BOUNDED_CURVE ( )  B_SPLINE_CURVE ( 2, ( #18468, #6988, #21567, #20252, #3858, #10728, #14428, #16448, #11068 ),
 .UNSPECIFIED., .F., .F. ) 
 B_SPLINE_CURVE_WITH_KNOTS ( ( 3, 2, 2, 2, 3 ),
 ( 0.1875000000000010270, 0.2031250000000009437, 0.2187500000000008327, 0.2343750000000007494, 0.2500000000000006661 ),
 .UNSPECIFIED. ) 
 CURVE ( )  GEOMETRIC_REPRESENTATION_ITEM ( )  RATIONAL_B_SPLINE_CURVE ( ( 0.9999999999999950040, 0.9238795325112917345, 1.000000000000000000, 0.9238795325112867385, 1.000000000000000000, 0.9238795325112867385, 1.000000000000000000, 0.9238795325112835188, 1.000000000000003331 ) ) 
 REPRESENTATION_ITEM ( '' )  );
#16448=CARTESIAN_POINT ( 'NONE',  ( 70.95000000000000284, 8.964466094067294222, 17.50000000000003908 ) ) ;
#16452=CARTESIAN_POINT ( 'NONE',  ( -69.50000000109248788, 12.06698730000000275, 15.85617417291294196 ) ) ;
#16454=CARTESIAN_POINT ( 'NONE',  ( -69.45000000109247651, 9.999999999999998224, 12.93301269999999192 ) ) ;
#16464=CARTESIAN_POINT ( 'NONE',  ( 70.20000000000000284, 8.232233047033627571, 16.76776695296636532 ) ) ;
#16481=CARTESIAN_POINT ( 'NONE',  ( 69.05000000000002558, 12.50000000000000000, 13.96446609406725869 ) ) ;
#16499=DIRECTION ( 'NONE',  ( -1.000000000000000000, -0.000000000000000000, -0.000000000000000000 ) ) ;
#16504=CARTESIAN_POINT ( 'NONE',  ( 70.80000000109248504, 9.143825827087050939, 12.93301269999999370 ) ) ;
#16516=CYLINDRICAL_SURFACE ( 'NONE', #4942, 2.500000000000002220 ) ;
#16523=FILL_AREA_STYLE ('',( #11382 ) ) ;
#16540=CARTESIAN_POINT ( 'NONE',  ( -66.90000000000000568, 9.999999999999998224, 17.49999999999999645 ) ) ;
#16544=CARTESIAN_POINT ( 'NONE',  ( 67.55000000109247082, 8.538419263543524096, 13.53841926354352054 ) ) ;
#16554=CARTESIAN_POINT ( 'NONE',  ( -67.95000000109247651, 11.46158073645647235, 16.46158073645647235 ) ) ;
#16557=CARTESIAN_POINT ( 'NONE',  ( -70.10000000109245377, 7.933012699999995476, 14.14382582708705094 ) ) ;
#16563=CARTESIAN_POINT ( 'NONE',  ( -71.00000000109247367, 12.06698730000000275, 14.14382582708705094 ) ) ;
#16564=CARTESIAN_POINT ( 'NONE',  ( -70.85000000109246798, 7.933012699999995476, 14.99999999999999645 ) ) ;
#16575=EDGE_CURVE ( 'NONE', #18117, #3012, #4679, .T. ) ;
#16588=CARTESIAN_POINT ( 'NONE',  ( 68.95000000000000284, 11.03553390593269157, 12.49999999999994849 ) ) ;
#16595=CARTESIAN_POINT ( 'NONE',  ( 68.45000000000000284, 11.03553390593273598, 17.50000000000000355 ) ) ;
#16602=CARTESIAN_POINT ( 'NONE',  ( -71.84999999999999432, 7.499999999999996447, 16.03553390593273775 ) ) ;
#16612=VECTOR ( 'NONE', #23017, 1000.000000000000000 ) ;
#16619=CARTESIAN_POINT ( 'NONE',  ( 66.30000000218494449, 8.232233047033627571, 16.76776695296636532 ) ) ;
#16622=CARTESIAN_POINT ( 'NONE',  ( 70.80000000109245661, 7.933012699999995476, 15.85617417291294196 ) ) ;
#16628=CARTESIAN_POINT ( 'NONE',  ( 69.80000000218494449, 9.999999999999998224, 12.49999999999999289 ) ) ;
#16629=CARTESIAN_POINT ( 'NONE',  ( 72.45000000000001705, 11.03553390593273953, 17.50000000000000355 ) ) ;
#16639=VECTOR ( 'NONE', #4054, 999.9999999999997726 ) ;
#16645=ADVANCED_FACE ( 'NONE', ( #16713 ), #10144, .T. ) ;
#16650=CARTESIAN_POINT ( 'NONE',  ( 66.60000000218495586, 9.999999999999998224, 12.49999999999999289 ) ) ;
#16651=CARTESIAN_POINT ( 'NONE',  ( 70.00000000109247367, 7.933012699999995476, 15.85617417291294196 ) ) ;
#16655=CARTESIAN_POINT ( 'NONE',  ( -68.59999999999999432, 8.232233047033627571, 16.76776695296636532 ) ) ;
#16658=CARTESIAN_POINT ( 'NONE',  ( 67.45000000109246230, 7.933012699999995476, 14.99999999999999645 ) ) ;
#16665=CARTESIAN_POINT ( 'NONE',  ( -67.10000000218495586, 8.232233047033627571, 16.76776695296636532 ) ) ;
#16668=CARTESIAN_POINT ( 'NONE',  ( -70.05000000109247082, 9.999999999999998224, 12.93301269999999192 ) ) ;
#16671=CARTESIAN_POINT ( 'NONE',  ( -70.20000000109246230, 9.143825827087050939, 12.93301269999999370 ) ) ;
#16675=EDGE_CURVE ( 'NONE', #17274, #14810, #12815, .T. ) ;
#16682=CARTESIAN_POINT ( 'NONE',  ( -70.70000000109247651, 7.933012699999995476, 14.14382582708705094 ) ) ;
#16685=CARTESIAN_POINT ( 'NONE',  ( -70.50000000109245946, 12.06698730000000275, 15.85617417291294196 ) ) ;
#16692=CARTESIAN_POINT ( 'NONE',  ( 68.79999999999999716, 8.232233047033629347, 13.23223304703362402 ) ) ;
#16694=CARTESIAN_POINT ( 'NONE',  ( 70.29999999999999716, 7.499999999999996447, 14.99999999999999645 ) ) ;
#16695=CARTESIAN_POINT ( 'NONE',  ( -70.39999999999999147, 8.232233047033629347, 13.23223304703362402 ) ) ;
#16711=CARTESIAN_POINT ( 'NONE',  ( 69.89999999999999147, 12.50000000000000000, 14.99999999999999645 ) ) ;
#16713=FACE_OUTER_BOUND ( 'NONE', #21508, .T. ) ;
#16718=DIRECTION ( 'NONE',  ( 0.000000000000000000, -0.000000000000000000, -1.000000000000000000 ) ) ;
#16726=VERTEX_POINT ( 'NONE', #19324 ) ;
#16737=CARTESIAN_POINT ( 'NONE',  ( 71.40000000109249356, 7.933012699999995476, 15.85617417291294196 ) ) ;
#16740=CARTESIAN_POINT ( 'NONE',  ( 71.60000000109246798, 7.933012699999995476, 15.85617417291294196 ) ) ;
#16756=DIRECTION ( 'NONE',  ( 0.000000000000000000, 0.000000000000000000, 1.000000000000000000 ) ) ;
#16757=( NAMED_UNIT ( * ) SI_UNIT ( $, .STERADIAN. ) SOLID_ANGLE_UNIT ( ) );
#16760=CARTESIAN_POINT ( 'NONE',  ( 70.75000000000000000, 12.50000000000000000, 16.03553390593273775 ) ) ;
#16775=CARTESIAN_POINT ( 'NONE',  ( 72.20000000109246230, 10.85617417291294551, 17.06698730000000097 ) ) ;
#16777=DIRECTION ( 'NONE',  ( -1.000000000000000000, -0.000000000000000000, -0.000000000000000000 ) ) ;
#16779=CARTESIAN_POINT ( 'NONE',  ( 66.25000000109247367, 12.06698730000000097, 14.99999999999999645 ) ) ;
#16790=CARTESIAN_POINT ( 'NONE',  ( -69.95000000109247651, 8.538419263543524096, 13.53841926354352054 ) ) ;
#16791=ORIENTED_EDGE ( 'NONE', *, *, #4663, .F. ) ;
#16793=CARTESIAN_POINT ( 'NONE',  ( -65.70000000109249072, 9.143825827087049163, 17.06698729999999742 ) ) ;
#16804=CARTESIAN_POINT ( 'NONE',  ( -67.25000000109247367, 9.999999999999998224, 17.06698730000000097 ) ) ;
#16805=CARTESIAN_POINT ( 'NONE',  ( 68.20000000109246230, 7.933012699999995476, 15.85617417291294196 ) ) ;
#16807=CARTESIAN_POINT ( 'NONE',  ( -67.20000000109247651, 12.06698730000000275, 14.14382582708705094 ) ) ;
#16829=ORIENTED_EDGE ( 'NONE', *, *, #6906, .F. ) ;
#16834=CARTESIAN_POINT ( 'NONE',  ( -71.50000000218496155, 11.76776695296636888, 13.23223304703362579 ) ) ;
#16838=CARTESIAN_POINT ( 'NONE',  ( 66.94999999999998863, 8.964466094067258695, 17.50000000000000355 ) ) ;
#16848=CARTESIAN_POINT ( 'NONE',  ( -71.95000000109247651, 11.46158073645647235, 13.53841926354352232 ) ) ;
#16853=CARTESIAN_POINT ( 'NONE',  ( -71.65000000109247935, 9.999999999999998224, 12.93301269999999192 ) ) ;
#16856=ORIENTED_EDGE ( 'NONE', *, *, #4392, .F. ) ;
#16867=CARTESIAN_POINT ( 'NONE',  ( 71.35000000109246798, 8.538419263543522320, 16.46158073645647235 ) ) ;
#16892=DIRECTION ( 'NONE',  ( -1.000000000000000000, -0.000000000000000000, -0.000000000000000000 ) ) ;
#16900=CARTESIAN_POINT ( 'NONE',  ( 70.75000000109247367, 8.538419263543522320, 16.46158073645647235 ) ) ;
#16903=CARTESIAN_POINT ( 'NONE',  ( 72.50000000000000000, 9.999999999999998224, 12.49999999999999289 ) ) ;
#16904=CARTESIAN_POINT ( 'NONE',  ( 71.75000000109247367, 8.538419263543524096, 13.53841926354352054 ) ) ;
#16910=CARTESIAN_POINT ( 'NONE',  ( -71.00000000218494733, 9.999999999999998224, 17.49999999999999645 ) ) ;
#16914=CARTESIAN_POINT ( 'NONE',  ( -65.90000000109247935, 7.933012699999995476, 14.14382582708705094 ) ) ;
#16917=CARTESIAN_POINT ( 'NONE',  ( -71.75000000109247367, 8.538419263543524096, 13.53841926354352054 ) ) ;
#16919=ORIENTED_EDGE ( 'NONE', *, *, #17831, .F. ) ;
#16926=CARTESIAN_POINT ( 'NONE',  ( -69.15000000109247935, 8.538419263543524096, 13.53841926354352054 ) ) ;
#16927=CARTESIAN_POINT ( 'NONE',  ( 67.80000000109247082, 12.06698729999999919, 14.14382582708705094 ) ) ;
#16928=CARTESIAN_POINT ( 'NONE',  ( -68.25000000109245946, 9.999999999999998224, 17.06698730000000097 ) ) ;
#16929=( BOUNDED_CURVE ( )  B_SPLINE_CURVE ( 2, ( #5668, #13000, #16692, #18721, #2423, #20380, #18478, #20265, #3987 ),
 .UNSPECIFIED., .F., .F. ) 
 B_SPLINE_CURVE_WITH_KNOTS ( ( 3, 2, 2, 2, 3 ),
 ( 0.5625000000000008882, 0.5781250000000007772, 0.5937500000000006661, 0.6093750000000006661, 0.6250000000000005551 ),
 .UNSPECIFIED. ) 
 CURVE ( )  GEOMETRIC_REPRESENTATION_ITEM ( )  RATIONAL_B_SPLINE_CURVE ( ( 0.9999999999999956701, 0.9238795325112910684, 1.000000000000000000, 0.9238795325112867385, 1.000000000000000000, 0.9238795325112867385, 1.000000000000000000, 0.9238795325112840739, 1.000000000000002665 ) ) 
 REPRESENTATION_ITEM ( '' )  );
#16950=CARTESIAN_POINT ( 'NONE',  ( -71.30000000218494449, 8.232233047033629347, 13.23223304703362402 ) ) ;
#16953=CARTESIAN_POINT ( 'NONE',  ( 69.25000000000000000, 11.03553390593273598, 17.50000000000000355 ) ) ;
#16960=CARTESIAN_POINT ( 'NONE',  ( -72.04999999999998295, 8.964466094067278235, 12.49999999999997691 ) ) ;
#16961=DIRECTION ( 'NONE',  ( -0.5000000000000013323, -0.000000000000000000, 0.8660254037844380415 ) ) ;
#16965=CYLINDRICAL_SURFACE ( 'NONE', #7942, 2.500000000000002220 ) ;
#16966=CARTESIAN_POINT ( 'NONE',  ( -70.90000000109246514, 10.85617417291294551, 12.93301269999999370 ) ) ;
#16974=AXIS2_PLACEMENT_3D ( 'NONE', #20286, #7276, #172 ) ;
#16978=CARTESIAN_POINT ( 'NONE',  ( 70.00000000109248788, 9.143825827087050939, 12.93301269999999370 ) ) ;
#16981=CARTESIAN_POINT ( 'NONE',  ( 71.65000000109246514, 7.933012699999995476, 14.99999999999999645 ) ) ;
#16989=CARTESIAN_POINT ( 'NONE',  ( 71.40000000218495302, 9.999999999999998224, 12.49999999999999289 ) ) ;
#16990=FACE_OUTER_BOUND ( 'NONE', #4951, .T. ) ;
#17003=ORIENTED_EDGE ( 'NONE', *, *, #22423, .T. ) ;
#17012=CARTESIAN_POINT ( 'NONE',  ( 69.95000000109247651, 8.538419263543522320, 16.46158073645647235 ) ) ;
#17017=CARTESIAN_POINT ( 'NONE',  ( 65.95000000109247651, 8.538419263543524096, 13.53841926354352054 ) ) ;
#17031=CARTESIAN_POINT ( 'NONE',  ( -70.25000000109245946, 9.999999999999998224, 12.93301269999999192 ) ) ;
#17041=CARTESIAN_POINT ( 'NONE',  ( -68.75000000109247367, 11.46158073645647235, 16.46158073645647235 ) ) ;
#17043=CARTESIAN_POINT ( 'NONE',  ( 69.80000000109247082, 7.933012699999995476, 15.85617417291294196 ) ) ;
#17045=CARTESIAN_POINT ( 'NONE',  ( -72.39999999999999147, 11.76776695296636888, 16.76776695296636532 ) ) ;
#17048=DIRECTION ( 'NONE',  ( 1.000000000000000000, 0.000000000000000000, 0.000000000000000000 ) ) ;
#17066=VECTOR ( 'NONE', #17624, 1000.000000000000000 ) ;
#17067=CARTESIAN_POINT ( 'NONE',  ( -71.15000000218493881, 7.499999999999995559, 16.03553390593273420 ) ) ;
#17072=CARTESIAN_POINT ( 'NONE',  ( -71.24999999999998579, 8.964466094067205404, 12.50000000000004263 ) ) ;
#17073=CARTESIAN_POINT ( 'NONE',  ( 69.50000000109248788, 12.06698730000000275, 15.85617417291294196 ) ) ;
#17079=CARTESIAN_POINT ( 'NONE',  ( -70.75000000109247367, 8.538419263543522320, 16.46158073645647235 ) ) ;
#17085=CARTESIAN_POINT ( 'NONE',  ( -71.95000000109247651, 11.46158073645647235, 16.46158073645647235 ) ) ;
#17086=ORIENTED_EDGE ( 'NONE', *, *, #20831, .T. ) ;
#17090=CARTESIAN_POINT ( 'NONE',  ( 69.70000000000000284, 9.999999999999998224, 12.49999999999999289 ) ) ;
#17093=CARTESIAN_POINT ( 'NONE',  ( 69.75000000109247367, 8.538419263543522320, 16.46158073645647235 ) ) ;
#17094=CARTESIAN_POINT ( 'NONE',  ( 71.35000000109246798, 11.46158073645647235, 16.46158073645647235 ) ) ;
#17096=( BOUNDED_CURVE ( )  B_SPLINE_CURVE ( 2, ( #10542, #3086, #3196, #4882, #6685, #19488, #8726, #17819, #23190 ),
 .UNSPECIFIED., .F., .F. ) 
 B_SPLINE_CURVE_WITH_KNOTS ( ( 3, 2, 2, 2, 3 ),
 ( 0.7499999999999997780, 0.7656249999999996669, 0.7812499999999995559, 0.7968749999999994449, 0.8124999999999993339 ),
 .UNSPECIFIED. ) 
 CURVE ( )  GEOMETRIC_REPRESENTATION_ITEM ( )  RATIONAL_B_SPLINE_CURVE ( ( 1.000000000000001110, 0.9238795325112856283, 1.000000000000000000, 0.9238795325112867385, 1.000000000000000000, 0.9238795325112867385, 1.000000000000000000, 0.9238795325112899581, 0.9999999999999967804 ) ) 
 REPRESENTATION_ITEM ( '' )  );
#17100=CARTESIAN_POINT ( 'NONE',  ( 66.70000000218495018, 11.76776695296636888, 13.23223304703362579 ) ) ;
#17104=CARTESIAN_POINT ( 'NONE',  ( -66.40000000109247935, 12.06698729999999919, 14.14382582708705094 ) ) ;
#17105=ORIENTED_EDGE ( 'NONE', *, *, #22673, .F. ) ;
#17113=ORIENTED_EDGE ( 'NONE', *, *, #8478, .T. ) ;
#17122=CARTESIAN_POINT ( 'NONE',  ( 71.55000000109247082, 8.538419263543524096, 13.53841926354352054 ) ) ;
#17124=CARTESIAN_POINT ( 'NONE',  ( 71.50000000218496155, 11.76776695296636888, 13.23223304703362579 ) ) ;
#17128=CARTESIAN_POINT ( 'NONE',  ( 72.15000000109246514, 11.46158073645647235, 16.46158073645647235 ) ) ;
#17135=CARTESIAN_POINT ( 'NONE',  ( 71.30000000109247082, 12.06698730000000275, 15.85617417291294196 ) ) ;
#17147=CARTESIAN_POINT ( 'NONE',  ( -65.85000000109248219, 7.933012699999995476, 14.99999999999999645 ) ) ;
#17150=CARTESIAN_POINT ( 'NONE',  ( -67.90000000109245093, 10.85617417291294551, 12.93301269999999370 ) ) ;
#17160=CARTESIAN_POINT ( 'NONE',  ( -68.70000000109246230, 12.06698730000000275, 15.85617417291294196 ) ) ;
#17161=CARTESIAN_POINT ( 'NONE',  ( 70.35000000109248219, 11.46158073645647235, 16.46158073645647235 ) ) ;
#17163=CARTESIAN_POINT ( 'NONE',  ( -66.75000000109245946, 8.538419263543522320, 16.46158073645647235 ) ) ;
#17179=CIRCLE ( 'NONE', #3016, 2.500000000000002220 ) ;
#17190=CARTESIAN_POINT ( 'NONE',  ( -69.80000000218494449, 9.999999999999998224, 12.49999999999999289 ) ) ;
#17194=CARTESIAN_POINT ( 'NONE',  ( 66.44999999999998863, 8.964466094067258695, 12.49999999999999289 ) ) ;
#17197=CARTESIAN_POINT ( 'NONE',  ( 70.30000000109248504, 12.06698730000000275, 15.85617417291294196 ) ) ;
#17205=CARTESIAN_POINT ( 'NONE',  ( -70.05000000218494449, 12.50000000000000000, 16.03553390593273775 ) ) ;
#17209=( NAMED_UNIT ( * ) PLANE_ANGLE_UNIT ( ) SI_UNIT ( $, .RADIAN. ) );
#17212=CARTESIAN_POINT ( 'NONE',  ( -69.50000000109248788, 12.06698730000000275, 15.85617417291294196 ) ) ;
#17222=CARTESIAN_POINT ( 'NONE',  ( 68.80000000109247082, 10.85617417291294551, 17.06698729999999742 ) ) ;
#17226=CARTESIAN_POINT ( 'NONE',  ( 68.80000000109247082, 12.06698730000000275, 14.14382582708705094 ) ) ;
#17230=CARTESIAN_POINT ( 'NONE',  ( 71.80000000218494449, 9.999999999999998224, 17.49999999999999645 ) ) ;
#17238=CARTESIAN_POINT ( 'NONE',  ( -70.70000000000000284, 12.50000000000000000, 14.99999999999999645 ) ) ;
#17245=VERTEX_POINT ( 'NONE', #4903 ) ;
#17248=CARTESIAN_POINT ( 'NONE',  ( 70.75000000109247367, 8.538419263543524096, 13.53841926354352054 ) ) ;
#17255=CARTESIAN_POINT ( 'NONE',  ( 67.00000000109245946, 9.143825827087052716, 12.93301269999999192 ) ) ;
#17261=CARTESIAN_POINT ( 'NONE',  ( 70.95000000109247651, 8.538419263543524096, 13.53841926354352054 ) ) ;
#17271=CARTESIAN_POINT ( 'NONE',  ( -66.65000000109247935, 7.933012699999995476, 14.99999999999999645 ) ) ;
#17273=CARTESIAN_POINT ( 'NONE',  ( -67.15000000109247935, 11.46158073645647235, 13.53841926354352232 ) ) ;
#17274=VERTEX_POINT ( 'NONE', #6477 ) ;
#17278=ADVANCED_FACE ( 'NONE', ( #2855 ), #3215, .T. ) ;
#17283=CARTESIAN_POINT ( 'NONE',  ( -68.85000000109248219, 9.999999999999998224, 17.06698730000000097 ) ) ;
#17285=CARTESIAN_POINT ( 'NONE',  ( 69.60000000109248219, 10.85617417291294551, 17.06698730000000097 ) ) ;
#17286=CARTESIAN_POINT ( 'NONE',  ( -67.60000000109246798, 7.933012699999995476, 15.85617417291294196 ) ) ;
#17293=CARTESIAN_POINT ( 'NONE',  ( 71.29999999999998295, 9.999999999999998224, 12.49999999999999289 ) ) ;
#17295=CARTESIAN_POINT ( 'NONE',  ( 72.50000000000000000, 9.999999999999998224, 17.49999999999999645 ) ) ;
#17306=DIRECTION ( 'NONE',  ( 1.000000000000000000, 0.000000000000000000, 0.000000000000000000 ) ) ;
#17309=FACE_OUTER_BOUND ( 'NONE', #15484, .T. ) ;
#17313=ADVANCED_FACE ( 'NONE', ( #15931 ), #10205, .T. ) ;
#17316=CARTESIAN_POINT ( 'NONE',  ( 69.80000000109247082, 7.933012699999995476, 15.85617417291294196 ) ) ;
#17324=CARTESIAN_POINT ( 'NONE',  ( -69.45000000109247651, 9.999999999999998224, 12.93301269999999192 ) ) ;
#17338=CARTESIAN_POINT ( 'NONE',  ( 68.45000000109247651, 9.999999999999998224, 12.93301269999999192 ) ) ;
#17339=CARTESIAN_POINT ( 'NONE',  ( 68.90000000109246514, 12.06698730000000275, 15.85617417291294196 ) ) ;
#17347=CARTESIAN_POINT ( 'NONE',  ( 67.85000000218494165, 8.964466094067287116, 17.50000000000002487 ) ) ;
#17364=CARTESIAN_POINT ( 'NONE',  ( 71.20000000218495018, 7.499999999999996447, 14.99999999999999645 ) ) ;
#17367=CARTESIAN_POINT ( 'NONE',  ( 69.05000000109247082, 9.999999999999998224, 17.06698730000000097 ) ) ;
#17371=CARTESIAN_POINT ( 'NONE',  ( 70.85000000109246798, 7.933012699999995476, 14.99999999999999645 ) ) ;
#17386=CARTESIAN_POINT ( 'NONE',  ( -66.55000000109247082, 11.46158073645647235, 16.46158073645647235 ) ) ;
#17396=CARTESIAN_POINT ( 'NONE',  ( -65.80000000109247082, 7.933012699999995476, 15.85617417291294196 ) ) ;
#17398=CARTESIAN_POINT ( 'NONE',  ( 66.65000000109247935, 7.933012699999995476, 14.99999999999999645 ) ) ;
#17400=CARTESIAN_POINT ( 'NONE',  ( -71.34999999999999432, 11.03553390593273598, 12.49999999999999289 ) ) ;
#17402=CARTESIAN_POINT ( 'NONE',  ( -71.59999999999999432, 11.76776695296636888, 16.76776695296636532 ) ) ;
#17416=EDGE_CURVE ( 'NONE', #20854, #11744, #541, .T. ) ;
#17427=EDGE_CURVE ( 'NONE', #7757, #23046, #3462, .T. ) ;
#17428=CARTESIAN_POINT ( 'NONE',  ( -68.60000000218495586, 9.999999999999998224, 17.49999999999999645 ) ) ;
#17430=CARTESIAN_POINT ( 'NONE',  ( -71.29999999999998295, 9.999999999999998224, 12.49999999999999289 ) ) ;
#17433=CARTESIAN_POINT ( 'NONE',  ( -72.09999999999999432, 9.999999999999998224, 12.49999999999999289 ) ) ;
#17434=CARTESIAN_POINT ( 'NONE',  ( 70.55000000109247082, 8.538419263543522320, 16.46158073645647235 ) ) ;
#17436=DIRECTION ( 'NONE',  ( 0.000000000000000000, 0.000000000000000000, 1.000000000000000000 ) ) ;
#17438=EDGE_CURVE ( 'NONE', #23070, #14683, #4537, .T. ) ;
#17443=CARTESIAN_POINT ( 'NONE',  ( -69.15000000109246514, 8.538419263543522320, 16.46158073645647235 ) ) ;
#17456=CARTESIAN_POINT ( 'NONE',  ( -66.49999999999998579, 9.999999999999998224, 12.49999999999999289 ) ) ;
#17460=EDGE_CURVE ( 'NONE', #20225, #19081, #20108, .T. ) ;
#17461=CARTESIAN_POINT ( 'NONE',  ( 67.25000000109247367, 9.999999999999998224, 17.06698730000000097 ) ) ;
#17462=CARTESIAN_POINT ( 'NONE',  ( 67.90000000109245093, 10.85617417291294551, 12.93301269999999370 ) ) ;
#17470=EDGE_LOOP ( 'NONE', ( #10362, #13621, #21647 ) ) ;
#17471=CARTESIAN_POINT ( 'NONE',  ( -67.40000000218495302, 9.999999999999998224, 12.49999999999999289 ) ) ;
#17482=EDGE_CURVE ( 'NONE', #20225, #14363, #5539, .T. ) ;
#17483=CARTESIAN_POINT ( 'NONE',  ( 71.50000000109248788, 7.933012699999995476, 14.14382582708705094 ) ) ;
#17484=CARTESIAN_POINT ( 'NONE',  ( 69.90000000218495302, 11.76776695296636888, 13.23223304703362579 ) ) ;
#17487=CARTESIAN_POINT ( 'NONE',  ( 67.40000000109247935, 10.85617417291294551, 17.06698730000000097 ) ) ;
#17491=CARTESIAN_POINT ( 'NONE',  ( 68.35000000109246798, 8.538419263543522320, 16.46158073645647235 ) ) ;
#17504=CARTESIAN_POINT ( 'NONE',  ( -69.00000000109245946, 10.85617417291294551, 17.06698729999999742 ) ) ;
#17507=LINE ( 'NONE', #2642, #4801 ) ;
#17517=CARTESIAN_POINT ( 'NONE',  ( -70.79999999999999716, 11.76776695296636888, 16.76776695296636532 ) ) ;
#17518=CARTESIAN_POINT ( 'NONE',  ( -71.29999999999998295, 9.999999999999998224, 12.49999999999999289 ) ) ;
#17521=VECTOR ( 'NONE', #7305, 1000.000000000000000 ) ;
#17526=CARTESIAN_POINT ( 'NONE',  ( -68.60000000218495586, 9.999999999999998224, 17.49999999999999645 ) ) ;
#17535=FACE_OUTER_BOUND ( 'NONE', #5952, .T. ) ;
#17538=ORIENTED_EDGE ( 'NONE', *, *, #8863, .F. ) ;
#17541=CARTESIAN_POINT ( 'NONE',  ( -66.40000000218495302, 7.499999999999996447, 14.99999999999999645 ) ) ;
#17552=CARTESIAN_POINT ( 'NONE',  ( 68.75000000109247367, 11.46158073645647235, 16.46158073645647235 ) ) ;
#17558=CARTESIAN_POINT ( 'NONE',  ( -69.90000000109246514, 9.143825827087049163, 17.06698730000000097 ) ) ;
#17569=VECTOR ( 'NONE', #5361, 1000.000000000000000 ) ;
#17571=ORIENTED_EDGE ( 'NONE', *, *, #15642, .F. ) ;
#17574=CARTESIAN_POINT ( 'NONE',  ( 69.35000000109248219, 11.46158073645647235, 13.53841926354352232 ) ) ;
#17576=CARTESIAN_POINT ( 'NONE',  ( 66.60000000109246798, 10.85617417291294551, 17.06698729999999742 ) ) ;
#17600=CARTESIAN_POINT ( 'NONE',  ( 66.05000000218494449, 12.50000000000000000, 16.03553390593273775 ) ) ;
#17604=CARTESIAN_POINT ( 'NONE',  ( 69.85000000218495586, 11.03553390593273598, 12.49999999999999289 ) ) ;
#17607=CARTESIAN_POINT ( 'NONE',  ( 66.05000000109247082, 7.933012699999995476, 14.99999999999999645 ) ) ;
#17614=CARTESIAN_POINT ( 'NONE',  ( 69.45000000109247651, 9.999999999999998224, 12.93301269999999192 ) ) ;
#17624=DIRECTION ( 'NONE',  ( 1.000000000000000000, -0.000000000000000000, -0.000000000000000000 ) ) ;
#17640=CARTESIAN_POINT ( 'NONE',  ( 66.10000000109248219, 10.85617417291294551, 12.93301269999999192 ) ) ;
#17641=CARTESIAN_POINT ( 'NONE',  ( -69.09999999999999432, 12.50000000000000000, 14.99999999999999645 ) ) ;
#17655=CARTESIAN_POINT ( 'NONE',  ( -70.55000000109247082, 8.538419263543522320, 16.46158073645647235 ) ) ;
#17656=CARTESIAN_POINT ( 'NONE',  ( 72.50000000000000000, 9.999999999999998224, 14.99999999999999645 ) ) ;
#17659=ORIENTED_EDGE ( 'NONE', *, *, #22166, .T. ) ;
#17663=CARTESIAN_POINT ( 'NONE',  ( -65.85000000218495586, 11.03553390593273598, 12.49999999999999289 ) ) ;
#17669=CARTESIAN_POINT ( 'NONE',  ( 67.09999999999999432, 7.499999999999996447, 14.99999999999999645 ) ) ;
#17673=CARTESIAN_POINT ( 'NONE',  ( -69.50000000109245946, 10.85617417291294551, 12.93301269999999192 ) ) ;
#17678=DIRECTION ( 'NONE',  ( -1.000000000000000000, -0.000000000000000000, -0.000000000000000000 ) ) ;
#17688=CARTESIAN_POINT ( 'NONE',  ( -69.55000000218493028, 7.499999999999996447, 16.03553390593273775 ) ) ;
#17691=CARTESIAN_POINT ( 'NONE',  ( 72.35000000000000853, 12.50000000000000000, 16.03553390593273420 ) ) ;
#17695=( BOUNDED_CURVE ( )  B_SPLINE_CURVE ( 2, ( #3474, #6608, #4794, #1417, #23471, #19871, #18085, #3117, #19750 ),
 .UNSPECIFIED., .F., .F. ) 
 B_SPLINE_CURVE_WITH_KNOTS ( ( 3, 2, 2, 2, 3 ),
 ( 0.8749999999999990008, 0.8906249999999994449, 0.9062499999999998890, 0.9218750000000003331, 0.9375000000000007772 ),
 .UNSPECIFIED. ) 
 CURVE ( )  GEOMETRIC_REPRESENTATION_ITEM ( )  RATIONAL_B_SPLINE_CURVE ( ( 1.000000000000004885, 0.9238795325112818535, 1.000000000000000000, 0.9238795325112867385, 1.000000000000000000, 0.9238795325112867385, 1.000000000000000000, 0.9238795325112829637, 1.000000000000003775 ) ) 
 REPRESENTATION_ITEM ( '' )  );
#17712=CARTESIAN_POINT ( 'NONE',  ( -68.50000000218494733, 11.76776695296636888, 16.76776695296636532 ) ) ;
#17716=CARTESIAN_POINT ( 'NONE',  ( 68.65000000218496723, 8.964466094067258695, 17.50000000000000355 ) ) ;
#17720=CARTESIAN_POINT ( 'NONE',  ( 68.25000000109245946, 9.999999999999998224, 17.06698730000000097 ) ) ;
#17724=CARTESIAN_POINT ( 'NONE',  ( 67.30000000109247082, 12.06698730000000275, 15.85617417291294196 ) ) ;
#17726=DIRECTION ( 'NONE',  ( -1.000000000000000000, -0.000000000000000000, -0.000000000000000000 ) ) ;
#17732=CARTESIAN_POINT ( 'NONE',  ( 66.84999999999999432, 11.03553390593268624, 17.50000000000005329 ) ) ;
#17736=ADVANCED_FACE ( 'NONE', ( #3076 ), #11854, .T. ) ;
#17749=CARTESIAN_POINT ( 'NONE',  ( -69.49999999999998579, 7.499999999999996447, 14.99999999999999645 ) ) ;
#17753=CARTESIAN_POINT ( 'NONE',  ( -67.40000000218495302, 9.999999999999998224, 12.49999999999999289 ) ) ;
#17754=CARTESIAN_POINT ( 'NONE',  ( -66.09999999999999432, 9.999999999999998224, 17.49999999999999645 ) ) ;
#17761=CARTESIAN_POINT ( 'NONE',  ( -67.80000000109247082, 12.06698730000000275, 14.14382582708705094 ) ) ;
#17767=DIRECTION ( 'NONE',  ( -1.000000000000000000, -0.000000000000000000, -0.000000000000000000 ) ) ;
#17772=CARTESIAN_POINT ( 'NONE',  ( -68.45000000218493597, 12.50000000000000000, 16.03553390593273420 ) ) ;
#17774=CARTESIAN_POINT ( 'NONE',  ( -72.20000000109246230, 10.85617417291294551, 17.06698729999999742 ) ) ;
#17796=CARTESIAN_POINT ( 'NONE',  ( 70.89999999999999147, 9.999999999999998224, 17.49999999999999645 ) ) ;
#17800=CARTESIAN_POINT ( 'NONE',  ( 66.10000000109248219, 10.85617417291294551, 12.93301269999999370 ) ) ;
#17801=CARTESIAN_POINT ( 'NONE',  ( 71.79999999999998295, 8.232233047033627571, 16.76776695296636532 ) ) ;
#17810=CARTESIAN_POINT ( 'NONE',  ( 68.15000000218495302, 8.964466094067214286, 12.50000000000004086 ) ) ;
#17819=CARTESIAN_POINT ( 'NONE',  ( -67.35000000000000853, 11.03553390593276973, 12.50000000000002665 ) ) ;
#17820=AXIS2_PLACEMENT_3D ( 'NONE', #17656, #6748, #10722 ) ;
#17822=ORIENTED_EDGE ( 'NONE', *, *, #7446, .T. ) ;
#17826=CARTESIAN_POINT ( 'NONE',  ( 67.60000000218495586, 12.50000000000000000, 14.99999999999999645 ) ) ;
#17831=EDGE_CURVE ( 'NONE', #16726, #3210, #10378, .T. ) ;
#17835=CARTESIAN_POINT ( 'NONE',  ( 67.25000000109245946, 12.06698730000000097, 14.99999999999999645 ) ) ;
#17842=CARTESIAN_POINT ( 'NONE',  ( 66.90000000000000568, 9.999999999999998224, 17.49999999999999645 ) ) ;
#17843=DIRECTION ( 'NONE',  ( 1.000000000000000000, 0.000000000000000000, 0.000000000000000000 ) ) ;
#17846=CYLINDRICAL_SURFACE ( 'NONE', #2082, 2.500000000000002220 ) ;
#17851=EDGE_LOOP ( 'NONE', ( #13680, #19872, #10505, #2185 ) ) ;
#17856=CARTESIAN_POINT ( 'NONE',  ( -65.95000000109247651, 8.538419263543524096, 13.53841926354352054 ) ) ;
#17857=ADVANCED_FACE ( 'NONE', ( #4871 ), #10177, .T. ) ;
#17858=CARTESIAN_POINT ( 'NONE',  ( 65.95000000109247651, 8.538419263543524096, 13.53841926354352054 ) ) ;
#17860=CARTESIAN_POINT ( 'NONE',  ( -71.50000000000000000, 12.50000000000000000, 14.99999999999999645 ) ) ;
#17867=CARTESIAN_POINT ( 'NONE',  ( 68.30000000218494449, 11.76776695296636888, 13.23223304703362579 ) ) ;
#17871=ADVANCED_FACE ( 'NONE', ( #9079 ), #1854, .T. ) ;
#17877=CARTESIAN_POINT ( 'NONE',  ( -67.30000000109247082, 9.143825827087049163, 17.06698729999999742 ) ) ;
#17882=CYLINDRICAL_SURFACE ( 'NONE', #22821, 2.500000000000002220 ) ;
#17885=CARTESIAN_POINT ( 'NONE',  ( -68.35000000218495586, 12.50000000000000000, 13.96446609406725869 ) ) ;
#17918=CARTESIAN_POINT ( 'NONE',  ( 66.00000000109245946, 7.933012699999995476, 15.85617417291294196 ) ) ;
#17919=CARTESIAN_POINT ( 'NONE',  ( -65.50000000218494733, 8.232233047033627571, 16.76776695296636532 ) ) ;
#17927=CARTESIAN_POINT ( 'NONE',  ( -68.49999999999998579, 9.999999999999998224, 17.49999999999999645 ) ) ;
#17933=ORIENTED_EDGE ( 'NONE', *, *, #17831, .T. ) ;
#17937=CARTESIAN_POINT ( 'NONE',  ( 71.15000000218496723, 7.499999999999996447, 16.03553390593273775 ) ) ;
#17939=ORIENTED_EDGE ( 'NONE', *, *, #1266, .T. ) ;
#17943=CARTESIAN_POINT ( 'NONE',  ( 67.30000000218494449, 8.232233047033629347, 13.23223304703362402 ) ) ;
#17953=CARTESIAN_POINT ( 'NONE',  ( 67.10000000109246798, 10.85617417291294551, 12.93301269999999370 ) ) ;
#17959=CARTESIAN_POINT ( 'NONE',  ( 68.49999999999998579, 9.999999999999998224, 17.49999999999999645 ) ) ;
#17967=ORIENTED_EDGE ( 'NONE', *, *, #7862, .F. ) ;
#17982=CARTESIAN_POINT ( 'NONE',  ( -67.34999999999999432, 11.03553390593273598, 12.49999999999999289 ) ) ;
#17984=CARTESIAN_POINT ( 'NONE',  ( 66.55000000218494449, 8.964466094067294222, 12.49999999999996092 ) ) ;
#17986=CARTESIAN_POINT ( 'NONE',  ( 70.90000000218495302, 11.76776695296636888, 16.76776695296636532 ) ) ;
#17989=CARTESIAN_POINT ( 'NONE',  ( 68.05000000000001137, 8.964466094067256918, 12.49999999999999822 ) ) ;
#17991=CARTESIAN_POINT ( 'NONE',  ( -66.30000000218494449, 8.232233047033627571, 16.76776695296636532 ) ) ;
#17993=CARTESIAN_POINT ( 'NONE',  ( -71.70000000109247651, 10.85617417291294551, 12.93301269999999192 ) ) ;
#17996=CARTESIAN_POINT ( 'NONE',  ( -67.25000000109247367, 9.999999999999998224, 17.06698730000000097 ) ) ;
#18008=CARTESIAN_POINT ( 'NONE',  ( -65.60000000218495586, 7.499999999999996447, 14.99999999999999645 ) ) ;
#18014=CYLINDRICAL_SURFACE ( 'NONE', #12217, 2.500000000000002220 ) ;
#18016=CARTESIAN_POINT ( 'NONE',  ( 67.24999999999998579, 8.964466094067294222, 12.49999999999996092 ) ) ;
#18020=CARTESIAN_POINT ( 'NONE',  ( 70.60000000218494165, 9.999999999999998224, 12.49999999999999289 ) ) ;
#18022=CARTESIAN_POINT ( 'NONE',  ( 70.50000000000000000, 9.999999999999998224, 12.49999999999999289 ) ) ;
#18032=ADVANCED_FACE ( 'NONE', ( #1741 ), #5462, .F. ) ;
#18033=CARTESIAN_POINT ( 'NONE',  ( 69.25000000000000000, 11.03553390593269157, 17.50000000000004619 ) ) ;
#18040=EDGE_CURVE ( 'NONE', #4247, #19246, #22079, .T. ) ;
#18041=CARTESIAN_POINT ( 'NONE',  ( 70.59999999999999432, 11.76776695296636888, 13.23223304703362579 ) ) ;
#18043=CARTESIAN_POINT ( 'NONE',  ( 69.65000000218496723, 7.499999999999996447, 13.96446609406725514 ) ) ;
#18060=ORIENTED_EDGE ( 'NONE', *, *, #10135, .T. ) ;
#18063=CARTESIAN_POINT ( 'NONE',  ( 66.75000000218494733, 12.50000000000000000, 13.96446609406725869 ) ) ;
#18065=CARTESIAN_POINT ( 'NONE',  ( 66.49999999999998579, 9.999999999999998224, 12.49999999999999289 ) ) ;
#18073=CARTESIAN_POINT ( 'NONE',  ( -69.20000000000000284, 11.76776695296636888, 16.76776695296636532 ) ) ;
#18085=CARTESIAN_POINT ( 'NONE',  ( -65.90000000218495302, 11.76776695296636888, 13.23223304703362579 ) ) ;
#18089=CARTESIAN_POINT ( 'NONE',  ( -66.40000000000000568, 8.232233047033629347, 13.23223304703362402 ) ) ;
#18092=CARTESIAN_POINT ( 'NONE',  ( 72.15000000109247935, 9.999999999999998224, 17.49999999999999645 ) ) ;
#18094=CARTESIAN_POINT ( 'NONE',  ( -66.64999999999999147, 12.50000000000000000, 13.96446609406725869 ) ) ;
#18095=VECTOR ( 'NONE', #23277, 1000.000000000000000 ) ;
#18106=CARTESIAN_POINT ( 'NONE',  ( -68.85000000109248219, 9.999999999999998224, 17.06698730000000097 ) ) ;
#18109=CARTESIAN_POINT ( 'NONE',  ( -67.35000000109248219, 8.538419263543522320, 16.46158073645647235 ) ) ;
#18113=FACE_OUTER_BOUND ( 'NONE', #20667, .T. ) ;
#18117=VERTEX_POINT ( 'NONE', #18754 ) ;
#18120=CARTESIAN_POINT ( 'NONE',  ( -69.80000000109247082, 7.933012699999995476, 15.85617417291294196 ) ) ;
#18121=CARTESIAN_POINT ( 'NONE',  ( -68.45000000109247651, 7.933012699999995476, 14.99999999999999645 ) ) ;
#18126=EDGE_CURVE ( 'NONE', #7757, #8256, #22584, .T. ) ;
#18138=CARTESIAN_POINT ( 'NONE',  ( 72.50000000000000000, 9.999999999999998224, 12.49999999999999289 ) ) ;
#18148=CARTESIAN_POINT ( 'NONE',  ( 70.79999999999999716, 11.76776695296636888, 16.76776695296636532 ) ) ;
#18151=VECTOR ( 'NONE', #5552, 1000.000000000000000 ) ;
#18177=CARTESIAN_POINT ( 'NONE',  ( 68.80000000218494449, 7.499999999999996447, 14.99999999999999645 ) ) ;
#18179=CARTESIAN_POINT ( 'NONE',  ( 66.90000000000000568, 9.999999999999998224, 17.49999999999999645 ) ) ;
#18188=CARTESIAN_POINT ( 'NONE',  ( -68.95000000000000284, 11.03553390593269157, 12.49999999999994849 ) ) ;
#18212=CARTESIAN_POINT ( 'NONE',  ( -67.14999999999999147, 7.499999999999995559, 13.96446609406725692 ) ) ;
#18221=CARTESIAN_POINT ( 'NONE',  ( -70.45000000109247651, 9.999999999999998224, 17.06698730000000097 ) ) ;
#18224=CARTESIAN_POINT ( 'NONE',  ( -66.85000000109248219, 9.999999999999998224, 12.93301269999999192 ) ) ;
#18232=CARTESIAN_POINT ( 'NONE',  ( -69.45000000109247651, 12.06698730000000097, 14.99999999999999645 ) ) ;
#18234=CARTESIAN_POINT ( 'NONE',  ( -68.40000000109246514, 7.933012699999995476, 15.85617417291294196 ) ) ;
#18240=CARTESIAN_POINT ( 'NONE',  ( -68.09999999999999432, 9.999999999999998224, 12.49999999999999289 ) ) ;
#18242=ORIENTED_EDGE ( 'NONE', *, *, #4398, .T. ) ;
#18243=CARTESIAN_POINT ( 'NONE',  ( 70.20000000218495018, 9.999999999999998224, 17.49999999999999645 ) ) ;
#18249=CARTESIAN_POINT ( 'NONE',  ( -72.15000000109247935, 9.999999999999998224, 17.49999999999999645 ) ) ;
#18253=DIRECTION ( 'NONE',  ( 0.000000000000000000, 0.000000000000000000, 1.000000000000000000 ) ) ;
#18262=CARTESIAN_POINT ( 'NONE',  ( 69.74999999999998579, 11.03553390593273598, 12.49999999999999289 ) ) ;
#18275=DIRECTION ( 'NONE',  ( 0.000000000000000000, -1.000000000000000000, -0.000000000000000000 ) ) ;
#18287=ORIENTED_EDGE ( 'NONE', *, *, #1294, .T. ) ;
#18291=CARTESIAN_POINT ( 'NONE',  ( 71.75000000109248788, 11.46158073645647235, 13.53841926354352232 ) ) ;
#18306=CARTESIAN_POINT ( 'NONE',  ( -67.99999999999998579, 8.232233047033629347, 13.23223304703362402 ) ) ;
#18308=ORIENTED_EDGE ( 'NONE', *, *, #2192, .F. ) ;
#18333=CARTESIAN_POINT ( 'NONE',  ( -67.79999999999999716, 8.232233047033627571, 16.76776695296636532 ) ) ;
#18334=CARTESIAN_POINT ( 'NONE',  ( 66.30000000218494449, 8.232233047033627571, 16.76776695296636532 ) ) ;
#18335=CARTESIAN_POINT ( 'NONE',  ( 67.25000000109247367, 9.999999999999998224, 17.06698730000000097 ) ) ;
#18341=CARTESIAN_POINT ( 'NONE',  ( 67.00000000218494733, 9.999999999999998224, 17.49999999999999645 ) ) ;
#18345=CARTESIAN_POINT ( 'NONE',  ( -70.40000000109249356, 10.85617417291294551, 17.06698730000000097 ) ) ;
#18348=CARTESIAN_POINT ( 'NONE',  ( -71.60000000109246798, 7.933012699999995476, 15.85617417291294196 ) ) ;
#18356=CARTESIAN_POINT ( 'NONE',  ( -71.35000000109246798, 8.538419263543522320, 16.46158073645647235 ) ) ;
#18359=CARTESIAN_POINT ( 'NONE',  ( -69.65000000109246514, 12.06698730000000097, 14.99999999999999645 ) ) ;
#18367=CARTESIAN_POINT ( 'NONE',  ( -69.00000000218494733, 9.999999999999998224, 12.49999999999999289 ) ) ;
#18376=VERTEX_POINT ( 'NONE', #6680 ) ;
#18379=CARTESIAN_POINT ( 'NONE',  ( 69.20000000000000284, 11.76776695296636888, 16.76776695296636532 ) ) ;
#18382=DIRECTION ( 'NONE',  ( 0.000000000000000000, 0.000000000000000000, 1.000000000000000000 ) ) ;
#18385=CARTESIAN_POINT ( 'NONE',  ( 68.20000000000000284, 11.76776695296636888, 13.23223304703362579 ) ) ;
#18400=ORIENTED_EDGE ( 'NONE', *, *, #17438, .T. ) ;
#18410=CARTESIAN_POINT ( 'NONE',  ( 71.70000000109247651, 10.85617417291294551, 12.93301269999999370 ) ) ;
#18412=CARTESIAN_POINT ( 'NONE',  ( 71.45000000109247651, 9.999999999999998224, 17.06698730000000097 ) ) ;
#18419=DIRECTION ( 'NONE',  ( 1.000000000000000000, 0.000000000000000000, 0.000000000000000000 ) ) ;
#18443=CARTESIAN_POINT ( 'NONE',  ( -68.45000000000000284, 11.03553390593273598, 17.50000000000000355 ) ) ;
#18446=DIRECTION ( 'NONE',  ( -1.000000000000000000, -0.000000000000000000, -0.000000000000000000 ) ) ;
#18447=CARTESIAN_POINT ( 'NONE',  ( 66.65000000109247935, 7.933012699999995476, 14.99999999999999645 ) ) ;
#18451=( BOUNDED_CURVE ( )  B_SPLINE_CURVE ( 2, ( #1440, #14292, #4697, #19295, #5165, #10711, #8544, #2886, #15746 ),
 .UNSPECIFIED., .F., .F. ) 
 B_SPLINE_CURVE_WITH_KNOTS ( ( 3, 2, 2, 2, 3 ),
 ( 0.6875000000000001110, 0.7031250000000000000, 0.7187500000000000000, 0.7343749999999998890, 0.7499999999999997780 ),
 .UNSPECIFIED. ) 
 CURVE ( )  GEOMETRIC_REPRESENTATION_ITEM ( )  RATIONAL_B_SPLINE_CURVE ( ( 0.9999999999999994449, 0.9238795325112872936, 1.000000000000000000, 0.9238795325112867385, 1.000000000000000000, 0.9238795325112867385, 1.000000000000000000, 0.9238795325112878487, 0.9999999999999988898 ) ) 
 REPRESENTATION_ITEM ( '' )  );
#18456=CARTESIAN_POINT ( 'NONE',  ( -67.20000000218495018, 7.499999999999996447, 14.99999999999999645 ) ) ;
#18458=CARTESIAN_POINT ( 'NONE',  ( -69.40000000109249356, 12.06698729999999919, 14.14382582708705094 ) ) ;
#18461=CARTESIAN_POINT ( 'NONE',  ( -69.65000000109246514, 12.06698730000000097, 14.99999999999999645 ) ) ;
#18468=CARTESIAN_POINT ( 'NONE',  ( 71.29999999999998295, 9.999999999999998224, 12.49999999999999289 ) ) ;
#18470=CARTESIAN_POINT ( 'NONE',  ( -71.05000000109247082, 12.06698730000000097, 14.99999999999999645 ) ) ;
#18471=CARTESIAN_POINT ( 'NONE',  ( -69.55000000109247082, 11.46158073645647235, 13.53841926354352232 ) ) ;
#18478=CARTESIAN_POINT ( 'NONE',  ( 68.59999999999999432, 8.232233047033627571, 16.76776695296636532 ) ) ;
#18480=VERTEX_POINT ( 'NONE', #17927 ) ;
#18481=CARTESIAN_POINT ( 'NONE',  ( -71.50000000218496155, 11.76776695296636888, 13.23223304703362579 ) ) ;
#18487=CARTESIAN_POINT ( 'NONE',  ( 72.50000000000000000, 9.999999999999998224, 17.49999999999999645 ) ) ;
#18496=CARTESIAN_POINT ( 'NONE',  ( 69.45000000000000284, 7.499999999999995559, 16.03553390593273420 ) ) ;
#18502=CARTESIAN_POINT ( 'NONE',  ( 69.00000000218494733, 9.999999999999998224, 12.49999999999999289 ) ) ;
#18503=CARTESIAN_POINT ( 'NONE',  ( -70.95000000109247651, 8.538419263543524096, 13.53841926354352054 ) ) ;
#18508=CARTESIAN_POINT ( 'NONE',  ( -70.09999999999999432, 9.999999999999998224, 17.49999999999999645 ) ) ;
#18511=CARTESIAN_POINT ( 'NONE',  ( 72.50000000000000000, 9.999999999999998224, 17.49999999999999645 ) ) ;
#18519=CARTESIAN_POINT ( 'NONE',  ( 70.25000000109247367, 12.06698730000000097, 14.99999999999999645 ) ) ;
#18522=FACE_OUTER_BOUND ( 'NONE', #20182, .T. ) ;
#18523=CARTESIAN_POINT ( 'NONE',  ( 70.45000000109247651, 12.06698730000000097, 14.99999999999999645 ) ) ;
#18531=CARTESIAN_POINT ( 'NONE',  ( -66.05000000109247082, 7.933012699999995476, 14.99999999999999645 ) ) ;
#18536=CARTESIAN_POINT ( 'NONE',  ( 72.50000000000000000, 9.999999999999998224, 14.99999999999999645 ) ) ;
#18553=EDGE_CURVE ( 'NONE', #13175, #683, #3130, .T. ) ;
#18555=CARTESIAN_POINT ( 'NONE',  ( 69.55000000109247082, 11.46158073645647235, 13.53841926354352232 ) ) ;
#18562=CARTESIAN_POINT ( 'NONE',  ( 66.80000000109247082, 9.143825827087050939, 12.93301269999999370 ) ) ;
#18573=CARTESIAN_POINT ( 'NONE',  ( -68.40000000109249356, 9.143825827087052716, 12.93301269999999192 ) ) ;
#18576=CARTESIAN_POINT ( 'NONE',  ( -71.55000000109245661, 8.538419263543522320, 16.46158073645647235 ) ) ;
#18582=VERTEX_POINT ( 'NONE', #3895 ) ;
#18586=CARTESIAN_POINT ( 'NONE',  ( -68.80000000109247082, 10.85617417291294551, 17.06698729999999742 ) ) ;
#18588=CARTESIAN_POINT ( 'NONE',  ( 69.40000000109249356, 12.06698729999999919, 14.14382582708705094 ) ) ;
#18589=CARTESIAN_POINT ( 'NONE',  ( -71.30000000109247082, 12.06698730000000275, 15.85617417291294196 ) ) ;
#18590=( BOUNDED_CURVE ( )  B_SPLINE_CURVE ( 2, ( #14127, #7049, #5012, #17600, #16156, #8860, #12221, #14366, #2958 ),
 .UNSPECIFIED., .F., .F. ) 
 B_SPLINE_CURVE_WITH_KNOTS ( ( 3, 2, 2, 2, 3 ),
 ( 0.8749999999999990008, 0.8906249999999994449, 0.9062499999999998890, 0.9218750000000003331, 0.9375000000000007772 ),
 .UNSPECIFIED. ) 
 CURVE ( )  GEOMETRIC_REPRESENTATION_ITEM ( )  RATIONAL_B_SPLINE_CURVE ( ( 1.000000000000004885, 0.9238795325112818535, 1.000000000000000000, 0.9238795325112867385, 1.000000000000000000, 0.9238795325112867385, 1.000000000000000000, 0.9238795325112829637, 1.000000000000003775 ) ) 
 REPRESENTATION_ITEM ( '' )  );
#18592=CARTESIAN_POINT ( 'NONE',  ( 67.70000000000000284, 9.999999999999998224, 17.49999999999999645 ) ) ;
#18610=CARTESIAN_POINT ( 'NONE',  ( -65.52500000163871618, 9.999999999999998224, 17.28349365000000049 ) ) ;
#18615=CARTESIAN_POINT ( 'NONE',  ( 67.59999999999999432, 11.76776695296636888, 16.76776695296636532 ) ) ;
#18625=CARTESIAN_POINT ( 'NONE',  ( 65.52500000163871618, 9.999999999999998224, 17.28349365000000049 ) ) ;
#18632=CARTESIAN_POINT ( 'NONE',  ( -71.45000000109247651, 7.933012699999995476, 14.99999999999999645 ) ) ;
#18644=CARTESIAN_POINT ( 'NONE',  ( 72.05000000109247082, 9.999999999999998224, 17.06698730000000097 ) ) ;
#18646=FACE_OUTER_BOUND ( 'NONE', #6960, .T. ) ;
#18681=CARTESIAN_POINT ( 'NONE',  ( 71.45000000109247651, 9.999999999999998224, 17.06698730000000097 ) ) ;
#18684=DIRECTION ( 'NONE',  ( 0.000000000000000000, 0.000000000000000000, -1.000000000000000000 ) ) ;
#18685=CARTESIAN_POINT ( 'NONE',  ( 72.05000000109245661, 12.06698730000000097, 14.99999999999999645 ) ) ;
#18695=CARTESIAN_POINT ( 'NONE',  ( -66.80000000109247082, 9.143825827087052716, 12.93301269999999192 ) ) ;
#18698=CARTESIAN_POINT ( 'NONE',  ( -71.20000000109246230, 12.06698730000000275, 14.14382582708705094 ) ) ;
#18710=CARTESIAN_POINT ( 'NONE',  ( -66.75000000109247367, 8.538419263543524096, 13.53841926354352054 ) ) ;
#18711=CARTESIAN_POINT ( 'NONE',  ( 68.10000000109248219, 9.143825827087049163, 17.06698730000000097 ) ) ;
#18713=CARTESIAN_POINT ( 'NONE',  ( -66.70000000109246230, 9.143825827087049163, 17.06698729999999742 ) ) ;
#18714=AXIS2_PLACEMENT_3D ( 'NONE', #21494, #21734, #5106 ) ;
#18721=CARTESIAN_POINT ( 'NONE',  ( 68.74999999999998579, 7.499999999999996447, 13.96446609406725514 ) ) ;
#18732=EDGE_LOOP ( 'NONE', ( #7108, #12011, #16301, #8835 ) ) ;
#18738=EDGE_CURVE ( 'NONE', #3314, #16036, #3754, .T. ) ;
#18741=( BOUNDED_CURVE ( )  B_SPLINE_CURVE ( 2, ( #10705, #17984, #8897, #118, #22142, #7449, #18334, #3952, #13200 ),
 .UNSPECIFIED., .F., .F. ) 
 B_SPLINE_CURVE_WITH_KNOTS ( ( 3, 2, 2, 2, 3 ),
 ( 0.8124999999999993339, 0.8281249999999992228, 0.8437499999999991118, 0.8593749999999991118, 0.8749999999999990008 ),
 .UNSPECIFIED. ) 
 CURVE ( )  GEOMETRIC_REPRESENTATION_ITEM ( )  RATIONAL_B_SPLINE_CURVE ( ( 1.000000000000003331, 0.9238795325112835188, 1.000000000000000000, 0.9238795325112867385, 1.000000000000000000, 0.9238795325112867385, 1.000000000000000000, 0.9238795325112916235, 0.9999999999999951150 ) ) 
 REPRESENTATION_ITEM ( '' )  );
#18746=CARTESIAN_POINT ( 'NONE',  ( 67.84999999999999432, 7.499999999999995559, 16.03553390593273420 ) ) ;
#18754=CARTESIAN_POINT ( 'NONE',  ( -67.29999999999999716, 9.999999999999998224, 12.49999999999999289 ) ) ;
#18757=CYLINDRICAL_SURFACE ( 'NONE', #4596, 2.500000000000002220 ) ;
#18759=EDGE_CURVE ( 'NONE', #23355, #19246, #15411, .T. ) ;
#18760=CARTESIAN_POINT ( 'NONE',  ( -71.70000000109247651, 10.85617417291294551, 12.93301269999999370 ) ) ;
#18772=CARTESIAN_POINT ( 'NONE',  ( 70.05000000109247082, 9.999999999999998224, 12.93301269999999192 ) ) ;
#18774=CARTESIAN_POINT ( 'NONE',  ( 70.05000000109247082, 7.933012699999995476, 14.99999999999999645 ) ) ;
#18782=AXIS2_PLACEMENT_3D ( 'NONE', #1885, #3916, #9229 ) ;
#18784=CARTESIAN_POINT ( 'NONE',  ( -66.00000000109245946, 7.933012699999995476, 15.85617417291294196 ) ) ;
#18792=LINE ( 'NONE', #922, #20476 ) ;
#18803=CARTESIAN_POINT ( 'NONE',  ( 70.60000000109246798, 10.85617417291294551, 17.06698730000000097 ) ) ;
#18804=EDGE_LOOP ( 'NONE', ( #11328, #10278, #6980, #15157 ) ) ;
#18807=CARTESIAN_POINT ( 'NONE',  ( 67.30000000109247082, 9.143825827087049163, 17.06698729999999742 ) ) ;
#18812=CARTESIAN_POINT ( 'NONE',  ( 72.50000000000000000, 9.999999999999998224, 17.49999999999999645 ) ) ;
#18816=CARTESIAN_POINT ( 'NONE',  ( -66.45000000109247651, 9.999999999999998224, 17.06698730000000097 ) ) ;
#18819=CARTESIAN_POINT ( 'NONE',  ( -70.30000000109248504, 10.85617417291294551, 12.93301269999999370 ) ) ;
#18823=ORIENTED_EDGE ( 'NONE', *, *, #6464, .F. ) ;
#18827=CARTESIAN_POINT ( 'NONE',  ( -68.90000000109247935, 9.143825827087049163, 17.06698729999999742 ) ) ;
#18828=CARTESIAN_POINT ( 'NONE',  ( 70.50000000109247367, 9.143825827087049163, 17.06698730000000097 ) ) ;
#18830=CARTESIAN_POINT ( 'NONE',  ( -66.35000000109246798, 11.46158073645647235, 13.53841926354352232 ) ) ;
#18833=CARTESIAN_POINT ( 'NONE',  ( -65.97500000054623115, 9.999999999999998224, 17.28349365000000049 ) ) ;
#18850=CARTESIAN_POINT ( 'NONE',  ( -71.00000000218494733, 9.999999999999998224, 17.49999999999999645 ) ) ;
#18854=CARTESIAN_POINT ( 'NONE',  ( 66.74999999999998579, 12.50000000000000000, 16.03553390593273420 ) ) ;
#18857=CARTESIAN_POINT ( 'NONE',  ( 68.15000000109247935, 8.538419263543522320, 16.46158073645647235 ) ) ;
#18864=CARTESIAN_POINT ( 'NONE',  ( -71.60000000109246798, 7.933012699999995476, 15.85617417291294196 ) ) ;
#18869=CARTESIAN_POINT ( 'NONE',  ( -71.85000000109246798, 12.06698730000000097, 14.99999999999999645 ) ) ;
#18878=UNCERTAINTY_MEASURE_WITH_UNIT (LENGTH_MEASURE( 1.000000000000000082E-05 ), #10914, 'distance_accuracy_value', 'NONE');
#18880=CARTESIAN_POINT ( 'NONE',  ( 69.05000000109247082, 7.933012699999995476, 14.99999999999999645 ) ) ;
#18881=CARTESIAN_POINT ( 'NONE',  ( 69.85000000109246798, 9.999999999999998224, 17.06698730000000097 ) ) ;
#18889=CARTESIAN_POINT ( 'NONE',  ( 66.75000000218494733, 12.50000000000000000, 13.96446609406725692 ) ) ;
#18892=CARTESIAN_POINT ( 'NONE',  ( -66.65000000109247935, 9.999999999999998224, 17.06698730000000097 ) ) ;
#18906=CARTESIAN_POINT ( 'NONE',  ( 71.05000000109247082, 12.06698730000000097, 14.99999999999999645 ) ) ;
#18911=CARTESIAN_POINT ( 'NONE',  ( 69.15000000109246514, 8.538419263543522320, 16.46158073645647235 ) ) ;
#18913=LINE ( 'NONE', #2619, #2232 ) ;
#18916=CARTESIAN_POINT ( 'NONE',  ( 70.35000000109246798, 11.46158073645647235, 13.53841926354352232 ) ) ;
#18930=CARTESIAN_POINT ( 'NONE',  ( -65.65000000109247935, 9.999999999999998224, 17.06698730000000097 ) ) ;
#18931=ORIENTED_EDGE ( 'NONE', *, *, #7963, .T. ) ;
#18933=CARTESIAN_POINT ( 'NONE',  ( -68.65000000109246514, 9.999999999999998224, 12.93301269999999192 ) ) ;
#18942=CARTESIAN_POINT ( 'NONE',  ( -67.00000000109247367, 12.06698730000000275, 14.14382582708705094 ) ) ;
#18944=CARTESIAN_POINT ( 'NONE',  ( 68.85000000109248219, 9.999999999999998224, 17.06698730000000097 ) ) ;
#18945=CARTESIAN_POINT ( 'NONE',  ( -67.65000000109247935, 7.933012699999995476, 14.99999999999999645 ) ) ;
#18954=ORIENTED_EDGE ( 'NONE', *, *, #23224, .F. ) ;
#18967=CARTESIAN_POINT ( 'NONE',  ( -70.20000000218495018, 9.999999999999998224, 17.49999999999999645 ) ) ;
#18972=CARTESIAN_POINT ( 'NONE',  ( 71.15000000109247935, 11.46158073645647235, 16.46158073645647235 ) ) ;
#18983=CARTESIAN_POINT ( 'NONE',  ( -69.60000000109249640, 10.85617417291294551, 17.06698729999999742 ) ) ;
#18993=CARTESIAN_POINT ( 'NONE',  ( 67.40000000109247935, 7.933012699999995476, 15.85617417291294196 ) ) ;
#18994=CARTESIAN_POINT ( 'NONE',  ( 69.70000000109246230, 12.06698730000000275, 15.85617417291294196 ) ) ;
#19010=CARTESIAN_POINT ( 'NONE',  ( 69.20000000218495018, 12.50000000000000000, 14.99999999999999645 ) ) ;
#19029=CARTESIAN_POINT ( 'NONE',  ( 67.25000000109245946, 12.06698730000000097, 14.99999999999999645 ) ) ;
#19034=CARTESIAN_POINT ( 'NONE',  ( 70.90000000109245093, 7.933012699999995476, 14.14382582708705094 ) ) ;
#19047=CARTESIAN_POINT ( 'NONE',  ( -66.60000000109246798, 10.85617417291294551, 17.06698729999999742 ) ) ;
#19060=CARTESIAN_POINT ( 'NONE',  ( -68.45000000109247651, 9.999999999999998224, 12.93301269999999192 ) ) ;
#19061=CARTESIAN_POINT ( 'NONE',  ( 69.50000000109247367, 12.06698729999999919, 15.85617417291294196 ) ) ;
#19063=CARTESIAN_POINT ( 'NONE',  ( -67.05000000109247082, 9.999999999999998224, 12.93301269999999192 ) ) ;
#19070=CARTESIAN_POINT ( 'NONE',  ( 71.50000000000000000, 12.50000000000000000, 14.99999999999999645 ) ) ;
#19072=DIRECTION ( 'NONE',  ( -1.000000000000000000, -0.000000000000000000, -0.000000000000000000 ) ) ;
#19081=VERTEX_POINT ( 'NONE', #515 ) ;
#19088=CARTESIAN_POINT ( 'NONE',  ( -69.90000000218495302, 11.76776695296636888, 13.23223304703362579 ) ) ;
#19096=CARTESIAN_POINT ( 'NONE',  ( 71.00000000109247367, 12.06698730000000275, 14.14382582708705094 ) ) ;
#19103=CARTESIAN_POINT ( 'NONE',  ( -69.75000000109245946, 11.46158073645647235, 16.46158073645647235 ) ) ;
#19108=CARTESIAN_POINT ( 'NONE',  ( -70.89999999999999147, 9.999999999999998224, 17.49999999999999645 ) ) ;
#19114=LINE ( 'NONE', #15318, #13692 ) ;
#19120=CARTESIAN_POINT ( 'NONE',  ( 69.20000000109246230, 9.143825827087050939, 12.93301269999999370 ) ) ;
#19123=CARTESIAN_POINT ( 'NONE',  ( 68.30000000109247082, 9.143825827087049163, 17.06698729999999742 ) ) ;
#19124=EDGE_LOOP ( 'NONE', ( #1164, #13687, #8947, #20428, #3292 ) ) ;
#19125=EDGE_CURVE ( 'NONE', #19131, #3314, #23354, .T. ) ;
#19131=VERTEX_POINT ( 'NONE', #12884 ) ;
#19141=CARTESIAN_POINT ( 'NONE',  ( -71.00000000218494733, 9.999999999999998224, 17.49999999999999645 ) ) ;
#19142=ORIENTED_EDGE ( 'NONE', *, *, #21216, .T. ) ;
#19149=CARTESIAN_POINT ( 'NONE',  ( 68.45000000109247651, 7.933012699999995476, 14.99999999999999645 ) ) ;
#19156=CARTESIAN_POINT ( 'NONE',  ( 70.55000000109245661, 11.46158073645647235, 16.46158073645647235 ) ) ;
#19170=CARTESIAN_POINT ( 'NONE',  ( -68.95000000109247651, 11.46158073645647235, 16.46158073645647235 ) ) ;
#19181=CARTESIAN_POINT ( 'NONE',  ( 66.85000000109248219, 9.999999999999998224, 12.93301269999999192 ) ) ;
#19182=CARTESIAN_POINT ( 'NONE',  ( -67.55000000109247082, 8.538419263543522320, 16.46158073645647235 ) ) ;
#19184=CARTESIAN_POINT ( 'NONE',  ( -71.39999999999999147, 11.76776695296636888, 13.23223304703362579 ) ) ;
#19190=CYLINDRICAL_SURFACE ( 'NONE', #22951, 2.500000000000002220 ) ;
#19191=EDGE_CURVE ( 'NONE', #9434, #21422, #14685, .T. ) ;
#19192=EDGE_CURVE ( 'NONE', #13424, #7292, #14637, .T. ) ;
#19203=DIRECTION ( 'NONE',  ( -1.000000000000000000, -0.000000000000000000, -0.000000000000000000 ) ) ;
#19206=CARTESIAN_POINT ( 'NONE',  ( -69.40000000218495302, 9.999999999999998224, 17.49999999999999645 ) ) ;
#19207=CARTESIAN_POINT ( 'NONE',  ( -72.15000000109247935, 9.999999999999998224, 17.06698730000000097 ) ) ;
#19211=CARTESIAN_POINT ( 'NONE',  ( -70.89999999999999147, 9.999999999999998224, 17.49999999999999645 ) ) ;
#19212=CARTESIAN_POINT ( 'NONE',  ( 69.25000000109247367, 9.999999999999998224, 12.93301269999999192 ) ) ;
#19220=CARTESIAN_POINT ( 'NONE',  ( -69.10000000109246798, 9.143825827087049163, 17.06698730000000097 ) ) ;
#19228=DIRECTION ( 'NONE',  ( -1.000000000000000000, -0.000000000000000000, -0.000000000000000000 ) ) ;
#19229=CARTESIAN_POINT ( 'NONE',  ( -66.59999999999999432, 11.76776695296636888, 13.23223304703362579 ) ) ;
#19232=CARTESIAN_POINT ( 'NONE',  ( 68.05000000109247082, 9.999999999999998224, 17.06698730000000097 ) ) ;
#19233=CARTESIAN_POINT ( 'NONE',  ( 66.90000000109246514, 7.933012699999995476, 14.14382582708705094 ) ) ;
#19246=VERTEX_POINT ( 'NONE', #15278 ) ;
#19252=CARTESIAN_POINT ( 'NONE',  ( 71.25000000218494733, 7.499999999999996447, 13.96446609406725514 ) ) ;
#19254=CARTESIAN_POINT ( 'NONE',  ( -68.25000000218493312, 11.03553390593269157, 12.49999999999994849 ) ) ;
#19258=CARTESIAN_POINT ( 'NONE',  ( 70.60000000218494165, 9.999999999999998224, 12.49999999999999289 ) ) ;
#19261=CARTESIAN_POINT ( 'NONE',  ( 67.90000000109246514, 10.85617417291294551, 12.93301269999999192 ) ) ;
#19265=CARTESIAN_POINT ( 'NONE',  ( 69.55000000109247082, 11.46158073645647235, 13.53841926354352232 ) ) ;
#19277=CARTESIAN_POINT ( 'NONE',  ( -66.30000000109247082, 10.85617417291294551, 12.93301269999999370 ) ) ;
#19286=CARTESIAN_POINT ( 'NONE',  ( -66.00000000109247367, 9.143825827087050939, 12.93301269999999370 ) ) ;
#19289=CARTESIAN_POINT ( 'NONE',  ( -71.64999999999997726, 11.03553390593273598, 17.50000000000000355 ) ) ;
#19293=PLANE ( 'NONE',  #117 ) ;
#19295=CARTESIAN_POINT ( 'NONE',  ( 67.25000000218494733, 7.499999999999996447, 13.96446609406725514 ) ) ;
#19314=CARTESIAN_POINT ( 'NONE',  ( -67.10000000218495586, 8.232233047033627571, 16.76776695296636532 ) ) ;
#19322=CARTESIAN_POINT ( 'NONE',  ( 68.85000000109248219, 9.999999999999998224, 17.06698730000000097 ) ) ;
#19324=CARTESIAN_POINT ( 'NONE',  ( 68.20000000218495018, 9.999999999999998224, 12.49999999999999289 ) ) ;
#19330=CARTESIAN_POINT ( 'NONE',  ( -68.75000000109245946, 11.46158073645647235, 13.53841926354352232 ) ) ;
#19345=CARTESIAN_POINT ( 'NONE',  ( 68.25000000109247367, 7.933012699999995476, 14.99999999999999645 ) ) ;
#19347=CARTESIAN_POINT ( 'NONE',  ( 68.10000000109245377, 12.06698730000000275, 15.85617417291294196 ) ) ;
#19362=CARTESIAN_POINT ( 'NONE',  ( 71.55000000109247082, 8.538419263543524096, 13.53841926354352054 ) ) ;
#19364=CARTESIAN_POINT ( 'NONE',  ( -68.20000000218495018, 9.999999999999998224, 12.49999999999999289 ) ) ;
#19368=CARTESIAN_POINT ( 'NONE',  ( 71.70000000218495018, 11.76776695296636888, 16.76776695296636532 ) ) ;
#19372=CARTESIAN_POINT ( 'NONE',  ( 67.95000000109247651, 11.46158073645647235, 13.53841926354352232 ) ) ;
#19375=DIRECTION ( 'NONE',  ( -1.000000000000000000, -0.000000000000000000, -0.000000000000000000 ) ) ;
#19376=CARTESIAN_POINT ( 'NONE',  ( 69.50000000109247367, 10.85617417291294551, 12.93301269999999370 ) ) ;
#19386=( BOUNDED_CURVE ( )  B_SPLINE_CURVE ( 2, ( #333, #2696, #4489, #17205, #6301, #1125, #14990, #20880, #10038 ),
 .UNSPECIFIED., .F., .F. ) 
 B_SPLINE_CURVE_WITH_KNOTS ( ( 3, 2, 2, 2, 3 ),
 ( 0.2500000000000006661, 0.2656250000000005551, 0.2812500000000004441, 0.2968750000000003886, 0.3125000000000002776 ),
 .UNSPECIFIED. ) 
 CURVE ( )  GEOMETRIC_REPRESENTATION_ITEM ( )  RATIONAL_B_SPLINE_CURVE ( ( 0.9999999999999967804, 0.9238795325112899581, 1.000000000000000000, 0.9238795325112867385, 1.000000000000000000, 0.9238795325112867385, 1.000000000000000000, 0.9238795325112854062, 1.000000000000001332 ) ) 
 REPRESENTATION_ITEM ( '' )  );
#19391=CARTESIAN_POINT ( 'NONE',  ( -67.50000000109245946, 9.143825827087049163, 17.06698729999999742 ) ) ;
#19401=CARTESIAN_POINT ( 'NONE',  ( -66.05000000109247082, 9.999999999999998224, 12.93301269999999192 ) ) ;
#19403=CARTESIAN_POINT ( 'NONE',  ( -71.39999999999999147, 11.76776695296636888, 13.23223304703362579 ) ) ;
#19418=CARTESIAN_POINT ( 'NONE',  ( -70.15000000109247935, 11.46158073645647235, 13.53841926354352232 ) ) ;
#19430=CARTESIAN_POINT ( 'NONE',  ( -66.00000000218494733, 12.50000000000000000, 14.99999999999999645 ) ) ;
#19434=CARTESIAN_POINT ( 'NONE',  ( -71.60000000109246798, 7.933012699999995476, 15.85617417291294196 ) ) ;
#19445=CARTESIAN_POINT ( 'NONE',  ( 67.45000000218493597, 11.03553390593273420, 12.49999999999998934 ) ) ;
#19448=CARTESIAN_POINT ( 'NONE',  ( -67.80000000109247082, 9.143825827087052716, 12.93301269999999192 ) ) ;
#19457=EDGE_CURVE ( 'NONE', #17245, #5464, #3898, .T. ) ;
#19460=ORIENTED_EDGE ( 'NONE', *, *, #23224, .T. ) ;
#19462=VECTOR ( 'NONE', #4653, 1000.000000000000000 ) ;
#19470=CARTESIAN_POINT ( 'NONE',  ( 68.00000000109245946, 12.06698730000000275, 14.14382582708705094 ) ) ;
#19488=CARTESIAN_POINT ( 'NONE',  ( -67.45000000000000284, 12.50000000000000000, 13.96446609406725692 ) ) ;
#19495=CARTESIAN_POINT ( 'NONE',  ( 69.65000000218496723, 7.499999999999995559, 13.96446609406725692 ) ) ;
#19497=( BOUNDED_CURVE ( )  B_SPLINE_CURVE ( 2, ( #4015, #16960, #20768, #13143, #4260, #16602, #14825, #22078, #5697 ),
 .UNSPECIFIED., .F., .F. ) 
 B_SPLINE_CURVE_WITH_KNOTS ( ( 3, 2, 2, 2, 3 ),
 ( 0.06249999999999961836, 0.07812499999999952816, 0.09374999999999943101, 0.1093749999999993339, 0.1249999999999992367 ),
 .UNSPECIFIED. ) 
 CURVE ( )  GEOMETRIC_REPRESENTATION_ITEM ( )  RATIONAL_B_SPLINE_CURVE ( ( 1.000000000000001776, 0.9238795325112848511, 1.000000000000000000, 0.9238795325112867385, 1.000000000000000000, 0.9238795325112867385, 1.000000000000000000, 0.9238795325112904022, 0.9999999999999963363 ) ) 
 REPRESENTATION_ITEM ( '' )  );
#19499=CARTESIAN_POINT ( 'NONE',  ( 68.35000000109246798, 8.538419263543522320, 16.46158073645647235 ) ) ;
#19522=ORIENTED_EDGE ( 'NONE', *, *, #3329, .F. ) ;
#19526=CARTESIAN_POINT ( 'NONE',  ( -67.95000000218495018, 7.499999999999996447, 16.03553390593273775 ) ) ;
#19527=CARTESIAN_POINT ( 'NONE',  ( 65.75000000109247367, 8.538419263543522320, 16.46158073645647235 ) ) ;
#19529=CARTESIAN_POINT ( 'NONE',  ( -68.74999999999998579, 7.499999999999995559, 13.96446609406725692 ) ) ;
#19543=CARTESIAN_POINT ( 'NONE',  ( -67.95000000109247651, 11.46158073645647235, 16.46158073645647235 ) ) ;
#19550=EDGE_LOOP ( 'NONE', ( #2133, #3901, #9244, #5672 ) ) ;
#19553=CARTESIAN_POINT ( 'NONE',  ( -68.95000000218495018, 8.964466094067258695, 12.49999999999999289 ) ) ;
#19562=CARTESIAN_POINT ( 'NONE',  ( 72.50000000000000000, 9.999999999999998224, 12.49999999999999289 ) ) ;
#19567=ORIENTED_EDGE ( 'NONE', *, *, #11893, .T. ) ;
#19572=VERTEX_POINT ( 'NONE', #8884 ) ;
#19582=CARTESIAN_POINT ( 'NONE',  ( 66.15000000109247935, 8.538419263543524096, 13.53841926354352054 ) ) ;
#19584=ADVANCED_FACE ( 'NONE', ( #23351 ), #17846, .T. ) ;
#19593=CARTESIAN_POINT ( 'NONE',  ( 72.50000000000000000, 9.999999999999998224, 14.99999999999999645 ) ) ;
#19597=CARTESIAN_POINT ( 'NONE',  ( -66.49999999999998579, 9.999999999999998224, 12.49999999999999289 ) ) ;
#19606=CARTESIAN_POINT ( 'NONE',  ( 67.10000000218495586, 8.232233047033627571, 16.76776695296636532 ) ) ;
#19615=CARTESIAN_POINT ( 'NONE',  ( 67.40000000109247935, 10.85617417291294551, 17.06698729999999742 ) ) ;
#19628=CARTESIAN_POINT ( 'NONE',  ( -66.00000000109245946, 7.933012699999995476, 15.85617417291294196 ) ) ;
#19638=CARTESIAN_POINT ( 'NONE',  ( -68.20000000218495018, 9.999999999999998224, 12.49999999999999289 ) ) ;
#19639=CARTESIAN_POINT ( 'NONE',  ( 67.10000000109248219, 12.06698729999999919, 15.85617417291294196 ) ) ;
#19643=CARTESIAN_POINT ( 'NONE',  ( -69.14999999999999147, 12.50000000000000000, 16.03553390593273420 ) ) ;
#19655=CARTESIAN_POINT ( 'NONE',  ( -66.45000000109247651, 9.999999999999998224, 17.06698730000000097 ) ) ;
#19662=FACE_OUTER_BOUND ( 'NONE', #19550, .T. ) ;
#19666=CARTESIAN_POINT ( 'NONE',  ( -67.80000000218494449, 9.999999999999998224, 17.49999999999999645 ) ) ;
#19693=CARTESIAN_POINT ( 'NONE',  ( -69.70000000218495018, 8.232233047033629347, 13.23223304703362402 ) ) ;
#19697=CARTESIAN_POINT ( 'NONE',  ( 71.14999999999999147, 7.499999999999995559, 13.96446609406725692 ) ) ;
#19698=AXIS2_PLACEMENT_3D ( 'NONE', #2717, #914, #4640 ) ;
#19711=CARTESIAN_POINT ( 'NONE',  ( 68.14999999999999147, 11.03553390593273420, 12.49999999999998934 ) ) ;
#19725=CARTESIAN_POINT ( 'NONE',  ( 68.70000000218495018, 8.232233047033627571, 16.76776695296636532 ) ) ;
#19743=CARTESIAN_POINT ( 'NONE',  ( 66.59999999999999432, 11.76776695296636888, 13.23223304703362579 ) ) ;
#19750=CARTESIAN_POINT ( 'NONE',  ( -65.80000000218494449, 9.999999999999998224, 12.49999999999999289 ) ) ;
#19756=CARTESIAN_POINT ( 'NONE',  ( -66.09999999999999432, 9.999999999999998224, 17.49999999999999645 ) ) ;
#19760=CARTESIAN_POINT ( 'NONE',  ( -67.70000000000000284, 9.999999999999998224, 17.49999999999999645 ) ) ;
#19765=CARTESIAN_POINT ( 'NONE',  ( -67.50000000218494733, 11.76776695296636888, 13.23223304703362579 ) ) ;
#19767=CARTESIAN_POINT ( 'NONE',  ( 67.70000000000000284, 9.999999999999998224, 17.49999999999999645 ) ) ;
#19769=CARTESIAN_POINT ( 'NONE',  ( -66.50000000218494733, 8.232233047033629347, 13.23223304703362402 ) ) ;
#19772=CARTESIAN_POINT ( 'NONE',  ( -71.65000000109247935, 9.999999999999998224, 12.93301269999999192 ) ) ;
#19775=CARTESIAN_POINT ( 'NONE',  ( -68.65000000109247935, 12.06698730000000097, 14.99999999999999645 ) ) ;
#19778=DIRECTION ( 'NONE',  ( 0.000000000000000000, 0.000000000000000000, 1.000000000000000000 ) ) ;
#19787=CARTESIAN_POINT ( 'NONE',  ( -67.50000000218494733, 11.76776695296636888, 13.23223304703362579 ) ) ;
#19790=CARTESIAN_POINT ( 'NONE',  ( -72.05000000109245661, 12.06698730000000097, 14.99999999999999645 ) ) ;
#19800=CARTESIAN_POINT ( 'NONE',  ( -68.14999999999999147, 11.03553390593273420, 12.49999999999998934 ) ) ;
#19801=ORIENTED_EDGE ( 'NONE', *, *, #15530, .F. ) ;
#19808=LINE ( 'NONE', #18138, #1714 ) ;
#19819=CARTESIAN_POINT ( 'NONE',  ( -70.60000000218494165, 9.999999999999998224, 12.49999999999999289 ) ) ;
#19820=CARTESIAN_POINT ( 'NONE',  ( 71.45000000000000284, 12.50000000000000000, 13.96446609406725869 ) ) ;
#19827=CARTESIAN_POINT ( 'NONE',  ( -70.35000000218495586, 7.499999999999996447, 16.03553390593273775 ) ) ;
#19843=CARTESIAN_POINT ( 'NONE',  ( 66.95000000218496439, 11.03553390593273598, 17.50000000000000355 ) ) ;
#19868=CARTESIAN_POINT ( 'NONE',  ( -65.95000000109246230, 8.538419263543522320, 16.46158073645647235 ) ) ;
#19871=CARTESIAN_POINT ( 'NONE',  ( -65.95000000218495018, 12.50000000000000000, 13.96446609406725692 ) ) ;
#19872=ORIENTED_EDGE ( 'NONE', *, *, #10467, .T. ) ;
#19874=ADVANCED_BREP_SHAPE_REPRESENTATION ( '', ( #13661, #7318 ), #14589 ) ;
#19883=CARTESIAN_POINT ( 'NONE',  ( -68.20000000000000284, 11.76776695296636888, 13.23223304703362579 ) ) ;
#19890=CARTESIAN_POINT ( 'NONE',  ( -66.25000000109245946, 9.999999999999998224, 12.93301269999999192 ) ) ;
#19891=CARTESIAN_POINT ( 'NONE',  ( 67.89999999999999147, 7.499999999999996447, 14.99999999999999645 ) ) ;
#19898=CARTESIAN_POINT ( 'NONE',  ( -66.40000000109247935, 10.85617417291294551, 17.06698729999999742 ) ) ;
#19907=CARTESIAN_POINT ( 'NONE',  ( -65.45000000218496439, 8.964466094067258695, 17.50000000000000355 ) ) ;
#19909=CARTESIAN_POINT ( 'NONE',  ( -68.55000000109247082, 8.538419263543524096, 13.53841926354352054 ) ) ;
#19915=CARTESIAN_POINT ( 'NONE',  ( 66.90000000000000568, 9.999999999999998224, 17.49999999999999645 ) ) ;
#19920=CARTESIAN_POINT ( 'NONE',  ( -68.20000000000000284, 11.76776695296636888, 13.23223304703362579 ) ) ;
#19937=CARTESIAN_POINT ( 'NONE',  ( 70.34999999999999432, 7.499999999999995559, 13.96446609406725692 ) ) ;
#19938=EDGE_CURVE ( 'NONE', #4847, #4037, #5448, .T. ) ;
#19940=EDGE_CURVE ( 'NONE', #4468, #8256, #11631, .T. ) ;
#19941=CARTESIAN_POINT ( 'NONE',  ( 69.45000000218495018, 8.964466094067256918, 17.49999999999999289 ) ) ;
#19950=CARTESIAN_POINT ( 'NONE',  ( 68.29999999999999716, 12.50000000000000000, 14.99999999999999645 ) ) ;
#19951=PLANE ( 'NONE',  #22695 ) ;
#19953=VERTEX_POINT ( 'NONE', #2601 ) ;
#19960=CARTESIAN_POINT ( 'NONE',  ( 66.50000000218494733, 8.232233047033629347, 13.23223304703362402 ) ) ;
#19962=CARTESIAN_POINT ( 'NONE',  ( -68.89999999999999147, 9.999999999999998224, 12.49999999999999289 ) ) ;
#19969=CARTESIAN_POINT ( 'NONE',  ( 66.55000000109247082, 11.46158073645647235, 16.46158073645647235 ) ) ;
#19972=ORIENTED_EDGE ( 'NONE', *, *, #6434, .F. ) ;
#19982=CARTESIAN_POINT ( 'NONE',  ( 69.99999999999998579, 11.76776695296636888, 16.76776695296636532 ) ) ;
#19990=CARTESIAN_POINT ( 'NONE',  ( -68.14999999999999147, 11.03553390593273598, 12.49999999999999289 ) ) ;
#19996=CARTESIAN_POINT ( 'NONE',  ( 67.84999999999999432, 7.499999999999996447, 16.03553390593273775 ) ) ;
#20001=CARTESIAN_POINT ( 'NONE',  ( -68.90000000109247935, 9.143825827087049163, 17.06698730000000097 ) ) ;
#20004=CARTESIAN_POINT ( 'NONE',  ( -67.10000000109248219, 12.06698730000000275, 15.85617417291294196 ) ) ;
#20014=CARTESIAN_POINT ( 'NONE',  ( -69.55000000109247082, 11.46158073645647235, 16.46158073645647235 ) ) ;
#20015=CARTESIAN_POINT ( 'NONE',  ( -68.50000000109245946, 7.933012699999995476, 14.14382582708705094 ) ) ;
#20019=CARTESIAN_POINT ( 'NONE',  ( 71.95000000000001705, 7.499999999999996447, 13.96446609406725514 ) ) ;
#20022=LINE ( 'NONE', #19562, #18095 ) ;
#20041=DIRECTION ( 'NONE',  ( 0.000000000000000000, 0.000000000000000000, 1.000000000000000000 ) ) ;
#20043=CARTESIAN_POINT ( 'NONE',  ( 70.09999999999999432, 9.999999999999998224, 17.49999999999999645 ) ) ;
#20051=CARTESIAN_POINT ( 'NONE',  ( 72.37500000054622262, 9.999999999999998224, 17.28349365000000049 ) ) ;
#20057=CARTESIAN_POINT ( 'NONE',  ( 67.80000000218494449, 9.999999999999998224, 17.49999999999999645 ) ) ;
#20061=EDGE_CURVE ( 'NONE', #11744, #13392, #19808, .T. ) ;
#20068=EDGE_CURVE ( 'NONE', #23046, #13424, #1363, .T. ) ;
#20072=CARTESIAN_POINT ( 'NONE',  ( 65.85000000218495586, 11.03553390593273598, 12.49999999999999289 ) ) ;
#20096=ORIENTED_EDGE ( 'NONE', *, *, #21389, .T. ) ;
#20105=CARTESIAN_POINT ( 'NONE',  ( 66.40000000109247935, 10.85617417291294551, 17.06698729999999742 ) ) ;
#20108=( BOUNDED_CURVE ( )  B_SPLINE_CURVE ( 2, ( #10908, #16629, #14856, #5732, #1769, #93, #3810, #14622, #21882 ),
 .UNSPECIFIED., .F., .F. ) 
 B_SPLINE_CURVE_WITH_KNOTS ( ( 3, 2, 2, 2, 3 ),
 ( 0.000000000000000000, 0.01562499999999990459, 0.03124999999999980918, 0.04687499999999971551, 0.06249999999999961836 ),
 .UNSPECIFIED. ) 
 CURVE ( )  GEOMETRIC_REPRESENTATION_ITEM ( )  RATIONAL_B_SPLINE_CURVE ( ( 1.000000000000000000, 0.9238795325112867385, 1.000000000000000000, 0.9238795325112867385, 1.000000000000000000, 0.9238795325112867385, 1.000000000000000000, 0.9238795325112886259, 0.9999999999999981126 ) ) 
 REPRESENTATION_ITEM ( '' )  );
#20110=CARTESIAN_POINT ( 'NONE',  ( 68.40000000218495302, 12.50000000000000000, 14.99999999999999645 ) ) ;
#20114=CARTESIAN_POINT ( 'NONE',  ( -68.00000000109247367, 10.85617417291294551, 17.06698730000000097 ) ) ;
#20117=CARTESIAN_POINT ( 'NONE',  ( -72.15000000109246514, 11.46158073645647235, 16.46158073645647235 ) ) ;
#20124=CARTESIAN_POINT ( 'NONE',  ( -71.60000000109246798, 9.143825827087050939, 12.93301269999999370 ) ) ;
#20127=CARTESIAN_POINT ( 'NONE',  ( -69.40000000109246514, 9.143825827087050939, 12.93301269999999370 ) ) ;
#20159=CARTESIAN_POINT ( 'NONE',  ( 69.84999999999999432, 12.50000000000000000, 13.96446609406725869 ) ) ;
#20172=VERTEX_POINT ( 'NONE', #4115 ) ;
#20175=FACE_OUTER_BOUND ( 'NONE', #20585, .T. ) ;
#20182=EDGE_LOOP ( 'NONE', ( #22791, #399 ) ) ;
#20186=CARTESIAN_POINT ( 'NONE',  ( 70.60000000109246798, 7.933012699999995476, 15.85617417291294196 ) ) ;
#20189=CARTESIAN_POINT ( 'NONE',  ( 72.05000000109245661, 12.06698730000000097, 14.99999999999999645 ) ) ;
#20192=ORIENTED_EDGE ( 'NONE', *, *, #10467, .F. ) ;
#20204=ORIENTED_EDGE ( 'NONE', *, *, #18738, .T. ) ;
#20209=ORIENTED_EDGE ( 'NONE', *, *, #4804, .F. ) ;
#20225=VERTEX_POINT ( 'NONE', #18487 ) ;
#20227=CARTESIAN_POINT ( 'NONE',  ( -66.84999999999999432, 11.03553390593273598, 17.50000000000000355 ) ) ;
#20230=CARTESIAN_POINT ( 'NONE',  ( 67.65000000109247935, 9.999999999999998224, 12.93301269999999192 ) ) ;
#20233=EDGE_CURVE ( 'NONE', #23046, #433, #7907, .T. ) ;
#20242=CARTESIAN_POINT ( 'NONE',  ( -68.25000000109247367, 7.933012699999995476, 14.99999999999999645 ) ) ;
#20245=CARTESIAN_POINT ( 'NONE',  ( -71.65000000109246514, 7.933012699999995476, 14.99999999999999645 ) ) ;
#20252=CARTESIAN_POINT ( 'NONE',  ( 71.14999999999999147, 7.499999999999996447, 13.96446609406725514 ) ) ;
#20254=CARTESIAN_POINT ( 'NONE',  ( -70.85000000109246798, 9.999999999999998224, 12.93301269999999192 ) ) ;
#20256=CARTESIAN_POINT ( 'NONE',  ( -70.95000000109247651, 8.538419263543524096, 13.53841926354352054 ) ) ;
#20259=CARTESIAN_POINT ( 'NONE',  ( 65.97500000054623115, 9.999999999999998224, 17.28349365000000049 ) ) ;
#20265=CARTESIAN_POINT ( 'NONE',  ( 68.54999999999998295, 8.964466094067287116, 17.50000000000002487 ) ) ;
#20268=CARTESIAN_POINT ( 'NONE',  ( 69.95000000218493597, 12.50000000000000000, 13.96446609406725692 ) ) ;
#20269=CARTESIAN_POINT ( 'NONE',  ( -70.50000000000000000, 9.999999999999998224, 12.49999999999999289 ) ) ;
#20285=CARTESIAN_POINT ( 'NONE',  ( 69.39999999999999147, 8.232233047033627571, 16.76776695296636532 ) ) ;
#20286=CARTESIAN_POINT ( 'NONE',  ( 72.50000000000000000, 9.999999999999998224, 14.99999999999999645 ) ) ;
#20308=CARTESIAN_POINT ( 'NONE',  ( 71.30000000109248504, 9.143825827087049163, 17.06698729999999742 ) ) ;
#20309=DIRECTION ( 'NONE',  ( 0.000000000000000000, 0.000000000000000000, -1.000000000000000000 ) ) ;
#20318=CARTESIAN_POINT ( 'NONE',  ( -67.45000000109246230, 9.999999999999998224, 17.06698730000000097 ) ) ;
#20340=CARTESIAN_POINT ( 'NONE',  ( 69.80000000109247082, 10.85617417291294551, 17.06698730000000097 ) ) ;
#20346=CARTESIAN_POINT ( 'NONE',  ( 67.80000000109247082, 12.06698730000000275, 14.14382582708705094 ) ) ;
#20355=CARTESIAN_POINT ( 'NONE',  ( -67.90000000109247935, 12.06698729999999919, 15.85617417291294196 ) ) ;
#20358=CARTESIAN_POINT ( 'NONE',  ( -69.40000000109246514, 9.143825827087050939, 12.93301269999999370 ) ) ;
#20369=CARTESIAN_POINT ( 'NONE',  ( -68.10000000109246798, 9.143825827087049163, 17.06698729999999742 ) ) ;
#20371=CARTESIAN_POINT ( 'NONE',  ( 69.20000000109246230, 9.143825827087052716, 12.93301269999999192 ) ) ;
#20372=CARTESIAN_POINT ( 'NONE',  ( -68.70000000109246230, 10.85617417291294551, 12.93301269999999370 ) ) ;
#20373=CARTESIAN_POINT ( 'NONE',  ( 66.09999999999999432, 9.999999999999998224, 17.49999999999999645 ) ) ;
#20380=CARTESIAN_POINT ( 'NONE',  ( 68.64999999999999147, 7.499999999999996447, 16.03553390593273775 ) ) ;
#20385=EDGE_LOOP ( 'NONE', ( #16059, #20096, #18242, #8979 ) ) ;
#20398=( BOUNDED_CURVE ( )  B_SPLINE_CURVE ( 2, ( #2008, #13183, #14995, #16760, #3930, #9349, #15104, #218, #14866 ),
 .UNSPECIFIED., .F., .F. ) 
 B_SPLINE_CURVE_WITH_KNOTS ( ( 3, 2, 2, 2, 3 ),
 ( 0.2500000000000006661, 0.2656250000000005551, 0.2812500000000004441, 0.2968750000000003886, 0.3125000000000002776 ),
 .UNSPECIFIED. ) 
 CURVE ( )  GEOMETRIC_REPRESENTATION_ITEM ( )  RATIONAL_B_SPLINE_CURVE ( ( 0.9999999999999967804, 0.9238795325112899581, 1.000000000000000000, 0.9238795325112867385, 1.000000000000000000, 0.9238795325112867385, 1.000000000000000000, 0.9238795325112854062, 1.000000000000001332 ) ) 
 REPRESENTATION_ITEM ( '' )  );
#20400=CARTESIAN_POINT ( 'NONE',  ( 68.84999999999999432, 8.964466094067258695, 12.49999999999999289 ) ) ;
#20408=CARTESIAN_POINT ( 'NONE',  ( -71.75000000109247367, 8.538419263543524096, 13.53841926354352054 ) ) ;
#20413=CARTESIAN_POINT ( 'NONE',  ( -69.70000000109246230, 9.143825827087049163, 17.06698729999999742 ) ) ;
#20423=CARTESIAN_POINT ( 'NONE',  ( 65.55000000218494449, 7.499999999999995559, 16.03553390593273420 ) ) ;
#20426=CARTESIAN_POINT ( 'NONE',  ( 70.90000000109245093, 7.933012699999995476, 14.14382582708705094 ) ) ;
#20428=ORIENTED_EDGE ( 'NONE', *, *, #19191, .T. ) ;
#20458=FACE_OUTER_BOUND ( 'NONE', #11426, .T. ) ;
#20460=CARTESIAN_POINT ( 'NONE',  ( 71.30000000109247082, 12.06698729999999919, 15.85617417291294196 ) ) ;
#20462=ADVANCED_FACE ( 'NONE', ( #18113 ), #23135, .T. ) ;
#20467=CARTESIAN_POINT ( 'NONE',  ( 71.65000000109246514, 7.933012699999995476, 14.99999999999999645 ) ) ;
#20472=CARTESIAN_POINT ( 'NONE',  ( -71.10000000218494165, 8.232233047033627571, 16.76776695296636532 ) ) ;
#20474=CARTESIAN_POINT ( 'NONE',  ( -67.00000000218494733, 9.999999999999998224, 17.49999999999999645 ) ) ;
#20476=VECTOR ( 'NONE', #11747, 1000.000000000000000 ) ;
#20477=ADVANCED_FACE ( 'NONE', ( #10367 ), #3139, .T. ) ;
#20480=CARTESIAN_POINT ( 'NONE',  ( -68.65000000109247935, 12.06698730000000097, 14.99999999999999645 ) ) ;
#20483=CARTESIAN_POINT ( 'NONE',  ( -70.80000000109245661, 7.933012699999995476, 15.85617417291294196 ) ) ;
#20492=CARTESIAN_POINT ( 'NONE',  ( -67.60000000109248219, 9.143825827087050939, 12.93301269999999370 ) ) ;
#20493=CARTESIAN_POINT ( 'NONE',  ( 70.70000000109247651, 7.933012699999995476, 14.14382582708705094 ) ) ;
#20494=CARTESIAN_POINT ( 'NONE',  ( -66.85000000109246798, 7.933012699999995476, 14.99999999999999645 ) ) ;
#20507=ORIENTED_EDGE ( 'NONE', *, *, #18553, .F. ) ;
#20518=CARTESIAN_POINT ( 'NONE',  ( -71.20000000218495018, 7.499999999999996447, 14.99999999999999645 ) ) ;
#20520=CARTESIAN_POINT ( 'NONE',  ( 69.95000000000000284, 12.50000000000000000, 16.03553390593273420 ) ) ;
#20528=CARTESIAN_POINT ( 'NONE',  ( 68.65000000218495302, 8.964466094067214286, 17.49999999999996092 ) ) ;
#20529=CARTESIAN_POINT ( 'NONE',  ( -70.50000000109247367, 12.06698729999999919, 15.85617417291294196 ) ) ;
#20535=CARTESIAN_POINT ( 'NONE',  ( -70.50000000109247367, 9.143825827087049163, 17.06698729999999742 ) ) ;
#20548=CARTESIAN_POINT ( 'NONE',  ( 70.30000000109248504, 12.06698730000000275, 15.85617417291294196 ) ) ;
#20559=VECTOR ( 'NONE', #11580, 1000.000000000000000 ) ;
#20562=ORIENTED_EDGE ( 'NONE', *, *, #7341, .T. ) ;
#20570=ORIENTED_EDGE ( 'NONE', *, *, #14039, .F. ) ;
#20583=CARTESIAN_POINT ( 'NONE',  ( 69.50000000109245946, 10.85617417291294551, 12.93301269999999192 ) ) ;
#20585=EDGE_LOOP ( 'NONE', ( #11578, #23677, #5755, #13005 ) ) ;
#20588=CARTESIAN_POINT ( 'NONE',  ( 67.40000000109247935, 7.933012699999995476, 15.85617417291294196 ) ) ;
#20598=CARTESIAN_POINT ( 'NONE',  ( -67.15000000109247935, 11.46158073645647235, 16.46158073645647235 ) ) ;
#20601=CARTESIAN_POINT ( 'NONE',  ( -70.60000000109246798, 10.85617417291294551, 17.06698729999999742 ) ) ;
#20611=CARTESIAN_POINT ( 'NONE',  ( -68.35000000109248219, 8.538419263543524096, 13.53841926354352054 ) ) ;
#20613=CARTESIAN_POINT ( 'NONE',  ( 67.60000000109248219, 9.143825827087052716, 12.93301269999999192 ) ) ;
#20614=EDGE_CURVE ( 'NONE', #21869, #735, #12754, .T. ) ;
#20617=CARTESIAN_POINT ( 'NONE',  ( -67.45000000109246230, 9.999999999999998224, 17.06698730000000097 ) ) ;
#20618=FACE_OUTER_BOUND ( 'NONE', #21256, .T. ) ;
#20641=CARTESIAN_POINT ( 'NONE',  ( -70.65000000218496723, 11.03553390593273598, 12.49999999999999289 ) ) ;
#20648=CARTESIAN_POINT ( 'NONE',  ( 67.89999999999999147, 7.499999999999996447, 14.99999999999999645 ) ) ;
#20651=CARTESIAN_POINT ( 'NONE',  ( -67.04999999999999716, 7.499999999999996447, 16.03553390593273775 ) ) ;
#20662=CARTESIAN_POINT ( 'NONE',  ( -69.90000000109247935, 7.933012699999995476, 14.14382582708705094 ) ) ;
#20667=EDGE_LOOP ( 'NONE', ( #10401, #3969, #4322, #6962 ) ) ;
#20671=CARTESIAN_POINT ( 'NONE',  ( 69.10000000109248219, 7.933012699999995476, 14.14382582708705094 ) ) ;
#20683=CARTESIAN_POINT ( 'NONE',  ( -66.95000000109246230, 8.538419263543524096, 13.53841926354352054 ) ) ;
#20685=CYLINDRICAL_SURFACE ( 'NONE', #21393, 2.500000000000002220 ) ;
#20690=CARTESIAN_POINT ( 'NONE',  ( 69.15000000218495302, 12.50000000000000000, 13.96446609406725692 ) ) ;
#20695=CYLINDRICAL_SURFACE ( 'NONE', #2615, 2.500000000000002220 ) ;
#20701=( LENGTH_UNIT ( ) NAMED_UNIT ( * ) SI_UNIT ( .MILLI., .METRE. ) );
#20702=CARTESIAN_POINT ( 'NONE',  ( 69.25000000109245946, 7.933012699999995476, 14.99999999999999645 ) ) ;
#20707=CARTESIAN_POINT ( 'NONE',  ( 70.20000000109246230, 9.143825827087050939, 12.93301269999999370 ) ) ;
#20717=CARTESIAN_POINT ( 'NONE',  ( -65.95000000109247651, 8.538419263543524096, 13.53841926354352054 ) ) ;
#20720=CARTESIAN_POINT ( 'NONE',  ( -67.00000000109247367, 9.143825827087050939, 12.93301269999999370 ) ) ;
#20728=CARTESIAN_POINT ( 'NONE',  ( -67.90000000109246514, 12.06698730000000275, 15.85617417291294196 ) ) ;
#20729=CARTESIAN_POINT ( 'NONE',  ( 70.40000000109249356, 10.85617417291294551, 17.06698730000000097 ) ) ;
#20730=CARTESIAN_POINT ( 'NONE',  ( -72.20000000000000284, 11.76776695296636888, 13.23223304703362579 ) ) ;
#20759=CARTESIAN_POINT ( 'NONE',  ( 68.60000000109248219, 12.06698730000000275, 14.14382582708705094 ) ) ;
#20768=CARTESIAN_POINT ( 'NONE',  ( -72.00000000000000000, 8.232233047033629347, 13.23223304703362402 ) ) ;
#20769=CARTESIAN_POINT ( 'NONE',  ( -70.60000000109246798, 10.85617417291294551, 17.06698730000000097 ) ) ;
#20772=ORIENTED_EDGE ( 'NONE', *, *, #8180, .F. ) ;
#20774=CARTESIAN_POINT ( 'NONE',  ( -69.75000000109247367, 8.538419263543522320, 16.46158073645647235 ) ) ;
#20775=EDGE_CURVE ( 'NONE', #14210, #9234, #17507, .T. ) ;
#20784=CARTESIAN_POINT ( 'NONE',  ( 68.90000000109247935, 9.143825827087049163, 17.06698729999999742 ) ) ;
#20785=CARTESIAN_POINT ( 'NONE',  ( 67.75000000109245946, 8.538419263543524096, 13.53841926354352054 ) ) ;
#20804=CARTESIAN_POINT ( 'NONE',  ( -69.40000000218495302, 9.999999999999998224, 17.49999999999999645 ) ) ;
#20810=CARTESIAN_POINT ( 'NONE',  ( 70.85000000109246798, 9.999999999999998224, 12.93301269999999192 ) ) ;
#20816=CARTESIAN_POINT ( 'NONE',  ( 70.15000000109246514, 8.538419263543524096, 13.53841926354352054 ) ) ;
#20818=DIRECTION ( 'NONE',  ( -1.000000000000000000, -0.000000000000000000, -0.000000000000000000 ) ) ;
#20820=CARTESIAN_POINT ( 'NONE',  ( 68.45000000109247651, 7.933012699999995476, 14.99999999999999645 ) ) ;
#20828=CARTESIAN_POINT ( 'NONE',  ( 69.40000000218495302, 9.999999999999998224, 17.49999999999999645 ) ) ;
#20831=EDGE_CURVE ( 'NONE', #9234, #4247, #9856, .T. ) ;
#20833=CARTESIAN_POINT ( 'NONE',  ( -66.00000000109247367, 9.143825827087052716, 12.93301269999999192 ) ) ;
#20835=CARTESIAN_POINT ( 'NONE',  ( -68.90000000109246514, 12.06698730000000275, 15.85617417291294196 ) ) ;
#20841=CARTESIAN_POINT ( 'NONE',  ( -65.75000000109245946, 9.999999999999998224, 17.06698730000000097 ) ) ;
#20843=CARTESIAN_POINT ( 'NONE',  ( -68.25000000109247367, 7.933012699999995476, 14.99999999999999645 ) ) ;
#20845=CARTESIAN_POINT ( 'NONE',  ( 69.35000000109248219, 11.46158073645647235, 13.53841926354352232 ) ) ;
#20846=CARTESIAN_POINT ( 'NONE',  ( -66.45000000109246230, 12.06698730000000097, 14.99999999999999645 ) ) ;
#20854=VERTEX_POINT ( 'NONE', #11552 ) ;
#20867=CARTESIAN_POINT ( 'NONE',  ( -69.00000000218494733, 9.999999999999998224, 12.49999999999999289 ) ) ;
#20870=CARTESIAN_POINT ( 'NONE',  ( 66.24999999999998579, 7.499999999999995559, 16.03553390593273420 ) ) ;
#20873=CARTESIAN_POINT ( 'NONE',  ( 70.85000000109246798, 9.999999999999998224, 12.93301269999999192 ) ) ;
#20879=CARTESIAN_POINT ( 'NONE',  ( -68.70000000109247651, 10.85617417291294551, 12.93301269999999192 ) ) ;
#20880=CARTESIAN_POINT ( 'NONE',  ( -69.85000000218497007, 11.03553390593272177, 12.49999999999998046 ) ) ;
#20884=( BOUNDED_CURVE ( )  B_SPLINE_CURVE ( 2, ( #6343, #4534, #17712, #10546, #5235, #4885, #16037, #19254, #19364 ),
 .UNSPECIFIED., .F., .F. ) 
 B_SPLINE_CURVE_WITH_KNOTS ( ( 3, 2, 2, 2, 3 ),
 ( 0.4999999999999991118, 0.5156249999999995559, 0.5312500000000000000, 0.5468750000000004441, 0.5625000000000008882 ),
 .UNSPECIFIED. ) 
 CURVE ( )  GEOMETRIC_REPRESENTATION_ITEM ( )  RATIONAL_B_SPLINE_CURVE ( ( 1.000000000000004219, 0.9238795325112824086, 1.000000000000000000, 0.9238795325112867385, 1.000000000000000000, 0.9238795325112867385, 1.000000000000000000, 0.9238795325112824086, 1.000000000000004219 ) ) 
 REPRESENTATION_ITEM ( '' )  );
#20893=EDGE_CURVE ( 'NONE', #19953, #4600, #17695, .T. ) ;
#20894=CARTESIAN_POINT ( 'NONE',  ( 67.05000000109247082, 12.06698730000000097, 14.99999999999999645 ) ) ;
#20895=CARTESIAN_POINT ( 'NONE',  ( 67.50000000109245946, 9.143825827087049163, 17.06698729999999742 ) ) ;
#20909=CARTESIAN_POINT ( 'NONE',  ( -70.59999999999999432, 11.76776695296636888, 13.23223304703362579 ) ) ;
#20921=CARTESIAN_POINT ( 'NONE',  ( -69.80000000218494449, 9.999999999999998224, 12.49999999999999289 ) ) ;
#20922=CARTESIAN_POINT ( 'NONE',  ( 70.65000000218496723, 11.03553390593273598, 12.49999999999999289 ) ) ;
#20925=CARTESIAN_POINT ( 'NONE',  ( 66.45000000109246230, 12.06698730000000097, 14.99999999999999645 ) ) ;
#20927=ORIENTED_EDGE ( 'NONE', *, *, #20061, .F. ) ;
#20933=CARTESIAN_POINT ( 'NONE',  ( 71.15000000109246514, 11.46158073645647235, 13.53841926354352232 ) ) ;
#20939=DIRECTION ( 'NONE',  ( -1.000000000000000000, -0.000000000000000000, -0.000000000000000000 ) ) ;
#20946=CARTESIAN_POINT ( 'NONE',  ( -68.50000000109245946, 7.933012699999995476, 14.14382582708705094 ) ) ;
#20955=CARTESIAN_POINT ( 'NONE',  ( 66.80000000109247082, 9.143825827087052716, 12.93301269999999192 ) ) ;
#20959=CARTESIAN_POINT ( 'NONE',  ( -67.80000000109247082, 9.143825827087050939, 12.93301269999999370 ) ) ;
#20960=CARTESIAN_POINT ( 'NONE',  ( -71.34999999999999432, 11.03553390593268269, 12.49999999999994138 ) ) ;
#20985=CARTESIAN_POINT ( 'NONE',  ( -70.55000000218495870, 8.964466094067258695, 12.49999999999999289 ) ) ;
#20992=CARTESIAN_POINT ( 'NONE',  ( 69.65000000109247935, 9.999999999999998224, 17.06698730000000097 ) ) ;
#20999=CARTESIAN_POINT ( 'NONE',  ( -67.75000000109245946, 8.538419263543524096, 13.53841926354352054 ) ) ;
#21002=CARTESIAN_POINT ( 'NONE',  ( -69.74999999999998579, 11.03553390593276262, 12.50000000000001776 ) ) ;
#21015=CARTESIAN_POINT ( 'NONE',  ( 66.90000000109246514, 10.85617417291294551, 12.93301269999999370 ) ) ;
#21018=CARTESIAN_POINT ( 'NONE',  ( 68.85000000109246798, 12.06698730000000097, 14.99999999999999645 ) ) ;
#21021=( BOUNDED_CURVE ( )  B_SPLINE_CURVE ( 2, ( #10190, #3200, #8611, #21265, #12102, #23193, #14251, #6807, #23325 ),
 .UNSPECIFIED., .F., .F. ) 
 B_SPLINE_CURVE_WITH_KNOTS ( ( 3, 2, 2, 2, 3 ),
 ( 0.4374999999999995004, 0.4531249999999993894, 0.4687499999999993339, 0.4843749999999992228, 0.4999999999999991118 ),
 .UNSPECIFIED. ) 
 CURVE ( )  GEOMETRIC_REPRESENTATION_ITEM ( )  RATIONAL_B_SPLINE_CURVE ( ( 1.000000000000002442, 0.9238795325112842960, 1.000000000000000000, 0.9238795325112867385, 1.000000000000000000, 0.9238795325112867385, 1.000000000000000000, 0.9238795325112910684, 0.9999999999999956701 ) ) 
 REPRESENTATION_ITEM ( '' )  );
#21047=CARTESIAN_POINT ( 'NONE',  ( 66.20000000109246230, 9.143825827087052716, 12.93301269999999192 ) ) ;
#21048=ORIENTED_EDGE ( 'NONE', *, *, #14642, .F. ) ;
#21053=CARTESIAN_POINT ( 'NONE',  ( 68.50000000109245946, 7.933012699999995476, 14.14382582708705094 ) ) ;
#21067=CARTESIAN_POINT ( 'NONE',  ( -68.45000000109247651, 7.933012699999995476, 14.99999999999999645 ) ) ;
#21071=DIRECTION ( 'NONE',  ( -0.5000000000000013323, -0.000000000000000000, -0.8660254037844380415 ) ) ;
#21073=EDGE_CURVE ( 'NONE', #22517, #7647, #11274, .T. ) ;
#21079=CARTESIAN_POINT ( 'NONE',  ( 67.35000000109248219, 8.538419263543522320, 16.46158073645647235 ) ) ;
#21080=CARTESIAN_POINT ( 'NONE',  ( -69.95000000000000284, 12.50000000000000000, 16.03553390593273420 ) ) ;
#21081=CARTESIAN_POINT ( 'NONE',  ( -71.70000000000000284, 9.999999999999998224, 17.49999999999999645 ) ) ;
#21088=CARTESIAN_POINT ( 'NONE',  ( 72.50000000000000000, 9.999999999999998224, 14.99999999999999645 ) ) ;
#21091=ORIENTED_EDGE ( 'NONE', *, *, #8067, .T. ) ;
#21102=CARTESIAN_POINT ( 'NONE',  ( -67.65000000218496723, 12.50000000000000000, 16.03553390593273420 ) ) ;
#21108=CARTESIAN_POINT ( 'NONE',  ( 69.75000000109247367, 8.538419263543522320, 16.46158073645647235 ) ) ;
#21112=CARTESIAN_POINT ( 'NONE',  ( 67.75000000218496155, 11.03553390593276617, 17.49999999999997513 ) ) ;
#21115=CARTESIAN_POINT ( 'NONE',  ( -68.95000000109247651, 11.46158073645647235, 16.46158073645647235 ) ) ;
#21124=VERTEX_POINT ( 'NONE', #2132 ) ;
#21126=ORIENTED_EDGE ( 'NONE', *, *, #11102, .T. ) ;
#21129=ORIENTED_EDGE ( 'NONE', *, *, #21216, .F. ) ;
#21131=CARTESIAN_POINT ( 'NONE',  ( 67.15000000109247935, 11.46158073645647235, 16.46158073645647235 ) ) ;
#21133=CARTESIAN_POINT ( 'NONE',  ( 69.55000000109247082, 11.46158073645647235, 13.53841926354352232 ) ) ;
#21135=EDGE_LOOP ( 'NONE', ( #16829, #8347, #1896, #15613 ) ) ;
#21148=CARTESIAN_POINT ( 'NONE',  ( 71.65000000109247935, 9.999999999999998224, 12.93301269999999192 ) ) ;
#21155=CARTESIAN_POINT ( 'NONE',  ( 70.30000000218494449, 8.232233047033627571, 16.76776695296636532 ) ) ;
#21158=( BOUNDED_CURVE ( )  B_SPLINE_CURVE ( 2, ( #17230, #2361, #9692, #11736, #4638, #22713, #8135, #11972, #16989 ),
 .UNSPECIFIED., .F., .F. ) 
 B_SPLINE_CURVE_WITH_KNOTS ( ( 3, 2, 2, 2, 3 ),
 ( 0.000000000000000000, 0.01562499999999990459, 0.03124999999999980918, 0.04687499999999971551, 0.06249999999999961836 ),
 .UNSPECIFIED. ) 
 CURVE ( )  GEOMETRIC_REPRESENTATION_ITEM ( )  RATIONAL_B_SPLINE_CURVE ( ( 1.000000000000000000, 0.9238795325112867385, 1.000000000000000000, 0.9238795325112867385, 1.000000000000000000, 0.9238795325112867385, 1.000000000000000000, 0.9238795325112886259, 0.9999999999999981126 ) ) 
 REPRESENTATION_ITEM ( '' )  );
#21160=CARTESIAN_POINT ( 'NONE',  ( 68.85000000109246798, 12.06698730000000097, 14.99999999999999645 ) ) ;
#21165=CARTESIAN_POINT ( 'NONE',  ( 69.65000000109246514, 12.06698730000000097, 14.99999999999999645 ) ) ;
#21177=CARTESIAN_POINT ( 'NONE',  ( -69.15000000109246514, 8.538419263543522320, 16.46158073645647235 ) ) ;
#21180=ORIENTED_EDGE ( 'NONE', *, *, #2574, .T. ) ;
#21181=ORIENTED_EDGE ( 'NONE', *, *, #20614, .F. ) ;
#21185=CARTESIAN_POINT ( 'NONE',  ( -68.10000000218495586, 8.232233047033629347, 13.23223304703362402 ) ) ;
#21186=EDGE_CURVE ( 'NONE', #12453, #20172, #6097, .T. ) ;
#21189=CARTESIAN_POINT ( 'NONE',  ( -69.59999999999999432, 8.232233047033629347, 13.23223304703362402 ) ) ;
#21191=CARTESIAN_POINT ( 'NONE',  ( -71.45000000000000284, 12.50000000000000000, 13.96446609406725692 ) ) ;
#21195=( BOUNDED_CURVE ( )  B_SPLINE_CURVE ( 2, ( #9109, #7425, #14735, #5608, #2589, #18889, #17100, #8367, #13413 ),
 .UNSPECIFIED., .F., .F. ) 
 B_SPLINE_CURVE_WITH_KNOTS ( ( 3, 2, 2, 2, 3 ),
 ( 0.7499999999999997780, 0.7656249999999996669, 0.7812499999999995559, 0.7968749999999994449, 0.8124999999999993339 ),
 .UNSPECIFIED. ) 
 CURVE ( )  GEOMETRIC_REPRESENTATION_ITEM ( )  RATIONAL_B_SPLINE_CURVE ( ( 1.000000000000001110, 0.9238795325112856283, 1.000000000000000000, 0.9238795325112867385, 1.000000000000000000, 0.9238795325112867385, 1.000000000000000000, 0.9238795325112899581, 0.9999999999999967804 ) ) 
 REPRESENTATION_ITEM ( '' )  );
#21202=CARTESIAN_POINT ( 'NONE',  ( -71.75000000109248788, 11.46158073645647235, 13.53841926354352232 ) ) ;
#21205=CARTESIAN_POINT ( 'NONE',  ( -69.95000000109247651, 8.538419263543524096, 13.53841926354352054 ) ) ;
#21215=CARTESIAN_POINT ( 'NONE',  ( -66.15000000218495302, 11.03553390593273598, 17.50000000000000355 ) ) ;
#21216=EDGE_CURVE ( 'NONE', #18117, #11987, #13431, .T. ) ;
#21222=CARTESIAN_POINT ( 'NONE',  ( 68.25000000109247367, 7.933012699999995476, 14.99999999999999645 ) ) ;
#21223=ADVANCED_FACE ( 'NONE', ( #9826 ), #20695, .T. ) ;
#21229=CARTESIAN_POINT ( 'NONE',  ( 67.60000000218495586, 12.50000000000000000, 14.99999999999999645 ) ) ;
#21231=CARTESIAN_POINT ( 'NONE',  ( -69.30000000109247082, 7.933012699999995476, 14.14382582708705094 ) ) ;
#21247=CARTESIAN_POINT ( 'NONE',  ( 69.05000000109247082, 9.999999999999998224, 17.06698730000000097 ) ) ;
#21256=EDGE_LOOP ( 'NONE', ( #10404, #16328, #9588, #1802 ) ) ;
#21262=CARTESIAN_POINT ( 'NONE',  ( 72.00000000109248788, 10.85617417291294551, 17.06698729999999742 ) ) ;
#21265=CARTESIAN_POINT ( 'NONE',  ( -69.54999999999999716, 7.499999999999996447, 13.96446609406725514 ) ) ;
#21266=ORIENTED_EDGE ( 'NONE', *, *, #3000, .F. ) ;
#21268=CARTESIAN_POINT ( 'NONE',  ( 71.30000000218494449, 8.232233047033629347, 13.23223304703362402 ) ) ;
#21272=CARTESIAN_POINT ( 'NONE',  ( 67.60000000109246798, 7.933012699999995476, 15.85617417291294196 ) ) ;
#21274=CARTESIAN_POINT ( 'NONE',  ( -68.60000000218495586, 9.999999999999998224, 17.49999999999999645 ) ) ;
#21285=CARTESIAN_POINT ( 'NONE',  ( 66.54999999999999716, 11.03553390593269867, 12.49999999999995559 ) ) ;
#21295=( BOUNDED_CURVE ( )  B_SPLINE_CURVE ( 2, ( #21081, #4806, #17402, #9748, #2768, #21191, #19184, #20960, #17518 ),
 .UNSPECIFIED., .F., .F. ) 
 B_SPLINE_CURVE_WITH_KNOTS ( ( 3, 2, 2, 2, 3 ),
 ( 0.1249999999999992367, 0.1406249999999996947, 0.1562500000000001388, 0.1718750000000005829, 0.1875000000000010270 ),
 .UNSPECIFIED. ) 
 CURVE ( )  GEOMETRIC_REPRESENTATION_ITEM ( )  RATIONAL_B_SPLINE_CURVE ( ( 1.000000000000003775, 0.9238795325112830747, 1.000000000000000000, 0.9238795325112867385, 1.000000000000000000, 0.9238795325112867385, 1.000000000000000000, 0.9238795325112817425, 1.000000000000005107 ) ) 
 REPRESENTATION_ITEM ( '' )  );
#21305=CARTESIAN_POINT ( 'NONE',  ( -68.89999999999999147, 9.999999999999998224, 12.49999999999999289 ) ) ;
#21314=VECTOR ( 'NONE', #11581, 999.9999999999997726 ) ;
#21321=CARTESIAN_POINT ( 'NONE',  ( -66.00000000109247367, 9.143825827087050939, 12.93301269999999370 ) ) ;
#21325=ORIENTED_EDGE ( 'NONE', *, *, #8429, .F. ) ;
#21331=EDGE_CURVE ( 'NONE', #22910, #4760, #20884, .T. ) ;
#21334=CARTESIAN_POINT ( 'NONE',  ( -66.05000000218494449, 12.50000000000000000, 16.03553390593273420 ) ) ;
#21337=CARTESIAN_POINT ( 'NONE',  ( -72.25000000109247367, 9.999999999999998224, 17.06698730000000097 ) ) ;
#21355=EDGE_CURVE ( 'NONE', #7935, #23355, #18590, .T. ) ;
#21365=FACE_OUTER_BOUND ( 'NONE', #13924, .T. ) ;
#21370=CARTESIAN_POINT ( 'NONE',  ( 66.35000000109246798, 11.46158073645647235, 13.53841926354352232 ) ) ;
#21377=CARTESIAN_POINT ( 'NONE',  ( 67.95000000218495018, 7.499999999999996447, 16.03553390593273775 ) ) ;
#21388=CARTESIAN_POINT ( 'NONE',  ( 71.90000000109247935, 12.06698730000000275, 15.85617417291294196 ) ) ;
#21389=EDGE_CURVE ( 'NONE', #16036, #20854, #21021, .T. ) ;
#21393=AXIS2_PLACEMENT_3D ( 'NONE', #7892, #4289, #2478 ) ;
#21398=CARTESIAN_POINT ( 'NONE',  ( 68.45000000218493597, 12.50000000000000000, 16.03553390593273420 ) ) ;
#21401=CARTESIAN_POINT ( 'NONE',  ( 67.15000000109247935, 11.46158073645647235, 13.53841926354352232 ) ) ;
#21405=CARTESIAN_POINT ( 'NONE',  ( 68.10000000109245377, 12.06698730000000275, 15.85617417291294196 ) ) ;
#21422=VERTEX_POINT ( 'NONE', #1047 ) ;
#21428=CARTESIAN_POINT ( 'NONE',  ( 65.90000000109247935, 7.933012699999995476, 14.14382582708705094 ) ) ;
#21431=CARTESIAN_POINT ( 'NONE',  ( -69.20000000000000284, 11.76776695296636888, 16.76776695296636532 ) ) ;
#21444=CARTESIAN_POINT ( 'NONE',  ( -66.55000000109247082, 8.538419263543522320, 16.46158073645647235 ) ) ;
#21446=( BOUNDED_CURVE ( )  B_SPLINE_CURVE ( 2, ( #13981, #10161, #23169, #8834, #21599, #6902, #19229, #2818, #17456 ),
 .UNSPECIFIED., .F., .F. ) 
 B_SPLINE_CURVE_WITH_KNOTS ( ( 3, 2, 2, 2, 3 ),
 ( 0.8749999999999990008, 0.8906249999999994449, 0.9062499999999998890, 0.9218750000000003331, 0.9375000000000007772 ),
 .UNSPECIFIED. ) 
 CURVE ( )  GEOMETRIC_REPRESENTATION_ITEM ( )  RATIONAL_B_SPLINE_CURVE ( ( 1.000000000000004885, 0.9238795325112818535, 1.000000000000000000, 0.9238795325112867385, 1.000000000000000000, 0.9238795325112867385, 1.000000000000000000, 0.9238795325112829637, 1.000000000000003775 ) ) 
 REPRESENTATION_ITEM ( '' )  );
#21449=DIRECTION ( 'NONE',  ( 0.000000000000000000, 0.000000000000000000, 1.000000000000000000 ) ) ;
#21454=CARTESIAN_POINT ( 'NONE',  ( -68.75000000218496155, 7.499999999999995559, 16.03553390593273420 ) ) ;
#21460=DIRECTION ( 'NONE',  ( -1.000000000000000000, -0.000000000000000000, -0.000000000000000000 ) ) ;
#21467=CARTESIAN_POINT ( 'NONE',  ( 70.25000000218493312, 8.964466094067294222, 17.50000000000003908 ) ) ;
#21484=CARTESIAN_POINT ( 'NONE',  ( 65.90000000109246514, 7.933012699999995476, 14.14382582708705094 ) ) ;
#21486=CARTESIAN_POINT ( 'NONE',  ( 71.59999999999999432, 11.76776695296636888, 16.76776695296636532 ) ) ;
#21494=CARTESIAN_POINT ( 'NONE',  ( 72.50000000000000000, 9.999999999999998224, 14.99999999999999645 ) ) ;
#21506=CARTESIAN_POINT ( 'NONE',  ( 71.80000000109247082, 12.06698730000000275, 14.14382582708705094 ) ) ;
#21508=EDGE_LOOP ( 'NONE', ( #6459, #11732, #13335, #8695 ) ) ;
#21513=CARTESIAN_POINT ( 'NONE',  ( 66.65000000218493881, 11.03553390593273598, 12.49999999999999289 ) ) ;
#21517=CARTESIAN_POINT ( 'NONE',  ( 70.60000000218494165, 9.999999999999998224, 12.49999999999999289 ) ) ;
#21518=ORIENTED_EDGE ( 'NONE', *, *, #14642, .T. ) ;
#21542=ORIENTED_EDGE ( 'NONE', *, *, #22427, .T. ) ;
#21548=CARTESIAN_POINT ( 'NONE',  ( -71.70000000000000284, 9.999999999999998224, 17.49999999999999645 ) ) ;
#21553=CARTESIAN_POINT ( 'NONE',  ( -67.75000000218496155, 11.03553390593276617, 17.49999999999997513 ) ) ;
#21558=CARTESIAN_POINT ( 'NONE',  ( -70.70000000109247651, 7.933012699999995476, 14.14382582708705094 ) ) ;
#21561=CARTESIAN_POINT ( 'NONE',  ( -68.60000000109248219, 12.06698730000000275, 14.14382582708705094 ) ) ;
#21567=CARTESIAN_POINT ( 'NONE',  ( 71.20000000000000284, 8.232233047033629347, 13.23223304703362402 ) ) ;
#21571=CARTESIAN_POINT ( 'NONE',  ( -67.15000000218495302, 7.499999999999995559, 16.03553390593273420 ) ) ;
#21576=FACE_OUTER_BOUND ( 'NONE', #21842, .T. ) ;
#21582=CARTESIAN_POINT ( 'NONE',  ( -68.29999999999999716, 12.50000000000000000, 14.99999999999999645 ) ) ;
#21583=VECTOR ( 'NONE', #9433, 999.9999999999997726 ) ;
#21589=VECTOR ( 'NONE', #10511, 1000.000000000000000 ) ;
#21599=CARTESIAN_POINT ( 'NONE',  ( -66.69999999999998863, 12.50000000000000000, 14.99999999999999645 ) ) ;
#21607=CARTESIAN_POINT ( 'NONE',  ( 71.24999999999998579, 8.964466094067258695, 12.49999999999999289 ) ) ;
#21610=CARTESIAN_POINT ( 'NONE',  ( 69.80000000218494449, 9.999999999999998224, 12.49999999999999289 ) ) ;
#21618=CARTESIAN_POINT ( 'NONE',  ( -70.40000000218495302, 7.499999999999996447, 14.99999999999999645 ) ) ;
#21620=FACE_OUTER_BOUND ( 'NONE', #1983, .T. ) ;
#21624=EDGE_CURVE ( 'NONE', #4004, #7647, #10893, .T. ) ;
#21635=CARTESIAN_POINT ( 'NONE',  ( 69.35000000218495586, 11.03553390593273598, 17.50000000000000355 ) ) ;
#21644=CARTESIAN_POINT ( 'NONE',  ( 66.70000000109246230, 9.143825827087049163, 17.06698729999999742 ) ) ;
#21647=ORIENTED_EDGE ( 'NONE', *, *, #10605, .T. ) ;
#21651=CARTESIAN_POINT ( 'NONE',  ( 66.69999999999998863, 12.50000000000000000, 14.99999999999999645 ) ) ;
#21670=CARTESIAN_POINT ( 'NONE',  ( -67.54999999999999716, 12.50000000000000000, 16.03553390593273420 ) ) ;
#21676=CARTESIAN_POINT ( 'NONE',  ( -66.30000000109247082, 10.85617417291294551, 12.93301269999999192 ) ) ;
#21677=CARTESIAN_POINT ( 'NONE',  ( 67.79999999999999716, 8.232233047033627571, 16.76776695296636532 ) ) ;
#21682=CARTESIAN_POINT ( 'NONE',  ( -72.00000000109248788, 10.85617417291294551, 17.06698730000000097 ) ) ;
#21685=CARTESIAN_POINT ( 'NONE',  ( -68.00000000109247367, 10.85617417291294551, 17.06698729999999742 ) ) ;
#21697=CARTESIAN_POINT ( 'NONE',  ( -71.50000000109248788, 7.933012699999995476, 14.14382582708705094 ) ) ;
#21698=CARTESIAN_POINT ( 'NONE',  ( -69.80000000109247082, 10.85617417291294551, 17.06698729999999742 ) ) ;
#21727=CARTESIAN_POINT ( 'NONE',  ( 66.20000000109247651, 12.06698730000000275, 14.14382582708705094 ) ) ;
#21728=CARTESIAN_POINT ( 'NONE',  ( 70.54999999999999716, 11.03553390593273598, 12.49999999999999289 ) ) ;
#21734=DIRECTION ( 'NONE',  ( -1.000000000000000000, -0.000000000000000000, -0.000000000000000000 ) ) ;
#21753=CARTESIAN_POINT ( 'NONE',  ( 66.85000000218495586, 12.50000000000000000, 16.03553390593273420 ) ) ;
#21757=CARTESIAN_POINT ( 'NONE',  ( -68.54999999999998295, 8.964466094067287116, 17.50000000000002487 ) ) ;
#21767=CARTESIAN_POINT ( 'NONE',  ( 67.35000000109246798, 11.46158073645647235, 16.46158073645647235 ) ) ;
#21768=CARTESIAN_POINT ( 'NONE',  ( -67.84999999999999432, 7.499999999999996447, 16.03553390593273775 ) ) ;
#21775=CARTESIAN_POINT ( 'NONE',  ( -72.39999999999999147, 11.76776695296636888, 16.76776695296636532 ) ) ;
#21788=CARTESIAN_POINT ( 'NONE',  ( -66.34999999999999432, 7.499999999999996447, 13.96446609406725514 ) ) ;
#21796=CARTESIAN_POINT ( 'NONE',  ( -67.45000000000000284, 12.50000000000000000, 13.96446609406725869 ) ) ;
#21803=CARTESIAN_POINT ( 'NONE',  ( -66.80000000109247082, 7.933012699999995476, 15.85617417291294196 ) ) ;
#21809=ORIENTED_EDGE ( 'NONE', *, *, #48, .T. ) ;
#21810=CARTESIAN_POINT ( 'NONE',  ( -68.30000000109247082, 7.933012699999995476, 14.14382582708705094 ) ) ;
#21813=CARTESIAN_POINT ( 'NONE',  ( -69.00000000109247367, 7.933012699999995476, 15.85617417291294196 ) ) ;
#21822=CARTESIAN_POINT ( 'NONE',  ( -69.65000000109247935, 9.999999999999998224, 17.06698730000000097 ) ) ;
#21823=CARTESIAN_POINT ( 'NONE',  ( -70.30000000109248504, 10.85617417291294551, 12.93301269999999370 ) ) ;
#21835=ORIENTED_EDGE ( 'NONE', *, *, #20614, .T. ) ;
#21836=CARTESIAN_POINT ( 'NONE',  ( 70.05000000218494449, 12.50000000000000000, 16.03553390593273775 ) ) ;
#21837=CARTESIAN_POINT ( 'NONE',  ( -70.20000000000000284, 8.232233047033627571, 16.76776695296636532 ) ) ;
#21842=EDGE_LOOP ( 'NONE', ( #8783, #2665, #17538, #12511 ) ) ;
#21849=CARTESIAN_POINT ( 'NONE',  ( 72.14999999999999147, 11.03553390593273598, 12.49999999999999289 ) ) ;
#21851=CARTESIAN_POINT ( 'NONE',  ( 69.34999999999999432, 8.964466094067214286, 17.49999999999996092 ) ) ;
#21860=CARTESIAN_POINT ( 'NONE',  ( 69.29999999999999716, 9.999999999999998224, 17.49999999999999645 ) ) ;
#21865=ORIENTED_EDGE ( 'NONE', *, *, #16675, .F. ) ;
#21869=VERTEX_POINT ( 'NONE', #12313 ) ;
#21872=CARTESIAN_POINT ( 'NONE',  ( 68.25000000218494733, 11.03553390593273598, 12.49999999999999289 ) ) ;
#21874=CARTESIAN_POINT ( 'NONE',  ( -68.70000000000000284, 7.499999999999996447, 14.99999999999999645 ) ) ;
#21882=CARTESIAN_POINT ( 'NONE',  ( 72.09999999999999432, 9.999999999999998224, 12.49999999999999289 ) ) ;
#21904=CARTESIAN_POINT ( 'NONE',  ( -66.94999999999998863, 8.964466094067258695, 17.50000000000000355 ) ) ;
#21906=CARTESIAN_POINT ( 'NONE',  ( 72.00000000109245946, 12.06698730000000275, 14.14382582708705094 ) ) ;
#21914=CARTESIAN_POINT ( 'NONE',  ( -70.15000000109247935, 11.46158073645647235, 13.53841926354352232 ) ) ;
#21917=CARTESIAN_POINT ( 'NONE',  ( -71.05000000109245661, 9.999999999999998224, 12.93301269999999192 ) ) ;
#21927=CARTESIAN_POINT ( 'NONE',  ( -71.10000000109246798, 12.06698730000000275, 15.85617417291294196 ) ) ;
#21931=CARTESIAN_POINT ( 'NONE',  ( -69.95000000109247651, 8.538419263543522320, 16.46158073645647235 ) ) ;
#21932=( BOUNDED_CURVE ( )  B_SPLINE_CURVE ( 2, ( #18020, #23400, #7006, #10747, #1355, #12411, #15994, #21467, #23279 ),
 .UNSPECIFIED., .F., .F. ) 
 B_SPLINE_CURVE_WITH_KNOTS ( ( 3, 2, 2, 2, 3 ),
 ( 0.1875000000000010270, 0.2031250000000009437, 0.2187500000000008327, 0.2343750000000007494, 0.2500000000000006661 ),
 .UNSPECIFIED. ) 
 CURVE ( )  GEOMETRIC_REPRESENTATION_ITEM ( )  RATIONAL_B_SPLINE_CURVE ( ( 0.9999999999999950040, 0.9238795325112917345, 1.000000000000000000, 0.9238795325112867385, 1.000000000000000000, 0.9238795325112867385, 1.000000000000000000, 0.9238795325112835188, 1.000000000000003331 ) ) 
 REPRESENTATION_ITEM ( '' )  );
#21941=CARTESIAN_POINT ( 'NONE',  ( 70.00000000218494733, 12.50000000000000000, 14.99999999999999645 ) ) ;
#21952=CARTESIAN_POINT ( 'NONE',  ( 68.89999999999999147, 9.999999999999998224, 12.49999999999999289 ) ) ;
#21957=CARTESIAN_POINT ( 'NONE',  ( 67.70000000000000284, 9.999999999999998224, 17.49999999999999645 ) ) ;
#21975=DIRECTION ( 'NONE',  ( -1.000000000000000000, -0.000000000000000000, -0.000000000000000000 ) ) ;
#21985=CARTESIAN_POINT ( 'NONE',  ( 71.65000000109247935, 9.999999999999998224, 12.93301269999999192 ) ) ;
#22003=( NAMED_UNIT ( * ) SI_UNIT ( $, .STERADIAN. ) SOLID_ANGLE_UNIT ( ) );
#22014=LINE ( 'NONE', #6993, #9872 ) ;
#22019=CARTESIAN_POINT ( 'NONE',  ( 67.70000000109246230, 10.85617417291294551, 12.93301269999999370 ) ) ;
#22027=CARTESIAN_POINT ( 'NONE',  ( -67.50000000109247367, 7.933012699999995476, 14.14382582708705094 ) ) ;
#22030=CARTESIAN_POINT ( 'NONE',  ( -70.90000000109245093, 7.933012699999995476, 14.14382582708705094 ) ) ;
#22038=CARTESIAN_POINT ( 'NONE',  ( -70.25000000109247367, 12.06698730000000097, 14.99999999999999645 ) ) ;
#22040=CARTESIAN_POINT ( 'NONE',  ( -70.40000000109247935, 12.06698730000000275, 14.14382582708705094 ) ) ;
#22053=CARTESIAN_POINT ( 'NONE',  ( -70.29999999999999716, 7.499999999999996447, 14.99999999999999645 ) ) ;
#22070=CARTESIAN_POINT ( 'NONE',  ( 68.89999999999999147, 9.999999999999998224, 12.49999999999999289 ) ) ;
#22073=CARTESIAN_POINT ( 'NONE',  ( -67.20000000000000284, 8.232233047033629347, 13.23223304703362402 ) ) ;
#22078=CARTESIAN_POINT ( 'NONE',  ( -71.75000000000001421, 8.964466094067221391, 17.49999999999996447 ) ) ;
#22079=LINE ( 'NONE', #18625, #1717 ) ;
#22085=DIRECTION ( 'NONE',  ( 0.000000000000000000, 0.000000000000000000, 1.000000000000000000 ) ) ;
#22086=EDGE_CURVE ( 'NONE', #16067, #11987, #9603, .T. ) ;
#22098=CARTESIAN_POINT ( 'NONE',  ( 70.35000000109248219, 11.46158073645647235, 16.46158073645647235 ) ) ;
#22100=CARTESIAN_POINT ( 'NONE',  ( -72.50000000000000000, 9.999999999999998224, 14.99999999999999645 ) ) ;
#22101=CARTESIAN_POINT ( 'NONE',  ( 70.60000000109246798, 10.85617417291294551, 17.06698729999999742 ) ) ;
#22137=CARTESIAN_POINT ( 'NONE',  ( 69.65000000109246514, 12.06698730000000097, 14.99999999999999645 ) ) ;
#22142=CARTESIAN_POINT ( 'NONE',  ( 66.40000000218495302, 7.499999999999996447, 14.99999999999999645 ) ) ;
#22143=CARTESIAN_POINT ( 'NONE',  ( 65.85000000109248219, 7.933012699999995476, 14.99999999999999645 ) ) ;
#22149=CARTESIAN_POINT ( 'NONE',  ( -71.35000000218497007, 8.964466094067278235, 12.49999999999997691 ) ) ;
#22153=CARTESIAN_POINT ( 'NONE',  ( -69.90000000109247935, 7.933012699999995476, 14.14382582708705094 ) ) ;
#22156=CARTESIAN_POINT ( 'NONE',  ( -71.95000000109247651, 11.46158073645647235, 13.53841926354352232 ) ) ;
#22166=EDGE_CURVE ( 'NONE', #6908, #4668, #18451, .T. ) ;
#22167=CARTESIAN_POINT ( 'NONE',  ( -71.20000000109246230, 10.85617417291294551, 17.06698729999999742 ) ) ;
#22169=CARTESIAN_POINT ( 'NONE',  ( 69.75000000109247367, 8.538419263543522320, 16.46158073645647235 ) ) ;
#22170=CARTESIAN_POINT ( 'NONE',  ( -71.25000000109247367, 12.06698730000000097, 14.99999999999999645 ) ) ;
#22194=CYLINDRICAL_SURFACE ( 'NONE', #22840, 2.500000000000002220 ) ;
#22198=CARTESIAN_POINT ( 'NONE',  ( 67.09999999999999432, 7.499999999999996447, 14.99999999999999645 ) ) ;
#22201=CARTESIAN_POINT ( 'NONE',  ( -67.14999999999999147, 7.499999999999996447, 13.96446609406725514 ) ) ;
#22206=CARTESIAN_POINT ( 'NONE',  ( -70.80000000109245661, 7.933012699999995476, 15.85617417291294196 ) ) ;
#22218=EDGE_LOOP ( 'NONE', ( #14486, #15056, #13010, #20209 ) ) ;
#22224=CARTESIAN_POINT ( 'NONE',  ( 70.90000000109246514, 10.85617417291294551, 12.93301269999999370 ) ) ;
#22244=CARTESIAN_POINT ( 'NONE',  ( 69.05000000218494449, 11.03553390593276262, 12.50000000000001776 ) ) ;
#22257=FILL_AREA_STYLE ('',( #7912 ) ) ;
#22258=CARTESIAN_POINT ( 'NONE',  ( 70.95000000109247651, 8.538419263543524096, 13.53841926354352054 ) ) ;
#22265=CARTESIAN_POINT ( 'NONE',  ( 71.90000000109246514, 10.85617417291294551, 12.93301269999999370 ) ) ;
#22274=CARTESIAN_POINT ( 'NONE',  ( -69.10000000109248219, 7.933012699999995476, 14.14382582708705094 ) ) ;
#22277=CARTESIAN_POINT ( 'NONE',  ( -71.35000000109246798, 11.46158073645647235, 16.46158073645647235 ) ) ;
#22284=CARTESIAN_POINT ( 'NONE',  ( -67.70000000109246230, 10.85617417291294551, 12.93301269999999370 ) ) ;
#22286=CARTESIAN_POINT ( 'NONE',  ( 69.10000000109248219, 7.933012699999995476, 14.14382582708705094 ) ) ;
#22287=ADVANCED_FACE ( 'NONE', ( #23546 ), #7282, .T. ) ;
#22289=CARTESIAN_POINT ( 'NONE',  ( -67.70000000109246230, 7.933012699999995476, 14.14382582708705094 ) ) ;
#22311=ORIENTED_EDGE ( 'NONE', *, *, #2307, .T. ) ;
#22313=CARTESIAN_POINT ( 'NONE',  ( -70.35000000218492744, 7.499999999999995559, 16.03553390593273420 ) ) ;
#22316=CARTESIAN_POINT ( 'NONE',  ( 67.34999999999999432, 11.03553390593273598, 12.49999999999999289 ) ) ;
#22324=CARTESIAN_POINT ( 'NONE',  ( -71.10000000109246798, 10.85617417291294551, 12.93301269999999192 ) ) ;
#22326=CARTESIAN_POINT ( 'NONE',  ( -69.99999999999998579, 11.76776695296636888, 16.76776695296636532 ) ) ;
#22329=CARTESIAN_POINT ( 'NONE',  ( -65.65000000109247935, 9.999999999999998224, 17.06698730000000097 ) ) ;
#22330=CARTESIAN_POINT ( 'NONE',  ( -72.00000000109248788, 10.85617417291294551, 17.06698729999999742 ) ) ;
#22340=CARTESIAN_POINT ( 'NONE',  ( 66.20000000218495018, 9.999999999999998224, 17.49999999999999645 ) ) ;
#22342=CARTESIAN_POINT ( 'NONE',  ( 66.19999999999998863, 8.232233047033627571, 16.76776695296636532 ) ) ;
#22343=CARTESIAN_POINT ( 'NONE',  ( 71.15000000109246514, 11.46158073645647235, 13.53841926354352232 ) ) ;
#22345=ORIENTED_EDGE ( 'NONE', *, *, #4663, .T. ) ;
#22355=ORIENTED_EDGE ( 'NONE', *, *, #8478, .F. ) ;
#22364=AXIS2_PLACEMENT_3D ( 'NONE', #20051, #7752, #16718 ) ;
#22376=CARTESIAN_POINT ( 'NONE',  ( 71.85000000109246798, 9.999999999999998224, 12.93301269999999192 ) ) ;
#22377=ORIENTED_EDGE ( 'NONE', *, *, #22832, .F. ) ;
#22383=CARTESIAN_POINT ( 'NONE',  ( 66.20000000109247651, 12.06698730000000275, 14.14382582708705094 ) ) ;
#22388=EDGE_CURVE ( 'NONE', #4037, #21869, #14493, .T. ) ;
#22391=CARTESIAN_POINT ( 'NONE',  ( -67.30000000218494449, 8.232233047033629347, 13.23223304703362402 ) ) ;
#22395=CARTESIAN_POINT ( 'NONE',  ( -66.10000000109248219, 10.85617417291294551, 12.93301269999999192 ) ) ;
#22398=CARTESIAN_POINT ( 'NONE',  ( -70.70000000109247651, 9.143825827087049163, 17.06698729999999742 ) ) ;
#22408=CARTESIAN_POINT ( 'NONE',  ( -67.30000000109247082, 9.143825827087049163, 17.06698729999999742 ) ) ;
#22409=CARTESIAN_POINT ( 'NONE',  ( 70.05000000109247082, 9.999999999999998224, 12.93301269999999192 ) ) ;
#22410=CARTESIAN_POINT ( 'NONE',  ( -66.50000000109245946, 12.06698730000000275, 15.85617417291294196 ) ) ;
#22423=EDGE_CURVE ( 'NONE', #433, #1904, #19497, .T. ) ;
#22427=EDGE_CURVE ( 'NONE', #9951, #7519, #1301, .T. ) ;
#22428=CARTESIAN_POINT ( 'NONE',  ( 72.50000000000000000, 9.999999999999998224, 12.49999999999999289 ) ) ;
#22432=CARTESIAN_POINT ( 'NONE',  ( -70.45000000218493597, 7.499999999999995559, 13.96446609406725692 ) ) ;
#22435=CARTESIAN_POINT ( 'NONE',  ( 68.05000000000002558, 8.964466094067258695, 12.49999999999999289 ) ) ;
#22436=CARTESIAN_POINT ( 'NONE',  ( -71.04999999999999716, 7.499999999999996447, 16.03553390593273775 ) ) ;
#22444=CARTESIAN_POINT ( 'NONE',  ( -70.40000000109247935, 12.06698729999999919, 14.14382582708705094 ) ) ;
#22445=CARTESIAN_POINT ( 'NONE',  ( -70.09999999999999432, 9.999999999999998224, 17.49999999999999645 ) ) ;
#22449=CARTESIAN_POINT ( 'NONE',  ( -70.45000000109247651, 9.999999999999998224, 17.06698730000000097 ) ) ;
#22459=CARTESIAN_POINT ( 'NONE',  ( 65.70000000218495018, 8.232233047033629347, 13.23223304703362402 ) ) ;
#22462=ORIENTED_EDGE ( 'NONE', *, *, #13673, .T. ) ;
#22472=AXIS2_PLACEMENT_3D ( 'NONE', #10019, #17306, #411 ) ;
#22474=CARTESIAN_POINT ( 'NONE',  ( -66.50000000109245946, 12.06698729999999919, 15.85617417291294196 ) ) ;
#22476=CARTESIAN_POINT ( 'NONE',  ( 72.50000000000000000, 9.999999999999998224, 12.49999999999999289 ) ) ;
#22479=CARTESIAN_POINT ( 'NONE',  ( -70.84999999999998010, 11.03553390593276973, 17.49999999999997158 ) ) ;
#22499=CARTESIAN_POINT ( 'NONE',  ( 70.20000000109246230, 9.143825827087052716, 12.93301269999999192 ) ) ;
#22505=CARTESIAN_POINT ( 'NONE',  ( 69.00000000109245946, 10.85617417291294551, 17.06698729999999742 ) ) ;
#22517=VERTEX_POINT ( 'NONE', #22929 ) ;
#22519=CARTESIAN_POINT ( 'NONE',  ( -67.70000000109246230, 7.933012699999995476, 14.14382582708705094 ) ) ;
#22532=CARTESIAN_POINT ( 'NONE',  ( -68.65000000109247935, 12.06698730000000097, 14.99999999999999645 ) ) ;
#22534=CARTESIAN_POINT ( 'NONE',  ( 68.00000000109247367, 10.85617417291294551, 17.06698730000000097 ) ) ;
#22536=CARTESIAN_POINT ( 'NONE',  ( -71.95000000000001705, 7.499999999999995559, 13.96446609406725692 ) ) ;
#22562=CARTESIAN_POINT ( 'NONE',  ( -70.90000000218495302, 11.76776695296636888, 16.76776695296636532 ) ) ;
#22569=EDGE_CURVE ( 'NONE', #18480, #23070, #8062, .T. ) ;
#22572=CARTESIAN_POINT ( 'NONE',  ( 71.05000000109247082, 12.06698730000000097, 14.99999999999999645 ) ) ;
#22580=CARTESIAN_POINT ( 'NONE',  ( -71.05000000109245661, 9.999999999999998224, 12.93301269999999192 ) ) ;
#22584=( BOUNDED_CURVE ( )  B_SPLINE_CURVE ( 2, ( #2338, #15307, #4261, #13144, #9551, #15068, #16848, #2561, #7513, #7861, #20408, #5698, #14955, #18864, #7986, #13032, #3893, #653, #2449, #426, #11229, #9428, #11597, #22324, #22580, #6184, #18503, #2090, #9671, #22206, #17079, #13504, #15184, #20769, #5939, #20529, #11478, #22444, #6057, #13388, #9784, #2808, #8340, #11952, #2695, #15658, #22930, #17558, #6543, #3045, #19103, #10268, #12177, #1123, #10036, #17673, #17324, #889, #2918, #21231, #22688, #6657, #17443, #19220, #8224, #13859, #21115, #8469, #13969, #8115, #19330, #20879, #15542, #11828, #8574, #4619, #15773, #783, #22807, #4732, #15425, #4488, #6300, #13618, #6419, #23045, #4843, #12063, #13734, #19448, #20999, #10393, #10149, #1235, #1008, #2118, #20318, #14538, #9453, #11512, #7779, #2364, #11621, #2476, #5734, #456, #20683, #13173, #3491, #21803, #5285, #4165, #18892, #23608, #9811, #22474, #7890, #17104, #7097, #21676, #19890, #15208, #14414, #12630, #18531, #18784, #13063, #15097, #9697 ),
 .UNSPECIFIED., .F., .F. ) 
 B_SPLINE_CURVE_WITH_KNOTS ( ( 3, 2, 2, 2, 2, 2, 2, 2, 2, 2, 2, 2, 2, 2, 2, 2, 2, 2, 2, 2, 2, 2, 2, 2, 2, 2, 2, 2, 2, 2, 2, 2, 2, 2, 2, 2, 2, 2, 2, 2, 2, 2, 2, 2, 2, 2, 2, 2, 2, 2, 2, 2, 2, 2, 2, 2, 2, 2, 2, 2, 2, 2, 2, 2, 3 ),
 ( 0.000000000000000000, 0.01562500000000000000, 0.03125000000000000000, 0.04687500000000000000, 0.06250000000000000000, 0.07812500000000000000, 0.09375000000000000000, 0.1093750000000000000, 0.1250000000000000000, 0.1406250000000000000, 0.1562500000000000000, 0.1718750000000000000, 0.1875000000000000000, 0.2031250000000000000, 0.2187500000000000000, 0.2343750000000000000, 0.2500000000000000000, 0.2656250000000000000, 0.2812500000000000000, 0.2968750000000000000, 0.3125000000000000000, 0.3281250000000000000, 0.3437500000000000000, 0.3593750000000000000, 0.3750000000000000000, 0.3906250000000000000, 0.4062500000000000000, 0.4218750000000000000, 0.4375000000000000000, 0.4531250000000000000, 0.4687500000000000000, 0.4843750000000000000, 0.5000000000000000000, 0.5156250000000000000, 0.5312500000000000000, 0.5468750000000000000, 0.5625000000000000000, 0.5781250000000000000, 0.5937500000000000000, 0.6093750000000000000, 0.6250000000000000000, 0.6406250000000000000, 0.6562500000000000000, 0.6718750000000000000, 0.6875000000000000000, 0.7031250000000000000, 0.7187500000000000000, 0.7343750000000000000, 0.7500000000000000000, 0.7656250000000000000, 0.7812500000000000000, 0.7968750000000000000, 0.8125000000000000000, 0.8281250000000000000, 0.8437500000000000000, 0.8593750000000000000, 0.8750000000000000000, 0.8906250000000000000, 0.9062500000000000000, 0.9218750000000000000, 0.9375000000000000000, 0.9531250000000000000, 0.9687500000000000000, 0.9843750000000000000, 1.000000000000000000 ),
 .UNSPECIFIED. ) 
 CURVE ( )  GEOMETRIC_REPRESENTATION_ITEM ( )  RATIONAL_B_SPLINE_CURVE ( ( 1.000000000000000000, 0.9238795325112867385, 1.000000000000000000, 0.9238795325112867385, 1.000000000000000000, 0.9238795325112867385, 1.000000000000000000, 0.9238795325112867385, 1.000000000000000000, 0.9238795325112867385, 1.000000000000000000, 0.9238795325112867385, 1.000000000000000000, 0.9238795325112867385, 1.000000000000000000, 0.9238795325112867385, 1.000000000000000000, 0.9238795325112867385, 1.000000000000000000, 0.9238795325112867385, 1.000000000000000000, 0.9238795325112867385, 1.000000000000000000, 0.9238795325112867385, 1.000000000000000000, 0.9238795325112867385, 1.000000000000000000, 0.9238795325112867385, 1.000000000000000000, 0.9238795325112867385, 1.000000000000000000, 0.9238795325112867385, 1.000000000000000000, 0.9238795325112867385, 1.000000000000000000, 0.9238795325112867385, 1.000000000000000000, 0.9238795325112867385, 1.000000000000000000, 0.9238795325112867385, 1.000000000000000000, 0.9238795325112867385, 1.000000000000000000, 0.9238795325112867385, 1.000000000000000000, 0.9238795325112867385, 1.000000000000000000, 0.9238795325112867385, 1.000000000000000000, 0.9238795325112867385, 1.000000000000000000, 0.9238795325112867385, 1.000000000000000000, 0.9238795325112867385, 1.000000000000000000, 0.9238795325112867385, 1.000000000000000000, 0.9238795325112867385, 1.000000000000000000, 0.9238795325112867385, 1.000000000000000000, 0.9238795325112867385, 1.000000000000000000, 0.9238795325112867385, 1.000000000000000000, 0.9238795325112867385, 1.000000000000000000, 0.9238795325112867385, 1.000000000000000000, 0.9238795325112867385, 1.000000000000000000, 0.9238795325112867385, 1.000000000000000000, 0.9238795325112867385, 1.000000000000000000, 0.9238795325112867385, 1.000000000000000000, 0.9238795325112867385, 1.000000000000000000, 0.9238795325112867385, 1.000000000000000000, 0.9238795325112867385, 1.000000000000000000, 0.9238795325112867385, 1.000000000000000000, 0.9238795325112867385, 1.000000000000000000, 0.9238795325112867385, 1.000000000000000000, 0.9238795325112867385, 1.000000000000000000, 0.9238795325112867385, 1.000000000000000000, 0.9238795325112867385, 1.000000000000000000, 0.9238795325112867385, 1.000000000000000000, 0.9238795325112867385, 1.000000000000000000, 0.9238795325112867385, 1.000000000000000000, 0.9238795325112867385, 1.000000000000000000, 0.9238795325112867385, 1.000000000000000000, 0.9238795325112867385, 1.000000000000000000, 0.9238795325112867385, 1.000000000000000000, 0.9238795325112867385, 1.000000000000000000, 0.9238795325112867385, 1.000000000000000000, 0.9238795325112867385, 1.000000000000000000, 0.9238795325112867385, 1.000000000000000000, 0.9238795325112867385, 1.000000000000000000, 0.9238795325112867385, 1.000000000000000000, 0.9238795325112867385, 1.000000000000000000, 0.9238795325112867385, 1.000000000000000000, 0.9238795325112867385, 1.000000000000000000, 0.9238795325112867385, 1.000000000000000000 ) ) 
 REPRESENTATION_ITEM ( '' )  );
#22586=CARTESIAN_POINT ( 'NONE',  ( -70.70000000109247651, 7.933012699999995476, 14.14382582708705094 ) ) ;
#22595=CARTESIAN_POINT ( 'NONE',  ( 67.85000000109248219, 12.06698730000000097, 14.99999999999999645 ) ) ;
#22596=CARTESIAN_POINT ( 'NONE',  ( 68.25000000109245946, 9.999999999999998224, 17.06698730000000097 ) ) ;
#22618=CARTESIAN_POINT ( 'NONE',  ( 71.00000000109248788, 12.06698729999999919, 14.14382582708705094 ) ) ;
#22620=CARTESIAN_POINT ( 'NONE',  ( 70.50000000218494733, 8.232233047033629347, 13.23223304703362402 ) ) ;
#22624=SURFACE_STYLE_USAGE ( .BOTH. , #5753 ) ;
#22625=CARTESIAN_POINT ( 'NONE',  ( 72.05000000109245661, 12.06698730000000097, 14.99999999999999645 ) ) ;
#22629=CARTESIAN_POINT ( 'NONE',  ( 71.45000000109247651, 9.999999999999998224, 17.06698730000000097 ) ) ;
#22640=CARTESIAN_POINT ( 'NONE',  ( -66.40000000109247935, 10.85617417291294551, 17.06698730000000097 ) ) ;
#22642=CARTESIAN_POINT ( 'NONE',  ( -66.80000000109247082, 7.933012699999995476, 15.85617417291294196 ) ) ;
#22650=CARTESIAN_POINT ( 'NONE',  ( -69.05000000109247082, 7.933012699999995476, 14.99999999999999645 ) ) ;
#22651=CARTESIAN_POINT ( 'NONE',  ( 68.05000000109247082, 9.999999999999998224, 17.06698730000000097 ) ) ;
#22652=CARTESIAN_POINT ( 'NONE',  ( -71.89999999999999147, 7.499999999999996447, 14.99999999999999645 ) ) ;
#22659=CARTESIAN_POINT ( 'NONE',  ( -72.50000000000000000, 9.999999999999998224, 17.49999999999999645 ) ) ;
#22673=EDGE_CURVE ( 'NONE', #14810, #4086, #21932, .T. ) ;
#22674=CARTESIAN_POINT ( 'NONE',  ( -71.35000000218494165, 8.964466094067258695, 12.49999999999999289 ) ) ;
#22679=CARTESIAN_POINT ( 'NONE',  ( 69.90000000109247935, 7.933012699999995476, 14.14382582708705094 ) ) ;
#22688=CARTESIAN_POINT ( 'NONE',  ( -69.25000000109245946, 7.933012699999995476, 14.99999999999999645 ) ) ;
#22690=CARTESIAN_POINT ( 'NONE',  ( 65.75000000218494733, 8.964466094067219615, 12.50000000000003553 ) ) ;
#22693=DIRECTION ( 'NONE',  ( 0.000000000000000000, 0.000000000000000000, 1.000000000000000000 ) ) ;
#22695=AXIS2_PLACEMENT_3D ( 'NONE', #71, #18275, #1860 ) ;
#22706=CARTESIAN_POINT ( 'NONE',  ( 69.85000000109248219, 7.933012699999995476, 14.99999999999999645 ) ) ;
#22707=CARTESIAN_POINT ( 'NONE',  ( 69.75000000109245946, 11.46158073645647235, 16.46158073645647235 ) ) ;
#22708=PRODUCT_DEFINITION_SHAPE ( 'NONE', 'NONE',  #3726 ) ;
#22713=CARTESIAN_POINT ( 'NONE',  ( 71.55000000218494449, 12.50000000000000000, 13.96446609406725692 ) ) ;
#22728=CARTESIAN_POINT ( 'NONE',  ( -70.90000000218495302, 11.76776695296636888, 16.76776695296636532 ) ) ;
#22735=DIRECTION ( 'NONE',  ( -1.000000000000000000, 0.000000000000000000, 0.000000000000000000 ) ) ;
#22736=CARTESIAN_POINT ( 'NONE',  ( 70.25000000218494733, 8.964466094067258695, 17.50000000000000355 ) ) ;
#22739=CARTESIAN_POINT ( 'NONE',  ( 67.55000000109247082, 8.538419263543522320, 16.46158073645647235 ) ) ;
#22743=CARTESIAN_POINT ( 'NONE',  ( 69.30000000109247082, 7.933012699999995476, 14.14382582708705094 ) ) ;
#22756=ORIENTED_EDGE ( 'NONE', *, *, #985, .T. ) ;
#22757=CARTESIAN_POINT ( 'NONE',  ( -69.10000000109246798, 9.143825827087049163, 17.06698729999999742 ) ) ;
#22765=CARTESIAN_POINT ( 'NONE',  ( -68.00000000109247367, 10.85617417291294551, 17.06698729999999742 ) ) ;
#22767=CARTESIAN_POINT ( 'NONE',  ( 65.85000000109248219, 7.933012699999995476, 14.99999999999999645 ) ) ;
#22769=CARTESIAN_POINT ( 'NONE',  ( -67.10000000109246798, 10.85617417291294551, 12.93301269999999370 ) ) ;
#22786=ORIENTED_EDGE ( 'NONE', *, *, #1612, .F. ) ;
#22787=CYLINDRICAL_SURFACE ( 'NONE', #2593, 2.500000000000002220 ) ;
#22791=ORIENTED_EDGE ( 'NONE', *, *, #8067, .F. ) ;
#22793=CARTESIAN_POINT ( 'NONE',  ( -69.45000000218493597, 8.964466094067258695, 17.50000000000000355 ) ) ;
#22795=EDGE_CURVE ( 'NONE', #5860, #13392, #10516, .T. ) ;
#22797=CARTESIAN_POINT ( 'NONE',  ( 66.09999999999999432, 9.999999999999998224, 17.49999999999999645 ) ) ;
#22799=CARTESIAN_POINT ( 'NONE',  ( -71.20000000000000284, 8.232233047033629347, 13.23223304703362402 ) ) ;
#22800=CARTESIAN_POINT ( 'NONE',  ( 69.35000000109248219, 11.46158073645647235, 13.53841926354352232 ) ) ;
#22807=CARTESIAN_POINT ( 'NONE',  ( -68.35000000109246798, 8.538419263543522320, 16.46158073645647235 ) ) ;
#22809=CARTESIAN_POINT ( 'NONE',  ( 65.50000000218494733, 8.232233047033627571, 16.76776695296636532 ) ) ;
#22820=CARTESIAN_POINT ( 'NONE',  ( 69.15000000109247935, 8.538419263543524096, 13.53841926354352054 ) ) ;
#22821=AXIS2_PLACEMENT_3D ( 'NONE', #8316, #10373, #3144 ) ;
#22822=CARTESIAN_POINT ( 'NONE',  ( 67.00000000109247367, 9.143825827087050939, 12.93301269999999370 ) ) ;
#22831=CARTESIAN_POINT ( 'NONE',  ( 68.10000000218495586, 8.232233047033629347, 13.23223304703362402 ) ) ;
#22832=EDGE_CURVE ( 'NONE', #11622, #735, #16929, .T. ) ;
#22840=AXIS2_PLACEMENT_3D ( 'NONE', #4005, #11344, #20041 ) ;
#22845=CARTESIAN_POINT ( 'NONE',  ( -70.75000000218496155, 12.50000000000000000, 13.96446609406725692 ) ) ;
#22849=CARTESIAN_POINT ( 'NONE',  ( 71.70000000109247651, 10.85617417291294551, 12.93301269999999192 ) ) ;
#22850=CARTESIAN_POINT ( 'NONE',  ( 71.65000000218496723, 12.50000000000000000, 16.03553390593273420 ) ) ;
#22852=CARTESIAN_POINT ( 'NONE',  ( 72.50000000000000000, 9.999999999999998224, 12.49999999999999289 ) ) ;
#22855=CARTESIAN_POINT ( 'NONE',  ( 66.25000000109245946, 9.999999999999998224, 12.93301269999999192 ) ) ;
#22861=CARTESIAN_POINT ( 'NONE',  ( 69.10000000109246798, 9.143825827087049163, 17.06698729999999742 ) ) ;
#22875=CARTESIAN_POINT ( 'NONE',  ( -66.75000000109245946, 8.538419263543522320, 16.46158073645647235 ) ) ;
#22889=CARTESIAN_POINT ( 'NONE',  ( -71.05000000000001137, 7.499999999999995559, 16.03553390593273420 ) ) ;
#22893=( BOUNDED_CURVE ( )  B_SPLINE_CURVE ( 2, ( #14293, #17989, #3249, #9026, #19891, #19996, #21677, #7346, #19767 ),
 .UNSPECIFIED., .F., .F. ) 
 B_SPLINE_CURVE_WITH_KNOTS ( ( 3, 2, 2, 2, 3 ),
 ( 0.6875000000000001110, 0.7031250000000000000, 0.7187500000000000000, 0.7343749999999998890, 0.7499999999999997780 ),
 .UNSPECIFIED. ) 
 CURVE ( )  GEOMETRIC_REPRESENTATION_ITEM ( )  RATIONAL_B_SPLINE_CURVE ( ( 0.9999999999999994449, 0.9238795325112872936, 1.000000000000000000, 0.9238795325112867385, 1.000000000000000000, 0.9238795325112867385, 1.000000000000000000, 0.9238795325112878487, 0.9999999999999988898 ) ) 
 REPRESENTATION_ITEM ( '' )  );
#22896=CARTESIAN_POINT ( 'NONE',  ( 71.59999999999999432, 11.76776695296636888, 16.76776695296636532 ) ) ;
#22910=VERTEX_POINT ( 'NONE', #17526 ) ;
#22915=CARTESIAN_POINT ( 'NONE',  ( -68.05000000218494449, 7.499999999999995559, 13.96446609406725692 ) ) ;
#22919=CARTESIAN_POINT ( 'NONE',  ( 66.19999999999998863, 8.232233047033627571, 16.76776695296636532 ) ) ;
#22923=CARTESIAN_POINT ( 'NONE',  ( 69.05000000109247082, 7.933012699999995476, 14.99999999999999645 ) ) ;
#22929=CARTESIAN_POINT ( 'NONE',  ( 70.09999999999999432, 9.999999999999998224, 17.49999999999999645 ) ) ;
#22930=CARTESIAN_POINT ( 'NONE',  ( -69.95000000109247651, 8.538419263543522320, 16.46158073645647235 ) ) ;
#22950=CARTESIAN_POINT ( 'NONE',  ( 69.60000000109249640, 10.85617417291294551, 17.06698729999999742 ) ) ;
#22951=AXIS2_PLACEMENT_3D ( 'NONE', #21088, #15854, #15508 ) ;
#22952=CARTESIAN_POINT ( 'NONE',  ( 66.75000000109245946, 8.538419263543522320, 16.46158073645647235 ) ) ;
#22963=DIRECTION ( 'NONE',  ( 0.5000000000000013323, 0.000000000000000000, 0.8660254037844380415 ) ) ;
#22966=EDGE_CURVE ( 'NONE', #4847, #5505, #15748, .T. ) ;
#22975=CARTESIAN_POINT ( 'NONE',  ( 71.20000000109246230, 10.85617417291294551, 17.06698730000000097 ) ) ;
#22977=CARTESIAN_POINT ( 'NONE',  ( 71.25000000218494733, 7.499999999999995559, 13.96446609406725692 ) ) ;
#22981=CARTESIAN_POINT ( 'NONE',  ( 66.15000000109247935, 8.538419263543524096, 13.53841926354352054 ) ) ;
#22986=CARTESIAN_POINT ( 'NONE',  ( 71.00000000109245946, 9.143825827087050939, 12.93301269999999370 ) ) ;
#22998=CARTESIAN_POINT ( 'NONE',  ( -66.20000000109246230, 9.143825827087050939, 12.93301269999999370 ) ) ;
#23000=ADVANCED_FACE ( 'NONE', ( #11682 ), #19190, .T. ) ;
#23001=VERTEX_POINT ( 'NONE', #751 ) ;
#23004=( BOUNDED_CURVE ( )  B_SPLINE_CURVE ( 2, ( #1267, #14358, #3191, #5352, #19950, #23554, #14120, #19711, #4876 ),
 .UNSPECIFIED., .F., .F. ) 
 B_SPLINE_CURVE_WITH_KNOTS ( ( 3, 2, 2, 2, 3 ),
 ( 0.6250000000000005551, 0.6406250000000004441, 0.6562500000000003331, 0.6718750000000002220, 0.6875000000000001110 ),
 .UNSPECIFIED. ) 
 CURVE ( )  GEOMETRIC_REPRESENTATION_ITEM ( )  RATIONAL_B_SPLINE_CURVE ( ( 0.9999999999999973355, 0.9238795325112894030, 1.000000000000000000, 0.9238795325112867385, 1.000000000000000000, 0.9238795325112867385, 1.000000000000000000, 0.9238795325112861834, 1.000000000000000444 ) ) 
 REPRESENTATION_ITEM ( '' )  );
#23010=CARTESIAN_POINT ( 'NONE',  ( 66.50000000109247367, 9.143825827087049163, 17.06698730000000097 ) ) ;
#23011=CARTESIAN_POINT ( 'NONE',  ( -69.70000000000000284, 9.999999999999998224, 12.49999999999999289 ) ) ;
#23017=DIRECTION ( 'NONE',  ( -1.000000000000000000, -0.000000000000000000, -0.000000000000000000 ) ) ;
#23024=CARTESIAN_POINT ( 'NONE',  ( -69.35000000109248219, 11.46158073645647235, 13.53841926354352232 ) ) ;
#23030=ORIENTED_EDGE ( 'NONE', *, *, #4398, .F. ) ;
#23033=CARTESIAN_POINT ( 'NONE',  ( -66.30000000218494449, 8.232233047033627571, 16.76776695296636532 ) ) ;
#23039=CARTESIAN_POINT ( 'NONE',  ( 68.40000000109249356, 9.143825827087050939, 12.93301269999999370 ) ) ;
#23044=CARTESIAN_POINT ( 'NONE',  ( 67.45000000000000284, 12.50000000000000000, 13.96446609406725692 ) ) ;
#23045=CARTESIAN_POINT ( 'NONE',  ( -68.00000000109245946, 12.06698729999999919, 14.14382582708705094 ) ) ;
#23046=VERTEX_POINT ( 'NONE', #22659 ) ;
#23058=CARTESIAN_POINT ( 'NONE',  ( 69.65000000109247935, 9.999999999999998224, 17.06698730000000097 ) ) ;
#23060=CARTESIAN_POINT ( 'NONE',  ( 68.50000000109245946, 7.933012699999995476, 14.14382582708705094 ) ) ;
#23070=VERTEX_POINT ( 'NONE', #12035 ) ;
#23084=CARTESIAN_POINT ( 'NONE',  ( 70.15000000218495302, 11.03553390593273598, 17.50000000000000355 ) ) ;
#23087=CARTESIAN_POINT ( 'NONE',  ( 68.00000000109245946, 12.06698729999999919, 14.14382582708705094 ) ) ;
#23092=CARTESIAN_POINT ( 'NONE',  ( 66.75000000109245946, 8.538419263543522320, 16.46158073645647235 ) ) ;
#23094=DIRECTION ( 'NONE',  ( -1.000000000000000000, -0.000000000000000000, -0.000000000000000000 ) ) ;
#23112=LINE ( 'NONE', #20841, #1157 ) ;
#23115=CARTESIAN_POINT ( 'NONE',  ( 66.70000000109246230, 7.933012699999995476, 14.14382582708705094 ) ) ;
#23118=CARTESIAN_POINT ( 'NONE',  ( -69.39999999999999147, 8.232233047033627571, 16.76776695296636532 ) ) ;
#23133=CARTESIAN_POINT ( 'NONE',  ( -70.30000000109248504, 12.06698730000000275, 15.85617417291294196 ) ) ;
#23135=CYLINDRICAL_SURFACE ( 'NONE', #12474, 2.500000000000002220 ) ;
#23144=CARTESIAN_POINT ( 'NONE',  ( -66.80000000218494449, 12.50000000000000000, 14.99999999999999645 ) ) ;
#23150=CARTESIAN_POINT ( 'NONE',  ( 67.14999999999999147, 7.499999999999996447, 13.96446609406725514 ) ) ;
#23169=CARTESIAN_POINT ( 'NONE',  ( -66.79999999999999716, 11.76776695296636888, 16.76776695296636532 ) ) ;
#23173=CARTESIAN_POINT ( 'NONE',  ( -69.40000000218495302, 9.999999999999998224, 17.49999999999999645 ) ) ;
#23176=CARTESIAN_POINT ( 'NONE',  ( 66.30000000109247082, 10.85617417291294551, 12.93301269999999370 ) ) ;
#23190=CARTESIAN_POINT ( 'NONE',  ( -67.29999999999999716, 9.999999999999998224, 12.49999999999999289 ) ) ;
#23193=CARTESIAN_POINT ( 'NONE',  ( -69.45000000000000284, 7.499999999999996447, 16.03553390593273775 ) ) ;
#23197=CARTESIAN_POINT ( 'NONE',  ( 67.50000000218494733, 11.76776695296636888, 13.23223304703362579 ) ) ;
#23201=CARTESIAN_POINT ( 'NONE',  ( 67.80000000109247082, 9.143825827087052716, 12.93301269999999192 ) ) ;
#23205=CARTESIAN_POINT ( 'NONE',  ( 65.95000000109246230, 8.538419263543522320, 16.46158073645647235 ) ) ;
#23224=EDGE_CURVE ( 'NONE', #18376, #19953, #8679, .T. ) ;
#23231=CARTESIAN_POINT ( 'NONE',  ( -66.85000000218495586, 12.50000000000000000, 16.03553390593273775 ) ) ;
#23232=CARTESIAN_POINT ( 'NONE',  ( 67.45000000109246230, 7.933012699999995476, 14.99999999999999645 ) ) ;
#23235=CARTESIAN_POINT ( 'NONE',  ( -70.89999999999999147, 9.999999999999998224, 17.49999999999999645 ) ) ;
#23240=CARTESIAN_POINT ( 'NONE',  ( -67.80000000218494449, 9.999999999999998224, 17.49999999999999645 ) ) ;
#23250=CARTESIAN_POINT ( 'NONE',  ( -68.75000000109247367, 11.46158073645647235, 16.46158073645647235 ) ) ;
#23264=CARTESIAN_POINT ( 'NONE',  ( -68.30000000218494449, 11.76776695296636888, 13.23223304703362579 ) ) ;
#23277=DIRECTION ( 'NONE',  ( -1.000000000000000000, -0.000000000000000000, -0.000000000000000000 ) ) ;
#23279=CARTESIAN_POINT ( 'NONE',  ( 70.20000000218495018, 9.999999999999998224, 17.49999999999999645 ) ) ;
#23285=LINE ( 'NONE', #8344, #11534 ) ;
#23301=CARTESIAN_POINT ( 'NONE',  ( 66.15000000109247935, 11.46158073645647235, 13.53841926354352232 ) ) ;
#23303=VECTOR ( 'NONE', #13904, 1000.000000000000000 ) ;
#23304=CARTESIAN_POINT ( 'NONE',  ( 71.34999999999999432, 11.03553390593273598, 12.49999999999999289 ) ) ;
#23314=ORIENTED_EDGE ( 'NONE', *, *, #4661, .F. ) ;
#23324=EDGE_LOOP ( 'NONE', ( #8730, #1493, #8352 ) ) ;
#23325=CARTESIAN_POINT ( 'NONE',  ( -69.29999999999999716, 9.999999999999998224, 17.49999999999999645 ) ) ;
#23331=CARTESIAN_POINT ( 'NONE',  ( 67.00000000218494733, 9.999999999999998224, 17.49999999999999645 ) ) ;
#23342=DIRECTION ( 'NONE',  ( 0.000000000000000000, 0.000000000000000000, 1.000000000000000000 ) ) ;
#23348=CARTESIAN_POINT ( 'NONE',  ( 66.79999999999999716, 11.76776695296636888, 16.76776695296636532 ) ) ;
#23351=FACE_OUTER_BOUND ( 'NONE', #5439, .T. ) ;
#23354=( BOUNDED_CURVE ( )  B_SPLINE_CURVE ( 2, ( #20269, #5796, #16695, #7730, #22053, #13124, #21837, #1829, #2187 ),
 .UNSPECIFIED., .F., .F. ) 
 B_SPLINE_CURVE_WITH_KNOTS ( ( 3, 2, 2, 2, 3 ),
 ( 0.3125000000000002776, 0.3281250000000001665, 0.3437500000000001110, 0.3593750000000000000, 0.3749999999999998890 ),
 .UNSPECIFIED. ) 
 CURVE ( )  GEOMETRIC_REPRESENTATION_ITEM ( )  RATIONAL_B_SPLINE_CURVE ( ( 0.9999999999999986677, 0.9238795325112880708, 1.000000000000000000, 0.9238795325112867385, 1.000000000000000000, 0.9238795325112867385, 1.000000000000000000, 0.9238795325112872936, 0.9999999999999994449 ) ) 
 REPRESENTATION_ITEM ( '' )  );
#23355=VERTEX_POINT ( 'NONE', #17 ) ;
#23357=EDGE_LOOP ( 'NONE', ( #20927, #9318, #5420, #17571 ) ) ;
#23366=CARTESIAN_POINT ( 'NONE',  ( -71.24999999999998579, 8.964466094067258695, 12.49999999999999289 ) ) ;
#23376=CARTESIAN_POINT ( 'NONE',  ( -70.85000000109246798, 9.999999999999998224, 12.93301269999999192 ) ) ;
#23379=CARTESIAN_POINT ( 'NONE',  ( -68.20000000109246230, 7.933012699999995476, 15.85617417291294196 ) ) ;
#23381=ADVANCED_FACE ( 'NONE', ( #11545 ), #7348, .T. ) ;
#23389=CARTESIAN_POINT ( 'NONE',  ( -66.75000000218494733, 12.50000000000000000, 13.96446609406725869 ) ) ;
#23400=CARTESIAN_POINT ( 'NONE',  ( 70.55000000218494449, 8.964466094067205404, 12.50000000000004263 ) ) ;
#23408=EDGE_CURVE ( 'NONE', #11987, #9892, #12956, .T. ) ;
#23416=ORIENTED_EDGE ( 'NONE', *, *, #16360, .T. ) ;
#23420=CARTESIAN_POINT ( 'NONE',  ( 72.00000000000000000, 8.232233047033629347, 13.23223304703362402 ) ) ;
#23423=CARTESIAN_POINT ( 'NONE',  ( -65.45000000218495018, 8.964466094067260471, 17.50000000000000355 ) ) ;
#23424=AXIS2_PLACEMENT_3D ( 'NONE', #1208, #8545, #15852 ) ;
#23447=CARTESIAN_POINT ( 'NONE',  ( 69.45000000218493597, 8.964466094067258695, 17.50000000000000355 ) ) ;
#23455=CARTESIAN_POINT ( 'NONE',  ( 66.20000000109246230, 9.143825827087050939, 12.93301269999999370 ) ) ;
#23471=CARTESIAN_POINT ( 'NONE',  ( -66.00000000218494733, 12.50000000000000000, 14.99999999999999645 ) ) ;
#23478=CARTESIAN_POINT ( 'NONE',  ( -66.79999999999999716, 11.76776695296636888, 16.76776695296636532 ) ) ;
#23487=CARTESIAN_POINT ( 'NONE',  ( -66.20000000218495018, 9.999999999999998224, 17.49999999999999645 ) ) ;
#23492=CARTESIAN_POINT ( 'NONE',  ( -66.95000000109246230, 11.46158073645647235, 13.53841926354352232 ) ) ;
#23503=CARTESIAN_POINT ( 'NONE',  ( -70.65000000109247935, 7.933012699999995476, 14.99999999999999645 ) ) ;
#23505=CARTESIAN_POINT ( 'NONE',  ( -71.20000000109246230, 12.06698730000000275, 14.14382582708705094 ) ) ;
#23539=CARTESIAN_POINT ( 'NONE',  ( 71.39999999999999147, 11.76776695296636888, 13.23223304703362579 ) ) ;
#23546=FACE_OUTER_BOUND ( 'NONE', #15995, .T. ) ;
#23552=VERTEX_POINT ( 'NONE', #11773 ) ;
#23554=CARTESIAN_POINT ( 'NONE',  ( 68.24999999999998579, 12.50000000000000000, 13.96446609406725692 ) ) ;
#23568=CARTESIAN_POINT ( 'NONE',  ( 69.40000000218495302, 9.999999999999998224, 17.49999999999999645 ) ) ;
#23579=CARTESIAN_POINT ( 'NONE',  ( 67.60000000109246798, 7.933012699999995476, 15.85617417291294196 ) ) ;
#23589=LINE ( 'NONE', #6717, #8242 ) ;
#23603=CARTESIAN_POINT ( 'NONE',  ( -67.89999999999999147, 7.499999999999996447, 14.99999999999999645 ) ) ;
#23608=CARTESIAN_POINT ( 'NONE',  ( -66.60000000109246798, 10.85617417291294551, 17.06698730000000097 ) ) ;
#23609=CARTESIAN_POINT ( 'NONE',  ( 68.25000000218493312, 11.03553390593269157, 12.49999999999994849 ) ) ;
#23611=CARTESIAN_POINT ( 'NONE',  ( -66.45000000218495018, 7.499999999999996447, 13.96446609406725514 ) ) ;
#23613=( GEOMETRIC_REPRESENTATION_CONTEXT ( 3 ) GLOBAL_UNCERTAINTY_ASSIGNED_CONTEXT ( ( #2352 ) ) GLOBAL_UNIT_ASSIGNED_CONTEXT ( ( #20701, #474, #15355 ) ) REPRESENTATION_CONTEXT ( 'NONE', 'WORKASPACE' ) );
#23614=CARTESIAN_POINT ( 'NONE',  ( -70.50000000109247367, 9.143825827087049163, 17.06698730000000097 ) ) ;
#23617=CARTESIAN_POINT ( 'NONE',  ( -65.90000000109246514, 7.933012699999995476, 14.14382582708705094 ) ) ;
#23626=CARTESIAN_POINT ( 'NONE',  ( -72.00000000109248788, 10.85617417291294551, 17.06698729999999742 ) ) ;
#23629=CARTESIAN_POINT ( 'NONE',  ( -69.25000000109245946, 7.933012699999995476, 14.99999999999999645 ) ) ;
#23634=LINE ( 'NONE', #1591, #5263 ) ;
#23639=CARTESIAN_POINT ( 'NONE',  ( -68.24999999999998579, 12.50000000000000000, 13.96446609406725692 ) ) ;
#23655=VECTOR ( 'NONE', #17767, 1000.000000000000000 ) ;
#23659=CARTESIAN_POINT ( 'NONE',  ( 70.25000000000000000, 7.499999999999995559, 16.03553390593273420 ) ) ;
#23662=CARTESIAN_POINT ( 'NONE',  ( 69.64999999999997726, 8.964466094067285340, 12.49999999999996980 ) ) ;
#23666=( BOUNDED_CURVE ( )  B_SPLINE_CURVE ( 2, ( #17842, #17732, #23348, #1296, #21651, #2979, #19743, #21285, #1411 ),
 .UNSPECIFIED., .F., .F. ) 
 B_SPLINE_CURVE_WITH_KNOTS ( ( 3, 2, 2, 2, 3 ),
 ( 0.8749999999999990008, 0.8906249999999994449, 0.9062499999999998890, 0.9218750000000003331, 0.9375000000000007772 ),
 .UNSPECIFIED. ) 
 CURVE ( )  GEOMETRIC_REPRESENTATION_ITEM ( )  RATIONAL_B_SPLINE_CURVE ( ( 1.000000000000004885, 0.9238795325112818535, 1.000000000000000000, 0.9238795325112867385, 1.000000000000000000, 0.9238795325112867385, 1.000000000000000000, 0.9238795325112829637, 1.000000000000003775 ) ) 
 REPRESENTATION_ITEM ( '' )  );
#23677=ORIENTED_EDGE ( 'NONE', *, *, #20068, .T. ) ;
#23686=CARTESIAN_POINT ( 'NONE',  ( 68.55000000218495870, 11.03553390593273598, 17.50000000000000355 ) ) ;
#23689=CARTESIAN_POINT ( 'NONE',  ( -68.84999999999998010, 8.964466094067214286, 12.50000000000004086 ) ) ;
ENDSEC;
END-ISO-10303-21;
